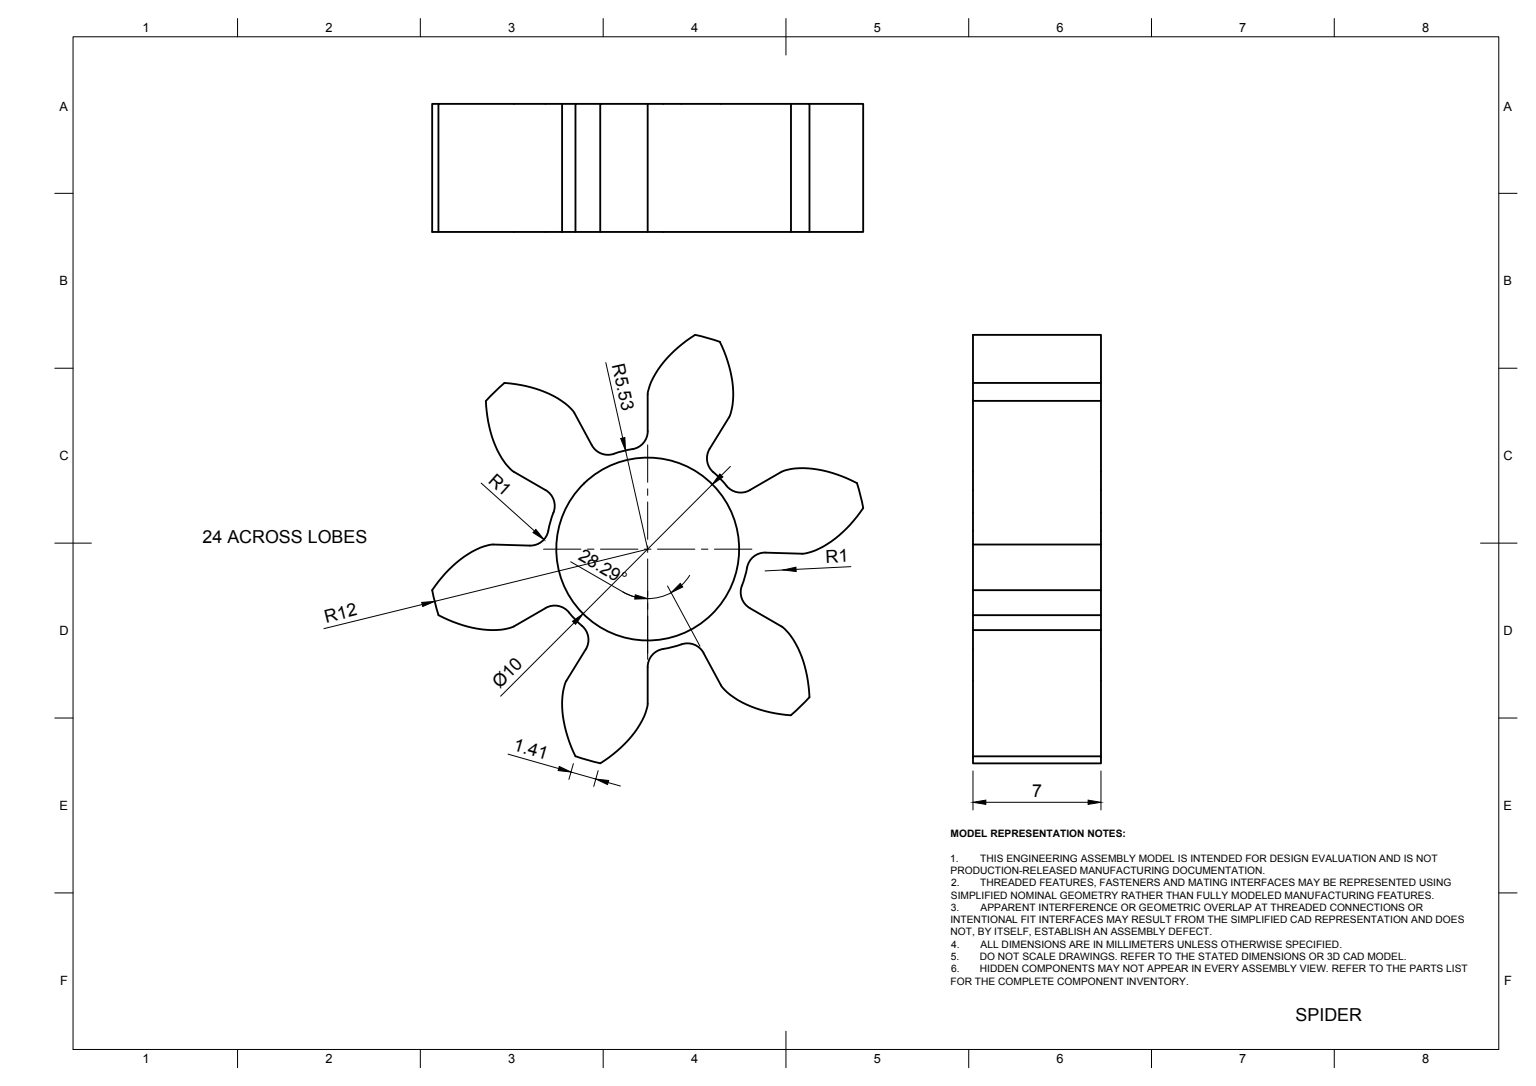
ISO-10303-21;
HEADER;
/* Generated by software containing ST-Developer
 * from STEP Tools, Inc. (www.steptools.com) 
 */

FILE_DESCRIPTION(
/* description */ (''),
/* implementation_level */ '2;1');

FILE_NAME(
/* name */ 'Spider.step',
/* time_stamp */ '2026-10-05T21:34:53-07:00',
/* author */ (''),
/* organization */ (''),
/* preprocessor_version */ 'ST-DEVELOPER v20.2',
/* originating_system */ 'Autodesk Translation Framework v15.15.0.0',
/* authorisation */ '');

FILE_SCHEMA (('AUTOMOTIVE_DESIGN { 1 0 10303 214 3 1 1 }'));
ENDSEC;

DATA;
#10=MECHANICAL_DESIGN_GEOMETRIC_PRESENTATION_REPRESENTATION('',(#65),#9822);
#47=SHAPE_REPRESENTATION_RELATIONSHIP('SRR','None',#9857,#56);
#56=ADVANCED_BREP_SHAPE_REPRESENTATION('',(#74),#9813);
#65=STYLED_ITEM('',(#9911),#74);
#74=MANIFOLD_SOLID_BREP('Body1',#3288);
#83=FACE_BOUND('',#486,.T.);
#84=FACE_BOUND('',#500,.T.);
#99=B_SPLINE_CURVE_WITH_KNOTS('',5,(#4949,#4950,#4951,#4952,#4953,#4954,
#4955,#4956,#4957,#4958,#4959,#4960,#4961,#4962,#4963,#4964,#4965,#4966,
#4967,#4968,#4969,#4970,#4971,#4972,#4973,#4974,#4975,#4976,#4977,#4978,
#4979,#4980,#4981,#4982,#4983,#4984,#4985,#4986,#4987,#4988,#4989,#4990,
#4991,#4992,#4993,#4994,#4995,#4996,#4997,#4998,#4999,#5000,#5001,#5002,
#5003,#5004,#5005,#5006,#5007,#5008,#5009,#5010,#5011,#5012,#5013,#5014,
#5015,#5016,#5017,#5018,#5019,#5020,#5021,#5022,#5023),.UNSPECIFIED.,.F.,
 .F.,(6,1,1,1,1,1,1,1,1,1,1,1,1,1,1,1,1,1,1,1,1,1,1,1,1,1,1,1,1,1,1,1,1,
1,1,1,1,1,1,1,1,1,1,1,1,1,1,1,1,1,1,1,1,1,1,1,1,1,1,1,1,1,1,1,1,1,1,1,1,
1,6),(-1.,-0.985714285714284,-0.97142857142857,-0.957142857142856,-0.942857142857141,
-0.928571428571427,-0.914285714285713,-0.899999999999999,-0.885714285714284,
-0.87142857142857,-0.857142857142856,-0.842857142857142,-0.828571428571428,
-0.814285714285713,-0.799999999999999,-0.785714285714285,-0.771428571428571,
-0.757142857142856,-0.742857142857142,-0.728571428571428,-0.714285714285714,
-0.699999999999999,-0.685714285714285,-0.671428571428571,-0.657142857142857,
-0.642857142857142,-0.628571428571428,-0.614285714285714,-0.6,-0.585714285714286,
-0.571428571428571,-0.557142857142857,-0.542857142857143,-0.528571428571429,
-0.514285714285714,-0.5,-0.485714285714286,-0.471428571428572,-0.457142857142857,
-0.442857142857143,-0.428571428571429,-0.414285714285714,-0.4,-0.385714285714286,
-0.371428571428571,-0.357142857142857,-0.342857142857143,-0.328571428571429,
-0.314285714285714,-0.3,-0.285714285714286,-0.271428571428571,-0.257142857142857,
-0.242857142857143,-0.228571428571429,-0.214285714285714,-0.2,-0.185714285714286,
-0.171428571428571,-0.157142857142857,-0.142857142857143,-0.128571428571429,
-0.114285714285714,-0.1,-0.0857142857142857,-0.0714285714285714,-0.0571428571428571,
-0.0428571428571429,-0.0285714285714286,-0.0142857142857143,0.),
 .UNSPECIFIED.);
#100=B_SPLINE_CURVE_WITH_KNOTS('',5,(#5025,#5026,#5027,#5028,#5029,#5030,
#5031,#5032,#5033,#5034,#5035,#5036,#5037,#5038,#5039,#5040,#5041,#5042,
#5043,#5044,#5045,#5046,#5047,#5048,#5049,#5050,#5051,#5052,#5053,#5054,
#5055,#5056,#5057,#5058,#5059,#5060,#5061,#5062,#5063,#5064,#5065,#5066,
#5067,#5068,#5069,#5070,#5071,#5072,#5073,#5074,#5075,#5076,#5077,#5078,
#5079,#5080,#5081,#5082,#5083,#5084,#5085,#5086,#5087,#5088,#5089,#5090,
#5091,#5092,#5093,#5094,#5095,#5096,#5097,#5098,#5099),.UNSPECIFIED.,.F.,
 .F.,(6,1,1,1,1,1,1,1,1,1,1,1,1,1,1,1,1,1,1,1,1,1,1,1,1,1,1,1,1,1,1,1,1,
1,1,1,1,1,1,1,1,1,1,1,1,1,1,1,1,1,1,1,1,1,1,1,1,1,1,1,1,1,1,1,1,1,1,1,1,
1,6),(-1.,-0.985714285714284,-0.97142857142857,-0.957142857142856,-0.942857142857141,
-0.928571428571427,-0.914285714285713,-0.899999999999999,-0.885714285714284,
-0.87142857142857,-0.857142857142856,-0.842857142857142,-0.828571428571428,
-0.814285714285713,-0.799999999999999,-0.785714285714285,-0.771428571428571,
-0.757142857142856,-0.742857142857142,-0.728571428571428,-0.714285714285714,
-0.699999999999999,-0.685714285714285,-0.671428571428571,-0.657142857142857,
-0.642857142857142,-0.628571428571428,-0.614285714285714,-0.6,-0.585714285714286,
-0.571428571428571,-0.557142857142857,-0.542857142857143,-0.528571428571429,
-0.514285714285714,-0.5,-0.485714285714286,-0.471428571428572,-0.457142857142857,
-0.442857142857143,-0.428571428571429,-0.414285714285714,-0.4,-0.385714285714286,
-0.371428571428571,-0.357142857142857,-0.342857142857143,-0.328571428571429,
-0.314285714285714,-0.3,-0.285714285714286,-0.271428571428571,-0.257142857142857,
-0.242857142857143,-0.228571428571429,-0.214285714285714,-0.2,-0.185714285714286,
-0.171428571428571,-0.157142857142857,-0.142857142857143,-0.128571428571429,
-0.114285714285714,-0.1,-0.0857142857142857,-0.0714285714285714,-0.0571428571428571,
-0.0428571428571429,-0.0285714285714286,-0.0142857142857143,0.),
 .UNSPECIFIED.);
#101=B_SPLINE_CURVE_WITH_KNOTS('',5,(#5257,#5258,#5259,#5260,#5261,#5262,
#5263,#5264,#5265,#5266,#5267,#5268,#5269,#5270,#5271,#5272,#5273,#5274,
#5275,#5276,#5277,#5278,#5279,#5280,#5281,#5282,#5283,#5284,#5285,#5286,
#5287,#5288,#5289,#5290,#5291,#5292,#5293,#5294,#5295,#5296,#5297,#5298,
#5299,#5300,#5301,#5302,#5303,#5304,#5305,#5306,#5307,#5308,#5309,#5310,
#5311,#5312,#5313,#5314,#5315,#5316,#5317,#5318,#5319,#5320,#5321,#5322,
#5323,#5324,#5325,#5326,#5327,#5328,#5329,#5330,#5331),.UNSPECIFIED.,.F.,
 .F.,(6,1,1,1,1,1,1,1,1,1,1,1,1,1,1,1,1,1,1,1,1,1,1,1,1,1,1,1,1,1,1,1,1,
1,1,1,1,1,1,1,1,1,1,1,1,1,1,1,1,1,1,1,1,1,1,1,1,1,1,1,1,1,1,1,1,1,1,1,1,
1,6),(0.,0.0142857142857143,0.0285714285714286,0.0428571428571429,0.0571428571428571,
0.0714285714285714,0.0857142857142857,0.1,0.114285714285714,0.128571428571429,
0.142857142857143,0.157142857142857,0.171428571428571,0.185714285714286,
0.2,0.214285714285714,0.228571428571429,0.242857142857143,0.257142857142857,
0.271428571428571,0.285714285714286,0.3,0.314285714285714,0.328571428571429,
0.342857142857143,0.357142857142857,0.371428571428571,0.385714285714286,
0.4,0.414285714285714,0.428571428571429,0.442857142857143,0.457142857142857,
0.471428571428572,0.485714285714286,0.5,0.514285714285714,0.528571428571429,
0.542857142857143,0.557142857142857,0.571428571428571,0.585714285714286,
0.6,0.614285714285714,0.628571428571428,0.642857142857142,0.657142857142857,
0.671428571428571,0.685714285714285,0.699999999999999,0.714285714285714,
0.728571428571428,0.742857142857142,0.757142857142856,0.771428571428571,
0.785714285714285,0.799999999999999,0.814285714285713,0.828571428571428,
0.842857142857142,0.857142857142856,0.87142857142857,0.885714285714284,
0.899999999999999,0.914285714285713,0.928571428571427,0.942857142857141,
0.957142857142856,0.97142857142857,0.985714285714284,1.),.UNSPECIFIED.);
#102=B_SPLINE_CURVE_WITH_KNOTS('',5,(#5332,#5333,#5334,#5335,#5336,#5337,
#5338,#5339,#5340,#5341,#5342,#5343,#5344,#5345,#5346,#5347,#5348,#5349,
#5350,#5351,#5352,#5353,#5354,#5355,#5356,#5357,#5358,#5359,#5360,#5361,
#5362,#5363,#5364,#5365,#5366,#5367,#5368,#5369,#5370,#5371,#5372,#5373,
#5374,#5375,#5376,#5377,#5378,#5379,#5380,#5381,#5382,#5383,#5384,#5385,
#5386,#5387,#5388,#5389,#5390,#5391,#5392,#5393,#5394,#5395,#5396,#5397,
#5398,#5399,#5400,#5401,#5402,#5403,#5404,#5405,#5406),.UNSPECIFIED.,.F.,
 .F.,(6,1,1,1,1,1,1,1,1,1,1,1,1,1,1,1,1,1,1,1,1,1,1,1,1,1,1,1,1,1,1,1,1,
1,1,1,1,1,1,1,1,1,1,1,1,1,1,1,1,1,1,1,1,1,1,1,1,1,1,1,1,1,1,1,1,1,1,1,1,
1,6),(0.,0.0142857142857143,0.0285714285714286,0.0428571428571429,0.0571428571428571,
0.0714285714285714,0.0857142857142857,0.1,0.114285714285714,0.128571428571429,
0.142857142857143,0.157142857142857,0.171428571428571,0.185714285714286,
0.2,0.214285714285714,0.228571428571429,0.242857142857143,0.257142857142857,
0.271428571428571,0.285714285714286,0.3,0.314285714285714,0.328571428571429,
0.342857142857143,0.357142857142857,0.371428571428571,0.385714285714286,
0.4,0.414285714285714,0.428571428571429,0.442857142857143,0.457142857142857,
0.471428571428572,0.485714285714286,0.5,0.514285714285714,0.528571428571429,
0.542857142857143,0.557142857142857,0.571428571428571,0.585714285714286,
0.6,0.614285714285714,0.628571428571428,0.642857142857142,0.657142857142857,
0.671428571428571,0.685714285714285,0.699999999999999,0.714285714285714,
0.728571428571428,0.742857142857142,0.757142857142856,0.771428571428571,
0.785714285714285,0.799999999999999,0.814285714285713,0.828571428571428,
0.842857142857142,0.857142857142856,0.87142857142857,0.885714285714284,
0.899999999999999,0.914285714285713,0.928571428571427,0.942857142857141,
0.957142857142856,0.97142857142857,0.985714285714284,1.),.UNSPECIFIED.);
#103=B_SPLINE_CURVE_WITH_KNOTS('',5,(#5558,#5559,#5560,#5561,#5562,#5563,
#5564,#5565,#5566,#5567,#5568,#5569,#5570,#5571,#5572,#5573,#5574,#5575,
#5576,#5577,#5578,#5579,#5580,#5581,#5582,#5583,#5584,#5585,#5586,#5587,
#5588,#5589,#5590,#5591,#5592,#5593,#5594,#5595,#5596,#5597,#5598,#5599,
#5600,#5601,#5602,#5603,#5604,#5605,#5606,#5607,#5608,#5609,#5610,#5611,
#5612,#5613,#5614,#5615,#5616,#5617,#5618,#5619,#5620,#5621,#5622,#5623,
#5624,#5625,#5626,#5627,#5628,#5629,#5630,#5631,#5632),.UNSPECIFIED.,.F.,
 .F.,(6,1,1,1,1,1,1,1,1,1,1,1,1,1,1,1,1,1,1,1,1,1,1,1,1,1,1,1,1,1,1,1,1,
1,1,1,1,1,1,1,1,1,1,1,1,1,1,1,1,1,1,1,1,1,1,1,1,1,1,1,1,1,1,1,1,1,1,1,1,
1,6),(-1.,-0.985714285714284,-0.97142857142857,-0.957142857142856,-0.942857142857141,
-0.928571428571427,-0.914285714285713,-0.899999999999999,-0.885714285714284,
-0.87142857142857,-0.857142857142856,-0.842857142857142,-0.828571428571428,
-0.814285714285713,-0.799999999999999,-0.785714285714285,-0.771428571428571,
-0.757142857142856,-0.742857142857142,-0.728571428571428,-0.714285714285714,
-0.699999999999999,-0.685714285714285,-0.671428571428571,-0.657142857142857,
-0.642857142857142,-0.628571428571428,-0.614285714285714,-0.6,-0.585714285714286,
-0.571428571428571,-0.557142857142857,-0.542857142857143,-0.528571428571429,
-0.514285714285714,-0.5,-0.485714285714286,-0.471428571428572,-0.457142857142857,
-0.442857142857143,-0.428571428571429,-0.414285714285714,-0.4,-0.385714285714286,
-0.371428571428571,-0.357142857142857,-0.342857142857143,-0.328571428571429,
-0.314285714285714,-0.3,-0.285714285714286,-0.271428571428571,-0.257142857142857,
-0.242857142857143,-0.228571428571429,-0.214285714285714,-0.2,-0.185714285714286,
-0.171428571428571,-0.157142857142857,-0.142857142857143,-0.128571428571429,
-0.114285714285714,-0.1,-0.0857142857142857,-0.0714285714285714,-0.0571428571428571,
-0.0428571428571429,-0.0285714285714286,-0.0142857142857143,0.),
 .UNSPECIFIED.);
#104=B_SPLINE_CURVE_WITH_KNOTS('',5,(#5634,#5635,#5636,#5637,#5638,#5639,
#5640,#5641,#5642,#5643,#5644,#5645,#5646,#5647,#5648,#5649,#5650,#5651,
#5652,#5653,#5654,#5655,#5656,#5657,#5658,#5659,#5660,#5661,#5662,#5663,
#5664,#5665,#5666,#5667,#5668,#5669,#5670,#5671,#5672,#5673,#5674,#5675,
#5676,#5677,#5678,#5679,#5680,#5681,#5682,#5683,#5684,#5685,#5686,#5687,
#5688,#5689,#5690,#5691,#5692,#5693,#5694,#5695,#5696,#5697,#5698,#5699,
#5700,#5701,#5702,#5703,#5704,#5705,#5706,#5707,#5708),.UNSPECIFIED.,.F.,
 .F.,(6,1,1,1,1,1,1,1,1,1,1,1,1,1,1,1,1,1,1,1,1,1,1,1,1,1,1,1,1,1,1,1,1,
1,1,1,1,1,1,1,1,1,1,1,1,1,1,1,1,1,1,1,1,1,1,1,1,1,1,1,1,1,1,1,1,1,1,1,1,
1,6),(-1.,-0.985714285714284,-0.97142857142857,-0.957142857142856,-0.942857142857141,
-0.928571428571427,-0.914285714285713,-0.899999999999999,-0.885714285714284,
-0.87142857142857,-0.857142857142856,-0.842857142857142,-0.828571428571428,
-0.814285714285713,-0.799999999999999,-0.785714285714285,-0.771428571428571,
-0.757142857142856,-0.742857142857142,-0.728571428571428,-0.714285714285714,
-0.699999999999999,-0.685714285714285,-0.671428571428571,-0.657142857142857,
-0.642857142857142,-0.628571428571428,-0.614285714285714,-0.6,-0.585714285714286,
-0.571428571428571,-0.557142857142857,-0.542857142857143,-0.528571428571429,
-0.514285714285714,-0.5,-0.485714285714286,-0.471428571428572,-0.457142857142857,
-0.442857142857143,-0.428571428571429,-0.414285714285714,-0.4,-0.385714285714286,
-0.371428571428571,-0.357142857142857,-0.342857142857143,-0.328571428571429,
-0.314285714285714,-0.3,-0.285714285714286,-0.271428571428571,-0.257142857142857,
-0.242857142857143,-0.228571428571429,-0.214285714285714,-0.2,-0.185714285714286,
-0.171428571428571,-0.157142857142857,-0.142857142857143,-0.128571428571429,
-0.114285714285714,-0.1,-0.0857142857142857,-0.0714285714285714,-0.0571428571428571,
-0.0428571428571429,-0.0285714285714286,-0.0142857142857143,0.),
 .UNSPECIFIED.);
#105=B_SPLINE_CURVE_WITH_KNOTS('',5,(#5866,#5867,#5868,#5869,#5870,#5871,
#5872,#5873,#5874,#5875,#5876,#5877,#5878,#5879,#5880,#5881,#5882,#5883,
#5884,#5885,#5886,#5887,#5888,#5889,#5890,#5891,#5892,#5893,#5894,#5895,
#5896,#5897,#5898,#5899,#5900,#5901,#5902,#5903,#5904,#5905,#5906,#5907,
#5908,#5909,#5910,#5911,#5912,#5913,#5914,#5915,#5916,#5917,#5918,#5919,
#5920,#5921,#5922,#5923,#5924,#5925,#5926,#5927,#5928,#5929,#5930,#5931,
#5932,#5933,#5934,#5935,#5936,#5937,#5938,#5939,#5940),.UNSPECIFIED.,.F.,
 .F.,(6,1,1,1,1,1,1,1,1,1,1,1,1,1,1,1,1,1,1,1,1,1,1,1,1,1,1,1,1,1,1,1,1,
1,1,1,1,1,1,1,1,1,1,1,1,1,1,1,1,1,1,1,1,1,1,1,1,1,1,1,1,1,1,1,1,1,1,1,1,
1,6),(0.,0.0142857142857143,0.0285714285714286,0.0428571428571429,0.0571428571428571,
0.0714285714285714,0.0857142857142857,0.1,0.114285714285714,0.128571428571429,
0.142857142857143,0.157142857142857,0.171428571428571,0.185714285714286,
0.2,0.214285714285714,0.228571428571429,0.242857142857143,0.257142857142857,
0.271428571428571,0.285714285714286,0.3,0.314285714285714,0.328571428571429,
0.342857142857143,0.357142857142857,0.371428571428571,0.385714285714286,
0.4,0.414285714285714,0.428571428571429,0.442857142857143,0.457142857142857,
0.471428571428572,0.485714285714286,0.5,0.514285714285714,0.528571428571429,
0.542857142857143,0.557142857142857,0.571428571428571,0.585714285714286,
0.6,0.614285714285714,0.628571428571428,0.642857142857142,0.657142857142857,
0.671428571428571,0.685714285714285,0.699999999999999,0.714285714285714,
0.728571428571428,0.742857142857142,0.757142857142856,0.771428571428571,
0.785714285714285,0.799999999999999,0.814285714285713,0.828571428571428,
0.842857142857142,0.857142857142856,0.87142857142857,0.885714285714284,
0.899999999999999,0.914285714285713,0.928571428571427,0.942857142857141,
0.957142857142856,0.97142857142857,0.985714285714284,1.),.UNSPECIFIED.);
#106=B_SPLINE_CURVE_WITH_KNOTS('',5,(#5941,#5942,#5943,#5944,#5945,#5946,
#5947,#5948,#5949,#5950,#5951,#5952,#5953,#5954,#5955,#5956,#5957,#5958,
#5959,#5960,#5961,#5962,#5963,#5964,#5965,#5966,#5967,#5968,#5969,#5970,
#5971,#5972,#5973,#5974,#5975,#5976,#5977,#5978,#5979,#5980,#5981,#5982,
#5983,#5984,#5985,#5986,#5987,#5988,#5989,#5990,#5991,#5992,#5993,#5994,
#5995,#5996,#5997,#5998,#5999,#6000,#6001,#6002,#6003,#6004,#6005,#6006,
#6007,#6008,#6009,#6010,#6011,#6012,#6013,#6014,#6015),.UNSPECIFIED.,.F.,
 .F.,(6,1,1,1,1,1,1,1,1,1,1,1,1,1,1,1,1,1,1,1,1,1,1,1,1,1,1,1,1,1,1,1,1,
1,1,1,1,1,1,1,1,1,1,1,1,1,1,1,1,1,1,1,1,1,1,1,1,1,1,1,1,1,1,1,1,1,1,1,1,
1,6),(0.,0.0142857142857143,0.0285714285714286,0.0428571428571429,0.0571428571428571,
0.0714285714285714,0.0857142857142857,0.1,0.114285714285714,0.128571428571429,
0.142857142857143,0.157142857142857,0.171428571428571,0.185714285714286,
0.2,0.214285714285714,0.228571428571429,0.242857142857143,0.257142857142857,
0.271428571428571,0.285714285714286,0.3,0.314285714285714,0.328571428571429,
0.342857142857143,0.357142857142857,0.371428571428571,0.385714285714286,
0.4,0.414285714285714,0.428571428571429,0.442857142857143,0.457142857142857,
0.471428571428572,0.485714285714286,0.5,0.514285714285714,0.528571428571429,
0.542857142857143,0.557142857142857,0.571428571428571,0.585714285714286,
0.6,0.614285714285714,0.628571428571428,0.642857142857142,0.657142857142857,
0.671428571428571,0.685714285714285,0.699999999999999,0.714285714285714,
0.728571428571428,0.742857142857142,0.757142857142856,0.771428571428571,
0.785714285714285,0.799999999999999,0.814285714285713,0.828571428571428,
0.842857142857142,0.857142857142856,0.87142857142857,0.885714285714284,
0.899999999999999,0.914285714285713,0.928571428571427,0.942857142857141,
0.957142857142856,0.97142857142857,0.985714285714284,1.),.UNSPECIFIED.);
#107=B_SPLINE_CURVE_WITH_KNOTS('',5,(#6167,#6168,#6169,#6170,#6171,#6172,
#6173,#6174,#6175,#6176,#6177,#6178,#6179,#6180,#6181,#6182,#6183,#6184,
#6185,#6186,#6187,#6188,#6189,#6190,#6191,#6192,#6193,#6194,#6195,#6196,
#6197,#6198,#6199,#6200,#6201,#6202,#6203,#6204,#6205,#6206,#6207,#6208,
#6209,#6210,#6211,#6212,#6213,#6214,#6215,#6216,#6217,#6218,#6219,#6220,
#6221,#6222,#6223,#6224,#6225,#6226,#6227,#6228,#6229,#6230,#6231,#6232,
#6233,#6234,#6235,#6236,#6237,#6238,#6239,#6240,#6241),.UNSPECIFIED.,.F.,
 .F.,(6,1,1,1,1,1,1,1,1,1,1,1,1,1,1,1,1,1,1,1,1,1,1,1,1,1,1,1,1,1,1,1,1,
1,1,1,1,1,1,1,1,1,1,1,1,1,1,1,1,1,1,1,1,1,1,1,1,1,1,1,1,1,1,1,1,1,1,1,1,
1,6),(-1.,-0.985714285714284,-0.97142857142857,-0.957142857142856,-0.942857142857141,
-0.928571428571427,-0.914285714285713,-0.899999999999999,-0.885714285714284,
-0.87142857142857,-0.857142857142856,-0.842857142857142,-0.828571428571428,
-0.814285714285713,-0.799999999999999,-0.785714285714285,-0.771428571428571,
-0.757142857142856,-0.742857142857142,-0.728571428571428,-0.714285714285714,
-0.699999999999999,-0.685714285714285,-0.671428571428571,-0.657142857142857,
-0.642857142857142,-0.628571428571428,-0.614285714285714,-0.6,-0.585714285714286,
-0.571428571428571,-0.557142857142857,-0.542857142857143,-0.528571428571429,
-0.514285714285714,-0.5,-0.485714285714286,-0.471428571428572,-0.457142857142857,
-0.442857142857143,-0.428571428571429,-0.414285714285714,-0.4,-0.385714285714286,
-0.371428571428571,-0.357142857142857,-0.342857142857143,-0.328571428571429,
-0.314285714285714,-0.3,-0.285714285714286,-0.271428571428571,-0.257142857142857,
-0.242857142857143,-0.228571428571429,-0.214285714285714,-0.2,-0.185714285714286,
-0.171428571428571,-0.157142857142857,-0.142857142857143,-0.128571428571429,
-0.114285714285714,-0.1,-0.0857142857142857,-0.0714285714285714,-0.0571428571428571,
-0.0428571428571429,-0.0285714285714286,-0.0142857142857143,0.),
 .UNSPECIFIED.);
#108=B_SPLINE_CURVE_WITH_KNOTS('',5,(#6243,#6244,#6245,#6246,#6247,#6248,
#6249,#6250,#6251,#6252,#6253,#6254,#6255,#6256,#6257,#6258,#6259,#6260,
#6261,#6262,#6263,#6264,#6265,#6266,#6267,#6268,#6269,#6270,#6271,#6272,
#6273,#6274,#6275,#6276,#6277,#6278,#6279,#6280,#6281,#6282,#6283,#6284,
#6285,#6286,#6287,#6288,#6289,#6290,#6291,#6292,#6293,#6294,#6295,#6296,
#6297,#6298,#6299,#6300,#6301,#6302,#6303,#6304,#6305,#6306,#6307,#6308,
#6309,#6310,#6311,#6312,#6313,#6314,#6315,#6316,#6317),.UNSPECIFIED.,.F.,
 .F.,(6,1,1,1,1,1,1,1,1,1,1,1,1,1,1,1,1,1,1,1,1,1,1,1,1,1,1,1,1,1,1,1,1,
1,1,1,1,1,1,1,1,1,1,1,1,1,1,1,1,1,1,1,1,1,1,1,1,1,1,1,1,1,1,1,1,1,1,1,1,
1,6),(-1.,-0.985714285714284,-0.97142857142857,-0.957142857142856,-0.942857142857141,
-0.928571428571427,-0.914285714285713,-0.899999999999999,-0.885714285714284,
-0.87142857142857,-0.857142857142856,-0.842857142857142,-0.828571428571428,
-0.814285714285713,-0.799999999999999,-0.785714285714285,-0.771428571428571,
-0.757142857142856,-0.742857142857142,-0.728571428571428,-0.714285714285714,
-0.699999999999999,-0.685714285714285,-0.671428571428571,-0.657142857142857,
-0.642857142857142,-0.628571428571428,-0.614285714285714,-0.6,-0.585714285714286,
-0.571428571428571,-0.557142857142857,-0.542857142857143,-0.528571428571429,
-0.514285714285714,-0.5,-0.485714285714286,-0.471428571428572,-0.457142857142857,
-0.442857142857143,-0.428571428571429,-0.414285714285714,-0.4,-0.385714285714286,
-0.371428571428571,-0.357142857142857,-0.342857142857143,-0.328571428571429,
-0.314285714285714,-0.3,-0.285714285714286,-0.271428571428571,-0.257142857142857,
-0.242857142857143,-0.228571428571429,-0.214285714285714,-0.2,-0.185714285714286,
-0.171428571428571,-0.157142857142857,-0.142857142857143,-0.128571428571429,
-0.114285714285714,-0.1,-0.0857142857142857,-0.0714285714285714,-0.0571428571428571,
-0.0428571428571429,-0.0285714285714286,-0.0142857142857143,0.),
 .UNSPECIFIED.);
#109=B_SPLINE_CURVE_WITH_KNOTS('',5,(#6475,#6476,#6477,#6478,#6479,#6480,
#6481,#6482,#6483,#6484,#6485,#6486,#6487,#6488,#6489,#6490,#6491,#6492,
#6493,#6494,#6495,#6496,#6497,#6498,#6499,#6500,#6501,#6502,#6503,#6504,
#6505,#6506,#6507,#6508,#6509,#6510,#6511,#6512,#6513,#6514,#6515,#6516,
#6517,#6518,#6519,#6520,#6521,#6522,#6523,#6524,#6525,#6526,#6527,#6528,
#6529,#6530,#6531,#6532,#6533,#6534,#6535,#6536,#6537,#6538,#6539,#6540,
#6541,#6542,#6543,#6544,#6545,#6546,#6547,#6548,#6549),.UNSPECIFIED.,.F.,
 .F.,(6,1,1,1,1,1,1,1,1,1,1,1,1,1,1,1,1,1,1,1,1,1,1,1,1,1,1,1,1,1,1,1,1,
1,1,1,1,1,1,1,1,1,1,1,1,1,1,1,1,1,1,1,1,1,1,1,1,1,1,1,1,1,1,1,1,1,1,1,1,
1,6),(0.,0.0142857142857143,0.0285714285714286,0.0428571428571429,0.0571428571428571,
0.0714285714285714,0.0857142857142857,0.1,0.114285714285714,0.128571428571429,
0.142857142857143,0.157142857142857,0.171428571428571,0.185714285714286,
0.2,0.214285714285714,0.228571428571429,0.242857142857143,0.257142857142857,
0.271428571428571,0.285714285714286,0.3,0.314285714285714,0.328571428571429,
0.342857142857143,0.357142857142857,0.371428571428571,0.385714285714286,
0.4,0.414285714285714,0.428571428571429,0.442857142857143,0.457142857142857,
0.471428571428572,0.485714285714286,0.5,0.514285714285714,0.528571428571429,
0.542857142857143,0.557142857142857,0.571428571428571,0.585714285714286,
0.6,0.614285714285714,0.628571428571428,0.642857142857142,0.657142857142857,
0.671428571428571,0.685714285714285,0.699999999999999,0.714285714285714,
0.728571428571428,0.742857142857142,0.757142857142856,0.771428571428571,
0.785714285714285,0.799999999999999,0.814285714285713,0.828571428571428,
0.842857142857142,0.857142857142856,0.87142857142857,0.885714285714284,
0.899999999999999,0.914285714285713,0.928571428571427,0.942857142857141,
0.957142857142856,0.97142857142857,0.985714285714284,1.),.UNSPECIFIED.);
#110=B_SPLINE_CURVE_WITH_KNOTS('',5,(#6550,#6551,#6552,#6553,#6554,#6555,
#6556,#6557,#6558,#6559,#6560,#6561,#6562,#6563,#6564,#6565,#6566,#6567,
#6568,#6569,#6570,#6571,#6572,#6573,#6574,#6575,#6576,#6577,#6578,#6579,
#6580,#6581,#6582,#6583,#6584,#6585,#6586,#6587,#6588,#6589,#6590,#6591,
#6592,#6593,#6594,#6595,#6596,#6597,#6598,#6599,#6600,#6601,#6602,#6603,
#6604,#6605,#6606,#6607,#6608,#6609,#6610,#6611,#6612,#6613,#6614,#6615,
#6616,#6617,#6618,#6619,#6620,#6621,#6622,#6623,#6624),.UNSPECIFIED.,.F.,
 .F.,(6,1,1,1,1,1,1,1,1,1,1,1,1,1,1,1,1,1,1,1,1,1,1,1,1,1,1,1,1,1,1,1,1,
1,1,1,1,1,1,1,1,1,1,1,1,1,1,1,1,1,1,1,1,1,1,1,1,1,1,1,1,1,1,1,1,1,1,1,1,
1,6),(0.,0.0142857142857143,0.0285714285714286,0.0428571428571429,0.0571428571428571,
0.0714285714285714,0.0857142857142857,0.1,0.114285714285714,0.128571428571429,
0.142857142857143,0.157142857142857,0.171428571428571,0.185714285714286,
0.2,0.214285714285714,0.228571428571429,0.242857142857143,0.257142857142857,
0.271428571428571,0.285714285714286,0.3,0.314285714285714,0.328571428571429,
0.342857142857143,0.357142857142857,0.371428571428571,0.385714285714286,
0.4,0.414285714285714,0.428571428571429,0.442857142857143,0.457142857142857,
0.471428571428572,0.485714285714286,0.5,0.514285714285714,0.528571428571429,
0.542857142857143,0.557142857142857,0.571428571428571,0.585714285714286,
0.6,0.614285714285714,0.628571428571428,0.642857142857142,0.657142857142857,
0.671428571428571,0.685714285714285,0.699999999999999,0.714285714285714,
0.728571428571428,0.742857142857142,0.757142857142856,0.771428571428571,
0.785714285714285,0.799999999999999,0.814285714285713,0.828571428571428,
0.842857142857142,0.857142857142856,0.87142857142857,0.885714285714284,
0.899999999999999,0.914285714285713,0.928571428571427,0.942857142857141,
0.957142857142856,0.97142857142857,0.985714285714284,1.),.UNSPECIFIED.);
#111=B_SPLINE_CURVE_WITH_KNOTS('',5,(#6776,#6777,#6778,#6779,#6780,#6781,
#6782,#6783,#6784,#6785,#6786,#6787,#6788,#6789,#6790,#6791,#6792,#6793,
#6794,#6795,#6796,#6797,#6798,#6799,#6800,#6801,#6802,#6803,#6804,#6805,
#6806,#6807,#6808,#6809,#6810,#6811,#6812,#6813,#6814,#6815,#6816,#6817,
#6818,#6819,#6820,#6821,#6822,#6823,#6824,#6825,#6826,#6827,#6828,#6829,
#6830,#6831,#6832,#6833,#6834,#6835,#6836,#6837,#6838,#6839,#6840,#6841,
#6842,#6843,#6844,#6845,#6846,#6847,#6848,#6849,#6850),.UNSPECIFIED.,.F.,
 .F.,(6,1,1,1,1,1,1,1,1,1,1,1,1,1,1,1,1,1,1,1,1,1,1,1,1,1,1,1,1,1,1,1,1,
1,1,1,1,1,1,1,1,1,1,1,1,1,1,1,1,1,1,1,1,1,1,1,1,1,1,1,1,1,1,1,1,1,1,1,1,
1,6),(-1.,-0.985714285714284,-0.97142857142857,-0.957142857142856,-0.942857142857141,
-0.928571428571427,-0.914285714285713,-0.899999999999999,-0.885714285714284,
-0.87142857142857,-0.857142857142856,-0.842857142857142,-0.828571428571428,
-0.814285714285713,-0.799999999999999,-0.785714285714285,-0.771428571428571,
-0.757142857142856,-0.742857142857142,-0.728571428571428,-0.714285714285714,
-0.699999999999999,-0.685714285714285,-0.671428571428571,-0.657142857142857,
-0.642857142857142,-0.628571428571428,-0.614285714285714,-0.6,-0.585714285714286,
-0.571428571428571,-0.557142857142857,-0.542857142857143,-0.528571428571429,
-0.514285714285714,-0.5,-0.485714285714286,-0.471428571428572,-0.457142857142857,
-0.442857142857143,-0.428571428571429,-0.414285714285714,-0.4,-0.385714285714286,
-0.371428571428571,-0.357142857142857,-0.342857142857143,-0.328571428571429,
-0.314285714285714,-0.3,-0.285714285714286,-0.271428571428571,-0.257142857142857,
-0.242857142857143,-0.228571428571429,-0.214285714285714,-0.2,-0.185714285714286,
-0.171428571428571,-0.157142857142857,-0.142857142857143,-0.128571428571429,
-0.114285714285714,-0.1,-0.0857142857142857,-0.0714285714285714,-0.0571428571428571,
-0.0428571428571429,-0.0285714285714286,-0.0142857142857143,0.),
 .UNSPECIFIED.);
#112=B_SPLINE_CURVE_WITH_KNOTS('',5,(#6852,#6853,#6854,#6855,#6856,#6857,
#6858,#6859,#6860,#6861,#6862,#6863,#6864,#6865,#6866,#6867,#6868,#6869,
#6870,#6871,#6872,#6873,#6874,#6875,#6876,#6877,#6878,#6879,#6880,#6881,
#6882,#6883,#6884,#6885,#6886,#6887,#6888,#6889,#6890,#6891,#6892,#6893,
#6894,#6895,#6896,#6897,#6898,#6899,#6900,#6901,#6902,#6903,#6904,#6905,
#6906,#6907,#6908,#6909,#6910,#6911,#6912,#6913,#6914,#6915,#6916,#6917,
#6918,#6919,#6920,#6921,#6922,#6923,#6924,#6925,#6926),.UNSPECIFIED.,.F.,
 .F.,(6,1,1,1,1,1,1,1,1,1,1,1,1,1,1,1,1,1,1,1,1,1,1,1,1,1,1,1,1,1,1,1,1,
1,1,1,1,1,1,1,1,1,1,1,1,1,1,1,1,1,1,1,1,1,1,1,1,1,1,1,1,1,1,1,1,1,1,1,1,
1,6),(-1.,-0.985714285714284,-0.97142857142857,-0.957142857142856,-0.942857142857141,
-0.928571428571427,-0.914285714285713,-0.899999999999999,-0.885714285714284,
-0.87142857142857,-0.857142857142856,-0.842857142857142,-0.828571428571428,
-0.814285714285713,-0.799999999999999,-0.785714285714285,-0.771428571428571,
-0.757142857142856,-0.742857142857142,-0.728571428571428,-0.714285714285714,
-0.699999999999999,-0.685714285714285,-0.671428571428571,-0.657142857142857,
-0.642857142857142,-0.628571428571428,-0.614285714285714,-0.6,-0.585714285714286,
-0.571428571428571,-0.557142857142857,-0.542857142857143,-0.528571428571429,
-0.514285714285714,-0.5,-0.485714285714286,-0.471428571428572,-0.457142857142857,
-0.442857142857143,-0.428571428571429,-0.414285714285714,-0.4,-0.385714285714286,
-0.371428571428571,-0.357142857142857,-0.342857142857143,-0.328571428571429,
-0.314285714285714,-0.3,-0.285714285714286,-0.271428571428571,-0.257142857142857,
-0.242857142857143,-0.228571428571429,-0.214285714285714,-0.2,-0.185714285714286,
-0.171428571428571,-0.157142857142857,-0.142857142857143,-0.128571428571429,
-0.114285714285714,-0.1,-0.0857142857142857,-0.0714285714285714,-0.0571428571428571,
-0.0428571428571429,-0.0285714285714286,-0.0142857142857143,0.),
 .UNSPECIFIED.);
#113=B_SPLINE_CURVE_WITH_KNOTS('',5,(#7084,#7085,#7086,#7087,#7088,#7089,
#7090,#7091,#7092,#7093,#7094,#7095,#7096,#7097,#7098,#7099,#7100,#7101,
#7102,#7103,#7104,#7105,#7106,#7107,#7108,#7109,#7110,#7111,#7112,#7113,
#7114,#7115,#7116,#7117,#7118,#7119,#7120,#7121,#7122,#7123,#7124,#7125,
#7126,#7127,#7128,#7129,#7130,#7131,#7132,#7133,#7134,#7135,#7136,#7137,
#7138,#7139,#7140,#7141,#7142,#7143,#7144,#7145,#7146,#7147,#7148,#7149,
#7150,#7151,#7152,#7153,#7154,#7155,#7156,#7157,#7158),.UNSPECIFIED.,.F.,
 .F.,(6,1,1,1,1,1,1,1,1,1,1,1,1,1,1,1,1,1,1,1,1,1,1,1,1,1,1,1,1,1,1,1,1,
1,1,1,1,1,1,1,1,1,1,1,1,1,1,1,1,1,1,1,1,1,1,1,1,1,1,1,1,1,1,1,1,1,1,1,1,
1,6),(0.,0.0142857142857143,0.0285714285714286,0.0428571428571429,0.0571428571428571,
0.0714285714285714,0.0857142857142857,0.1,0.114285714285714,0.128571428571429,
0.142857142857143,0.157142857142857,0.171428571428571,0.185714285714286,
0.2,0.214285714285714,0.228571428571429,0.242857142857143,0.257142857142857,
0.271428571428571,0.285714285714286,0.3,0.314285714285714,0.328571428571429,
0.342857142857143,0.357142857142857,0.371428571428571,0.385714285714286,
0.4,0.414285714285714,0.428571428571429,0.442857142857143,0.457142857142857,
0.471428571428572,0.485714285714286,0.5,0.514285714285714,0.528571428571429,
0.542857142857143,0.557142857142857,0.571428571428571,0.585714285714286,
0.6,0.614285714285714,0.628571428571428,0.642857142857142,0.657142857142857,
0.671428571428571,0.685714285714285,0.699999999999999,0.714285714285714,
0.728571428571428,0.742857142857142,0.757142857142856,0.771428571428571,
0.785714285714285,0.799999999999999,0.814285714285713,0.828571428571428,
0.842857142857142,0.857142857142856,0.87142857142857,0.885714285714284,
0.899999999999999,0.914285714285713,0.928571428571427,0.942857142857141,
0.957142857142856,0.97142857142857,0.985714285714284,1.),.UNSPECIFIED.);
#114=B_SPLINE_CURVE_WITH_KNOTS('',5,(#7159,#7160,#7161,#7162,#7163,#7164,
#7165,#7166,#7167,#7168,#7169,#7170,#7171,#7172,#7173,#7174,#7175,#7176,
#7177,#7178,#7179,#7180,#7181,#7182,#7183,#7184,#7185,#7186,#7187,#7188,
#7189,#7190,#7191,#7192,#7193,#7194,#7195,#7196,#7197,#7198,#7199,#7200,
#7201,#7202,#7203,#7204,#7205,#7206,#7207,#7208,#7209,#7210,#7211,#7212,
#7213,#7214,#7215,#7216,#7217,#7218,#7219,#7220,#7221,#7222,#7223,#7224,
#7225,#7226,#7227,#7228,#7229,#7230,#7231,#7232,#7233),.UNSPECIFIED.,.F.,
 .F.,(6,1,1,1,1,1,1,1,1,1,1,1,1,1,1,1,1,1,1,1,1,1,1,1,1,1,1,1,1,1,1,1,1,
1,1,1,1,1,1,1,1,1,1,1,1,1,1,1,1,1,1,1,1,1,1,1,1,1,1,1,1,1,1,1,1,1,1,1,1,
1,6),(0.,0.0142857142857143,0.0285714285714286,0.0428571428571429,0.0571428571428571,
0.0714285714285714,0.0857142857142857,0.1,0.114285714285714,0.128571428571429,
0.142857142857143,0.157142857142857,0.171428571428571,0.185714285714286,
0.2,0.214285714285714,0.228571428571429,0.242857142857143,0.257142857142857,
0.271428571428571,0.285714285714286,0.3,0.314285714285714,0.328571428571429,
0.342857142857143,0.357142857142857,0.371428571428571,0.385714285714286,
0.4,0.414285714285714,0.428571428571429,0.442857142857143,0.457142857142857,
0.471428571428572,0.485714285714286,0.5,0.514285714285714,0.528571428571429,
0.542857142857143,0.557142857142857,0.571428571428571,0.585714285714286,
0.6,0.614285714285714,0.628571428571428,0.642857142857142,0.657142857142857,
0.671428571428571,0.685714285714285,0.699999999999999,0.714285714285714,
0.728571428571428,0.742857142857142,0.757142857142856,0.771428571428571,
0.785714285714285,0.799999999999999,0.814285714285713,0.828571428571428,
0.842857142857142,0.857142857142856,0.87142857142857,0.885714285714284,
0.899999999999999,0.914285714285713,0.928571428571427,0.942857142857141,
0.957142857142856,0.97142857142857,0.985714285714284,1.),.UNSPECIFIED.);
#115=B_SPLINE_CURVE_WITH_KNOTS('',5,(#7385,#7386,#7387,#7388,#7389,#7390,
#7391,#7392,#7393,#7394,#7395,#7396,#7397,#7398,#7399,#7400,#7401,#7402,
#7403,#7404,#7405,#7406,#7407,#7408,#7409,#7410,#7411,#7412,#7413,#7414,
#7415,#7416,#7417,#7418,#7419,#7420,#7421,#7422,#7423,#7424,#7425,#7426,
#7427,#7428,#7429,#7430,#7431,#7432,#7433,#7434,#7435,#7436,#7437,#7438,
#7439,#7440,#7441,#7442,#7443,#7444,#7445,#7446,#7447,#7448,#7449,#7450,
#7451,#7452,#7453,#7454,#7455,#7456,#7457,#7458,#7459),.UNSPECIFIED.,.F.,
 .F.,(6,1,1,1,1,1,1,1,1,1,1,1,1,1,1,1,1,1,1,1,1,1,1,1,1,1,1,1,1,1,1,1,1,
1,1,1,1,1,1,1,1,1,1,1,1,1,1,1,1,1,1,1,1,1,1,1,1,1,1,1,1,1,1,1,1,1,1,1,1,
1,6),(-1.,-0.985714285714284,-0.97142857142857,-0.957142857142856,-0.942857142857141,
-0.928571428571427,-0.914285714285713,-0.899999999999999,-0.885714285714284,
-0.87142857142857,-0.857142857142856,-0.842857142857142,-0.828571428571428,
-0.814285714285713,-0.799999999999999,-0.785714285714285,-0.771428571428571,
-0.757142857142856,-0.742857142857142,-0.728571428571428,-0.714285714285714,
-0.699999999999999,-0.685714285714285,-0.671428571428571,-0.657142857142857,
-0.642857142857142,-0.628571428571428,-0.614285714285714,-0.6,-0.585714285714286,
-0.571428571428571,-0.557142857142857,-0.542857142857143,-0.528571428571429,
-0.514285714285714,-0.5,-0.485714285714286,-0.471428571428572,-0.457142857142857,
-0.442857142857143,-0.428571428571429,-0.414285714285714,-0.4,-0.385714285714286,
-0.371428571428571,-0.357142857142857,-0.342857142857143,-0.328571428571429,
-0.314285714285714,-0.3,-0.285714285714286,-0.271428571428571,-0.257142857142857,
-0.242857142857143,-0.228571428571429,-0.214285714285714,-0.2,-0.185714285714286,
-0.171428571428571,-0.157142857142857,-0.142857142857143,-0.128571428571429,
-0.114285714285714,-0.1,-0.0857142857142857,-0.0714285714285714,-0.0571428571428571,
-0.0428571428571429,-0.0285714285714286,-0.0142857142857143,0.),
 .UNSPECIFIED.);
#116=B_SPLINE_CURVE_WITH_KNOTS('',5,(#7461,#7462,#7463,#7464,#7465,#7466,
#7467,#7468,#7469,#7470,#7471,#7472,#7473,#7474,#7475,#7476,#7477,#7478,
#7479,#7480,#7481,#7482,#7483,#7484,#7485,#7486,#7487,#7488,#7489,#7490,
#7491,#7492,#7493,#7494,#7495,#7496,#7497,#7498,#7499,#7500,#7501,#7502,
#7503,#7504,#7505,#7506,#7507,#7508,#7509,#7510,#7511,#7512,#7513,#7514,
#7515,#7516,#7517,#7518,#7519,#7520,#7521,#7522,#7523,#7524,#7525,#7526,
#7527,#7528,#7529,#7530,#7531,#7532,#7533,#7534,#7535),.UNSPECIFIED.,.F.,
 .F.,(6,1,1,1,1,1,1,1,1,1,1,1,1,1,1,1,1,1,1,1,1,1,1,1,1,1,1,1,1,1,1,1,1,
1,1,1,1,1,1,1,1,1,1,1,1,1,1,1,1,1,1,1,1,1,1,1,1,1,1,1,1,1,1,1,1,1,1,1,1,
1,6),(-1.,-0.985714285714284,-0.97142857142857,-0.957142857142856,-0.942857142857141,
-0.928571428571427,-0.914285714285713,-0.899999999999999,-0.885714285714284,
-0.87142857142857,-0.857142857142856,-0.842857142857142,-0.828571428571428,
-0.814285714285713,-0.799999999999999,-0.785714285714285,-0.771428571428571,
-0.757142857142856,-0.742857142857142,-0.728571428571428,-0.714285714285714,
-0.699999999999999,-0.685714285714285,-0.671428571428571,-0.657142857142857,
-0.642857142857142,-0.628571428571428,-0.614285714285714,-0.6,-0.585714285714286,
-0.571428571428571,-0.557142857142857,-0.542857142857143,-0.528571428571429,
-0.514285714285714,-0.5,-0.485714285714286,-0.471428571428572,-0.457142857142857,
-0.442857142857143,-0.428571428571429,-0.414285714285714,-0.4,-0.385714285714286,
-0.371428571428571,-0.357142857142857,-0.342857142857143,-0.328571428571429,
-0.314285714285714,-0.3,-0.285714285714286,-0.271428571428571,-0.257142857142857,
-0.242857142857143,-0.228571428571429,-0.214285714285714,-0.2,-0.185714285714286,
-0.171428571428571,-0.157142857142857,-0.142857142857143,-0.128571428571429,
-0.114285714285714,-0.1,-0.0857142857142857,-0.0714285714285714,-0.0571428571428571,
-0.0428571428571429,-0.0285714285714286,-0.0142857142857143,0.),
 .UNSPECIFIED.);
#117=B_SPLINE_CURVE_WITH_KNOTS('',5,(#7693,#7694,#7695,#7696,#7697,#7698,
#7699,#7700,#7701,#7702,#7703,#7704,#7705,#7706,#7707,#7708,#7709,#7710,
#7711,#7712,#7713,#7714,#7715,#7716,#7717,#7718,#7719,#7720,#7721,#7722,
#7723,#7724,#7725,#7726,#7727,#7728,#7729,#7730,#7731,#7732,#7733,#7734,
#7735,#7736,#7737,#7738,#7739,#7740,#7741,#7742,#7743,#7744,#7745,#7746,
#7747,#7748,#7749,#7750,#7751,#7752,#7753,#7754,#7755,#7756,#7757,#7758,
#7759,#7760,#7761,#7762,#7763,#7764,#7765,#7766,#7767),.UNSPECIFIED.,.F.,
 .F.,(6,1,1,1,1,1,1,1,1,1,1,1,1,1,1,1,1,1,1,1,1,1,1,1,1,1,1,1,1,1,1,1,1,
1,1,1,1,1,1,1,1,1,1,1,1,1,1,1,1,1,1,1,1,1,1,1,1,1,1,1,1,1,1,1,1,1,1,1,1,
1,6),(0.,0.0142857142857143,0.0285714285714286,0.0428571428571429,0.0571428571428571,
0.0714285714285714,0.0857142857142857,0.1,0.114285714285714,0.128571428571429,
0.142857142857143,0.157142857142857,0.171428571428571,0.185714285714286,
0.2,0.214285714285714,0.228571428571429,0.242857142857143,0.257142857142857,
0.271428571428571,0.285714285714286,0.3,0.314285714285714,0.328571428571429,
0.342857142857143,0.357142857142857,0.371428571428571,0.385714285714286,
0.4,0.414285714285714,0.428571428571429,0.442857142857143,0.457142857142857,
0.471428571428572,0.485714285714286,0.5,0.514285714285714,0.528571428571429,
0.542857142857143,0.557142857142857,0.571428571428571,0.585714285714286,
0.6,0.614285714285714,0.628571428571428,0.642857142857142,0.657142857142857,
0.671428571428571,0.685714285714285,0.699999999999999,0.714285714285714,
0.728571428571428,0.742857142857142,0.757142857142856,0.771428571428571,
0.785714285714285,0.799999999999999,0.814285714285713,0.828571428571428,
0.842857142857142,0.857142857142856,0.87142857142857,0.885714285714284,
0.899999999999999,0.914285714285713,0.928571428571427,0.942857142857141,
0.957142857142856,0.97142857142857,0.985714285714284,1.),.UNSPECIFIED.);
#118=B_SPLINE_CURVE_WITH_KNOTS('',5,(#7768,#7769,#7770,#7771,#7772,#7773,
#7774,#7775,#7776,#7777,#7778,#7779,#7780,#7781,#7782,#7783,#7784,#7785,
#7786,#7787,#7788,#7789,#7790,#7791,#7792,#7793,#7794,#7795,#7796,#7797,
#7798,#7799,#7800,#7801,#7802,#7803,#7804,#7805,#7806,#7807,#7808,#7809,
#7810,#7811,#7812,#7813,#7814,#7815,#7816,#7817,#7818,#7819,#7820,#7821,
#7822,#7823,#7824,#7825,#7826,#7827,#7828,#7829,#7830,#7831,#7832,#7833,
#7834,#7835,#7836,#7837,#7838,#7839,#7840,#7841,#7842),.UNSPECIFIED.,.F.,
 .F.,(6,1,1,1,1,1,1,1,1,1,1,1,1,1,1,1,1,1,1,1,1,1,1,1,1,1,1,1,1,1,1,1,1,
1,1,1,1,1,1,1,1,1,1,1,1,1,1,1,1,1,1,1,1,1,1,1,1,1,1,1,1,1,1,1,1,1,1,1,1,
1,6),(0.,0.0142857142857143,0.0285714285714286,0.0428571428571429,0.0571428571428571,
0.0714285714285714,0.0857142857142857,0.1,0.114285714285714,0.128571428571429,
0.142857142857143,0.157142857142857,0.171428571428571,0.185714285714286,
0.2,0.214285714285714,0.228571428571429,0.242857142857143,0.257142857142857,
0.271428571428571,0.285714285714286,0.3,0.314285714285714,0.328571428571429,
0.342857142857143,0.357142857142857,0.371428571428571,0.385714285714286,
0.4,0.414285714285714,0.428571428571429,0.442857142857143,0.457142857142857,
0.471428571428572,0.485714285714286,0.5,0.514285714285714,0.528571428571429,
0.542857142857143,0.557142857142857,0.571428571428571,0.585714285714286,
0.6,0.614285714285714,0.628571428571428,0.642857142857142,0.657142857142857,
0.671428571428571,0.685714285714285,0.699999999999999,0.714285714285714,
0.728571428571428,0.742857142857142,0.757142857142856,0.771428571428571,
0.785714285714285,0.799999999999999,0.814285714285713,0.828571428571428,
0.842857142857142,0.857142857142856,0.87142857142857,0.885714285714284,
0.899999999999999,0.914285714285713,0.928571428571427,0.942857142857141,
0.957142857142856,0.97142857142857,0.985714285714284,1.),.UNSPECIFIED.);
#119=B_SPLINE_CURVE_WITH_KNOTS('',5,(#7854,#7855,#7856,#7857,#7858,#7859,
#7860,#7861,#7862,#7863,#7864,#7865,#7866,#7867,#7868,#7869,#7870,#7871,
#7872,#7873,#7874,#7875,#7876,#7877,#7878,#7879,#7880,#7881,#7882,#7883,
#7884,#7885,#7886,#7887,#7888,#7889,#7890,#7891,#7892,#7893,#7894,#7895,
#7896,#7897,#7898,#7899,#7900,#7901,#7902,#7903,#7904,#7905,#7906,#7907,
#7908,#7909,#7910,#7911,#7912,#7913,#7914,#7915,#7916,#7917,#7918,#7919,
#7920,#7921,#7922,#7923,#7924,#7925,#7926,#7927,#7928),.UNSPECIFIED.,.F.,
 .F.,(6,1,1,1,1,1,1,1,1,1,1,1,1,1,1,1,1,1,1,1,1,1,1,1,1,1,1,1,1,1,1,1,1,
1,1,1,1,1,1,1,1,1,1,1,1,1,1,1,1,1,1,1,1,1,1,1,1,1,1,1,1,1,1,1,1,1,1,1,1,
1,6),(-1.,-0.985714285714284,-0.97142857142857,-0.957142857142856,-0.942857142857141,
-0.928571428571427,-0.914285714285713,-0.899999999999999,-0.885714285714284,
-0.87142857142857,-0.857142857142856,-0.842857142857142,-0.828571428571428,
-0.814285714285713,-0.799999999999999,-0.785714285714285,-0.771428571428571,
-0.757142857142856,-0.742857142857142,-0.728571428571428,-0.714285714285714,
-0.699999999999999,-0.685714285714285,-0.671428571428571,-0.657142857142857,
-0.642857142857142,-0.628571428571428,-0.614285714285714,-0.6,-0.585714285714286,
-0.571428571428571,-0.557142857142857,-0.542857142857143,-0.528571428571429,
-0.514285714285714,-0.5,-0.485714285714286,-0.471428571428572,-0.457142857142857,
-0.442857142857143,-0.428571428571429,-0.414285714285714,-0.4,-0.385714285714286,
-0.371428571428571,-0.357142857142857,-0.342857142857143,-0.328571428571429,
-0.314285714285714,-0.3,-0.285714285714286,-0.271428571428571,-0.257142857142857,
-0.242857142857143,-0.228571428571429,-0.214285714285714,-0.2,-0.185714285714286,
-0.171428571428571,-0.157142857142857,-0.142857142857143,-0.128571428571429,
-0.114285714285714,-0.1,-0.0857142857142857,-0.0714285714285714,-0.0571428571428571,
-0.0428571428571429,-0.0285714285714286,-0.0142857142857143,0.),
 .UNSPECIFIED.);
#120=B_SPLINE_CURVE_WITH_KNOTS('',5,(#7932,#7933,#7934,#7935,#7936,#7937,
#7938,#7939,#7940,#7941,#7942,#7943,#7944,#7945,#7946,#7947,#7948,#7949,
#7950,#7951,#7952,#7953,#7954,#7955,#7956,#7957,#7958,#7959,#7960,#7961,
#7962,#7963,#7964,#7965,#7966,#7967,#7968,#7969,#7970,#7971,#7972,#7973,
#7974,#7975,#7976,#7977,#7978,#7979,#7980,#7981,#7982,#7983,#7984,#7985,
#7986,#7987,#7988,#7989,#7990,#7991,#7992,#7993,#7994,#7995,#7996,#7997,
#7998,#7999,#8000,#8001,#8002,#8003,#8004,#8005,#8006),.UNSPECIFIED.,.F.,
 .F.,(6,1,1,1,1,1,1,1,1,1,1,1,1,1,1,1,1,1,1,1,1,1,1,1,1,1,1,1,1,1,1,1,1,
1,1,1,1,1,1,1,1,1,1,1,1,1,1,1,1,1,1,1,1,1,1,1,1,1,1,1,1,1,1,1,1,1,1,1,1,
1,6),(0.,0.0142857142857143,0.0285714285714286,0.0428571428571429,0.0571428571428571,
0.0714285714285714,0.0857142857142857,0.1,0.114285714285714,0.128571428571429,
0.142857142857143,0.157142857142857,0.171428571428571,0.185714285714286,
0.2,0.214285714285714,0.228571428571429,0.242857142857143,0.257142857142857,
0.271428571428571,0.285714285714286,0.3,0.314285714285714,0.328571428571429,
0.342857142857143,0.357142857142857,0.371428571428571,0.385714285714286,
0.4,0.414285714285714,0.428571428571429,0.442857142857143,0.457142857142857,
0.471428571428572,0.485714285714286,0.5,0.514285714285714,0.528571428571429,
0.542857142857143,0.557142857142857,0.571428571428571,0.585714285714286,
0.6,0.614285714285714,0.628571428571428,0.642857142857142,0.657142857142857,
0.671428571428571,0.685714285714285,0.699999999999999,0.714285714285714,
0.728571428571428,0.742857142857142,0.757142857142856,0.771428571428571,
0.785714285714285,0.799999999999999,0.814285714285713,0.828571428571428,
0.842857142857142,0.857142857142856,0.87142857142857,0.885714285714284,
0.899999999999999,0.914285714285713,0.928571428571427,0.942857142857141,
0.957142857142856,0.97142857142857,0.985714285714284,1.),.UNSPECIFIED.);
#121=B_SPLINE_CURVE_WITH_KNOTS('',5,(#8196,#8197,#8198,#8199,#8200,#8201,
#8202,#8203,#8204,#8205,#8206,#8207,#8208,#8209,#8210,#8211,#8212,#8213,
#8214,#8215,#8216,#8217,#8218,#8219,#8220,#8221,#8222,#8223,#8224,#8225,
#8226,#8227,#8228,#8229,#8230,#8231,#8232,#8233,#8234,#8235,#8236,#8237,
#8238,#8239,#8240,#8241,#8242,#8243,#8244,#8245,#8246,#8247,#8248,#8249,
#8250,#8251,#8252,#8253,#8254,#8255,#8256,#8257,#8258,#8259,#8260,#8261,
#8262,#8263,#8264,#8265,#8266,#8267,#8268,#8269,#8270),.UNSPECIFIED.,.F.,
 .F.,(6,1,1,1,1,1,1,1,1,1,1,1,1,1,1,1,1,1,1,1,1,1,1,1,1,1,1,1,1,1,1,1,1,
1,1,1,1,1,1,1,1,1,1,1,1,1,1,1,1,1,1,1,1,1,1,1,1,1,1,1,1,1,1,1,1,1,1,1,1,
1,6),(-1.,-0.985714285714284,-0.97142857142857,-0.957142857142856,-0.942857142857141,
-0.928571428571427,-0.914285714285713,-0.899999999999999,-0.885714285714284,
-0.87142857142857,-0.857142857142856,-0.842857142857142,-0.828571428571428,
-0.814285714285713,-0.799999999999999,-0.785714285714285,-0.771428571428571,
-0.757142857142856,-0.742857142857142,-0.728571428571428,-0.714285714285714,
-0.699999999999999,-0.685714285714285,-0.671428571428571,-0.657142857142857,
-0.642857142857142,-0.628571428571428,-0.614285714285714,-0.6,-0.585714285714286,
-0.571428571428571,-0.557142857142857,-0.542857142857143,-0.528571428571429,
-0.514285714285714,-0.5,-0.485714285714286,-0.471428571428572,-0.457142857142857,
-0.442857142857143,-0.428571428571429,-0.414285714285714,-0.4,-0.385714285714286,
-0.371428571428571,-0.357142857142857,-0.342857142857143,-0.328571428571429,
-0.314285714285714,-0.3,-0.285714285714286,-0.271428571428571,-0.257142857142857,
-0.242857142857143,-0.228571428571429,-0.214285714285714,-0.2,-0.185714285714286,
-0.171428571428571,-0.157142857142857,-0.142857142857143,-0.128571428571429,
-0.114285714285714,-0.1,-0.0857142857142857,-0.0714285714285714,-0.0571428571428571,
-0.0428571428571429,-0.0285714285714286,-0.0142857142857143,0.),
 .UNSPECIFIED.);
#122=B_SPLINE_CURVE_WITH_KNOTS('',5,(#8426,#8427,#8428,#8429,#8430,#8431,
#8432,#8433,#8434,#8435,#8436,#8437,#8438,#8439,#8440,#8441,#8442,#8443,
#8444,#8445,#8446,#8447,#8448,#8449,#8450,#8451,#8452,#8453,#8454,#8455,
#8456,#8457,#8458,#8459,#8460,#8461,#8462,#8463,#8464,#8465,#8466,#8467,
#8468,#8469,#8470,#8471,#8472,#8473,#8474,#8475,#8476,#8477,#8478,#8479,
#8480,#8481,#8482,#8483,#8484,#8485,#8486,#8487,#8488,#8489,#8490,#8491,
#8492,#8493,#8494,#8495,#8496,#8497,#8498,#8499,#8500),.UNSPECIFIED.,.F.,
 .F.,(6,1,1,1,1,1,1,1,1,1,1,1,1,1,1,1,1,1,1,1,1,1,1,1,1,1,1,1,1,1,1,1,1,
1,1,1,1,1,1,1,1,1,1,1,1,1,1,1,1,1,1,1,1,1,1,1,1,1,1,1,1,1,1,1,1,1,1,1,1,
1,6),(0.,0.0142857142857143,0.0285714285714286,0.0428571428571429,0.0571428571428571,
0.0714285714285714,0.0857142857142857,0.1,0.114285714285714,0.128571428571429,
0.142857142857143,0.157142857142857,0.171428571428571,0.185714285714286,
0.2,0.214285714285714,0.228571428571429,0.242857142857143,0.257142857142857,
0.271428571428571,0.285714285714286,0.3,0.314285714285714,0.328571428571429,
0.342857142857143,0.357142857142857,0.371428571428571,0.385714285714286,
0.4,0.414285714285714,0.428571428571429,0.442857142857143,0.457142857142857,
0.471428571428572,0.485714285714286,0.5,0.514285714285714,0.528571428571429,
0.542857142857143,0.557142857142857,0.571428571428571,0.585714285714286,
0.6,0.614285714285714,0.628571428571428,0.642857142857142,0.657142857142857,
0.671428571428571,0.685714285714285,0.699999999999999,0.714285714285714,
0.728571428571428,0.742857142857142,0.757142857142856,0.771428571428571,
0.785714285714285,0.799999999999999,0.814285714285713,0.828571428571428,
0.842857142857142,0.857142857142856,0.87142857142857,0.885714285714284,
0.899999999999999,0.914285714285713,0.928571428571427,0.942857142857141,
0.957142857142856,0.97142857142857,0.985714285714284,1.),.UNSPECIFIED.);
#157=B_SPLINE_SURFACE_WITH_KNOTS('',5,1,((#4798,#4799),(#4800,#4801),(#4802,
#4803),(#4804,#4805),(#4806,#4807),(#4808,#4809),(#4810,#4811),(#4812,#4813),
(#4814,#4815),(#4816,#4817),(#4818,#4819),(#4820,#4821),(#4822,#4823),(#4824,
#4825),(#4826,#4827),(#4828,#4829),(#4830,#4831),(#4832,#4833),(#4834,#4835),
(#4836,#4837),(#4838,#4839),(#4840,#4841),(#4842,#4843),(#4844,#4845),(#4846,
#4847),(#4848,#4849),(#4850,#4851),(#4852,#4853),(#4854,#4855),(#4856,#4857),
(#4858,#4859),(#4860,#4861),(#4862,#4863),(#4864,#4865),(#4866,#4867),(#4868,
#4869),(#4870,#4871),(#4872,#4873),(#4874,#4875),(#4876,#4877),(#4878,#4879),
(#4880,#4881),(#4882,#4883),(#4884,#4885),(#4886,#4887),(#4888,#4889),(#4890,
#4891),(#4892,#4893),(#4894,#4895),(#4896,#4897),(#4898,#4899),(#4900,#4901),
(#4902,#4903),(#4904,#4905),(#4906,#4907),(#4908,#4909),(#4910,#4911),(#4912,
#4913),(#4914,#4915),(#4916,#4917),(#4918,#4919),(#4920,#4921),(#4922,#4923),
(#4924,#4925),(#4926,#4927),(#4928,#4929),(#4930,#4931),(#4932,#4933),(#4934,
#4935),(#4936,#4937),(#4938,#4939),(#4940,#4941),(#4942,#4943),(#4944,#4945),
(#4946,#4947)),.UNSPECIFIED.,.F.,.F.,.F.,(6,1,1,1,1,1,1,1,1,1,1,1,1,1,1,
1,1,1,1,1,1,1,1,1,1,1,1,1,1,1,1,1,1,1,1,1,1,1,1,1,1,1,1,1,1,1,1,1,1,1,1,
1,1,1,1,1,1,1,1,1,1,1,1,1,1,1,1,1,1,1,6),(2,2),(-1.,-0.985714285714284,
-0.97142857142857,-0.957142857142856,-0.942857142857141,-0.928571428571427,
-0.914285714285713,-0.899999999999999,-0.885714285714284,-0.87142857142857,
-0.857142857142856,-0.842857142857142,-0.828571428571428,-0.814285714285713,
-0.799999999999999,-0.785714285714285,-0.771428571428571,-0.757142857142856,
-0.742857142857142,-0.728571428571428,-0.714285714285714,-0.699999999999999,
-0.685714285714285,-0.671428571428571,-0.657142857142857,-0.642857142857142,
-0.628571428571428,-0.614285714285714,-0.6,-0.585714285714286,-0.571428571428571,
-0.557142857142857,-0.542857142857143,-0.528571428571429,-0.514285714285714,
-0.5,-0.485714285714286,-0.471428571428572,-0.457142857142857,-0.442857142857143,
-0.428571428571429,-0.414285714285714,-0.4,-0.385714285714286,-0.371428571428571,
-0.357142857142857,-0.342857142857143,-0.328571428571429,-0.314285714285714,
-0.3,-0.285714285714286,-0.271428571428571,-0.257142857142857,-0.242857142857143,
-0.228571428571429,-0.214285714285714,-0.2,-0.185714285714286,-0.171428571428571,
-0.157142857142857,-0.142857142857143,-0.128571428571429,-0.114285714285714,
-0.1,-0.0857142857142857,-0.0714285714285714,-0.0571428571428571,-0.0428571428571429,
-0.0285714285714286,-0.0142857142857143,0.),(0.,1.65),.UNSPECIFIED.);
#158=B_SPLINE_SURFACE_WITH_KNOTS('',5,1,((#5107,#5108),(#5109,#5110),(#5111,
#5112),(#5113,#5114),(#5115,#5116),(#5117,#5118),(#5119,#5120),(#5121,#5122),
(#5123,#5124),(#5125,#5126),(#5127,#5128),(#5129,#5130),(#5131,#5132),(#5133,
#5134),(#5135,#5136),(#5137,#5138),(#5139,#5140),(#5141,#5142),(#5143,#5144),
(#5145,#5146),(#5147,#5148),(#5149,#5150),(#5151,#5152),(#5153,#5154),(#5155,
#5156),(#5157,#5158),(#5159,#5160),(#5161,#5162),(#5163,#5164),(#5165,#5166),
(#5167,#5168),(#5169,#5170),(#5171,#5172),(#5173,#5174),(#5175,#5176),(#5177,
#5178),(#5179,#5180),(#5181,#5182),(#5183,#5184),(#5185,#5186),(#5187,#5188),
(#5189,#5190),(#5191,#5192),(#5193,#5194),(#5195,#5196),(#5197,#5198),(#5199,
#5200),(#5201,#5202),(#5203,#5204),(#5205,#5206),(#5207,#5208),(#5209,#5210),
(#5211,#5212),(#5213,#5214),(#5215,#5216),(#5217,#5218),(#5219,#5220),(#5221,
#5222),(#5223,#5224),(#5225,#5226),(#5227,#5228),(#5229,#5230),(#5231,#5232),
(#5233,#5234),(#5235,#5236),(#5237,#5238),(#5239,#5240),(#5241,#5242),(#5243,
#5244),(#5245,#5246),(#5247,#5248),(#5249,#5250),(#5251,#5252),(#5253,#5254),
(#5255,#5256)),.UNSPECIFIED.,.F.,.F.,.F.,(6,1,1,1,1,1,1,1,1,1,1,1,1,1,1,
1,1,1,1,1,1,1,1,1,1,1,1,1,1,1,1,1,1,1,1,1,1,1,1,1,1,1,1,1,1,1,1,1,1,1,1,
1,1,1,1,1,1,1,1,1,1,1,1,1,1,1,1,1,1,1,6),(2,2),(0.,0.0142857142857143,0.0285714285714286,
0.0428571428571429,0.0571428571428571,0.0714285714285714,0.0857142857142857,
0.1,0.114285714285714,0.128571428571429,0.142857142857143,0.157142857142857,
0.171428571428571,0.185714285714286,0.2,0.214285714285714,0.228571428571429,
0.242857142857143,0.257142857142857,0.271428571428571,0.285714285714286,
0.3,0.314285714285714,0.328571428571429,0.342857142857143,0.357142857142857,
0.371428571428571,0.385714285714286,0.4,0.414285714285714,0.428571428571429,
0.442857142857143,0.457142857142857,0.471428571428572,0.485714285714286,
0.5,0.514285714285714,0.528571428571429,0.542857142857143,0.557142857142857,
0.571428571428571,0.585714285714286,0.6,0.614285714285714,0.628571428571428,
0.642857142857142,0.657142857142857,0.671428571428571,0.685714285714285,
0.699999999999999,0.714285714285714,0.728571428571428,0.742857142857142,
0.757142857142856,0.771428571428571,0.785714285714285,0.799999999999999,
0.814285714285713,0.828571428571428,0.842857142857142,0.857142857142856,
0.87142857142857,0.885714285714284,0.899999999999999,0.914285714285713,
0.928571428571427,0.942857142857141,0.957142857142856,0.97142857142857,
0.985714285714284,1.),(0.,1.65),.UNSPECIFIED.);
#159=B_SPLINE_SURFACE_WITH_KNOTS('',5,1,((#5407,#5408),(#5409,#5410),(#5411,
#5412),(#5413,#5414),(#5415,#5416),(#5417,#5418),(#5419,#5420),(#5421,#5422),
(#5423,#5424),(#5425,#5426),(#5427,#5428),(#5429,#5430),(#5431,#5432),(#5433,
#5434),(#5435,#5436),(#5437,#5438),(#5439,#5440),(#5441,#5442),(#5443,#5444),
(#5445,#5446),(#5447,#5448),(#5449,#5450),(#5451,#5452),(#5453,#5454),(#5455,
#5456),(#5457,#5458),(#5459,#5460),(#5461,#5462),(#5463,#5464),(#5465,#5466),
(#5467,#5468),(#5469,#5470),(#5471,#5472),(#5473,#5474),(#5475,#5476),(#5477,
#5478),(#5479,#5480),(#5481,#5482),(#5483,#5484),(#5485,#5486),(#5487,#5488),
(#5489,#5490),(#5491,#5492),(#5493,#5494),(#5495,#5496),(#5497,#5498),(#5499,
#5500),(#5501,#5502),(#5503,#5504),(#5505,#5506),(#5507,#5508),(#5509,#5510),
(#5511,#5512),(#5513,#5514),(#5515,#5516),(#5517,#5518),(#5519,#5520),(#5521,
#5522),(#5523,#5524),(#5525,#5526),(#5527,#5528),(#5529,#5530),(#5531,#5532),
(#5533,#5534),(#5535,#5536),(#5537,#5538),(#5539,#5540),(#5541,#5542),(#5543,
#5544),(#5545,#5546),(#5547,#5548),(#5549,#5550),(#5551,#5552),(#5553,#5554),
(#5555,#5556)),.UNSPECIFIED.,.F.,.F.,.F.,(6,1,1,1,1,1,1,1,1,1,1,1,1,1,1,
1,1,1,1,1,1,1,1,1,1,1,1,1,1,1,1,1,1,1,1,1,1,1,1,1,1,1,1,1,1,1,1,1,1,1,1,
1,1,1,1,1,1,1,1,1,1,1,1,1,1,1,1,1,1,1,6),(2,2),(-1.,-0.985714285714284,
-0.97142857142857,-0.957142857142856,-0.942857142857141,-0.928571428571427,
-0.914285714285713,-0.899999999999999,-0.885714285714284,-0.87142857142857,
-0.857142857142856,-0.842857142857142,-0.828571428571428,-0.814285714285713,
-0.799999999999999,-0.785714285714285,-0.771428571428571,-0.757142857142856,
-0.742857142857142,-0.728571428571428,-0.714285714285714,-0.699999999999999,
-0.685714285714285,-0.671428571428571,-0.657142857142857,-0.642857142857142,
-0.628571428571428,-0.614285714285714,-0.6,-0.585714285714286,-0.571428571428571,
-0.557142857142857,-0.542857142857143,-0.528571428571429,-0.514285714285714,
-0.5,-0.485714285714286,-0.471428571428572,-0.457142857142857,-0.442857142857143,
-0.428571428571429,-0.414285714285714,-0.4,-0.385714285714286,-0.371428571428571,
-0.357142857142857,-0.342857142857143,-0.328571428571429,-0.314285714285714,
-0.3,-0.285714285714286,-0.271428571428571,-0.257142857142857,-0.242857142857143,
-0.228571428571429,-0.214285714285714,-0.2,-0.185714285714286,-0.171428571428571,
-0.157142857142857,-0.142857142857143,-0.128571428571429,-0.114285714285714,
-0.1,-0.0857142857142857,-0.0714285714285714,-0.0571428571428571,-0.0428571428571429,
-0.0285714285714286,-0.0142857142857143,0.),(0.,1.65),.UNSPECIFIED.);
#160=B_SPLINE_SURFACE_WITH_KNOTS('',5,1,((#5716,#5717),(#5718,#5719),(#5720,
#5721),(#5722,#5723),(#5724,#5725),(#5726,#5727),(#5728,#5729),(#5730,#5731),
(#5732,#5733),(#5734,#5735),(#5736,#5737),(#5738,#5739),(#5740,#5741),(#5742,
#5743),(#5744,#5745),(#5746,#5747),(#5748,#5749),(#5750,#5751),(#5752,#5753),
(#5754,#5755),(#5756,#5757),(#5758,#5759),(#5760,#5761),(#5762,#5763),(#5764,
#5765),(#5766,#5767),(#5768,#5769),(#5770,#5771),(#5772,#5773),(#5774,#5775),
(#5776,#5777),(#5778,#5779),(#5780,#5781),(#5782,#5783),(#5784,#5785),(#5786,
#5787),(#5788,#5789),(#5790,#5791),(#5792,#5793),(#5794,#5795),(#5796,#5797),
(#5798,#5799),(#5800,#5801),(#5802,#5803),(#5804,#5805),(#5806,#5807),(#5808,
#5809),(#5810,#5811),(#5812,#5813),(#5814,#5815),(#5816,#5817),(#5818,#5819),
(#5820,#5821),(#5822,#5823),(#5824,#5825),(#5826,#5827),(#5828,#5829),(#5830,
#5831),(#5832,#5833),(#5834,#5835),(#5836,#5837),(#5838,#5839),(#5840,#5841),
(#5842,#5843),(#5844,#5845),(#5846,#5847),(#5848,#5849),(#5850,#5851),(#5852,
#5853),(#5854,#5855),(#5856,#5857),(#5858,#5859),(#5860,#5861),(#5862,#5863),
(#5864,#5865)),.UNSPECIFIED.,.F.,.F.,.F.,(6,1,1,1,1,1,1,1,1,1,1,1,1,1,1,
1,1,1,1,1,1,1,1,1,1,1,1,1,1,1,1,1,1,1,1,1,1,1,1,1,1,1,1,1,1,1,1,1,1,1,1,
1,1,1,1,1,1,1,1,1,1,1,1,1,1,1,1,1,1,1,6),(2,2),(0.,0.0142857142857143,0.0285714285714286,
0.0428571428571429,0.0571428571428571,0.0714285714285714,0.0857142857142857,
0.1,0.114285714285714,0.128571428571429,0.142857142857143,0.157142857142857,
0.171428571428571,0.185714285714286,0.2,0.214285714285714,0.228571428571429,
0.242857142857143,0.257142857142857,0.271428571428571,0.285714285714286,
0.3,0.314285714285714,0.328571428571429,0.342857142857143,0.357142857142857,
0.371428571428571,0.385714285714286,0.4,0.414285714285714,0.428571428571429,
0.442857142857143,0.457142857142857,0.471428571428572,0.485714285714286,
0.5,0.514285714285714,0.528571428571429,0.542857142857143,0.557142857142857,
0.571428571428571,0.585714285714286,0.6,0.614285714285714,0.628571428571428,
0.642857142857142,0.657142857142857,0.671428571428571,0.685714285714285,
0.699999999999999,0.714285714285714,0.728571428571428,0.742857142857142,
0.757142857142856,0.771428571428571,0.785714285714285,0.799999999999999,
0.814285714285713,0.828571428571428,0.842857142857142,0.857142857142856,
0.87142857142857,0.885714285714284,0.899999999999999,0.914285714285713,
0.928571428571427,0.942857142857141,0.957142857142856,0.97142857142857,
0.985714285714284,1.),(0.,1.65),.UNSPECIFIED.);
#161=B_SPLINE_SURFACE_WITH_KNOTS('',5,1,((#6016,#6017),(#6018,#6019),(#6020,
#6021),(#6022,#6023),(#6024,#6025),(#6026,#6027),(#6028,#6029),(#6030,#6031),
(#6032,#6033),(#6034,#6035),(#6036,#6037),(#6038,#6039),(#6040,#6041),(#6042,
#6043),(#6044,#6045),(#6046,#6047),(#6048,#6049),(#6050,#6051),(#6052,#6053),
(#6054,#6055),(#6056,#6057),(#6058,#6059),(#6060,#6061),(#6062,#6063),(#6064,
#6065),(#6066,#6067),(#6068,#6069),(#6070,#6071),(#6072,#6073),(#6074,#6075),
(#6076,#6077),(#6078,#6079),(#6080,#6081),(#6082,#6083),(#6084,#6085),(#6086,
#6087),(#6088,#6089),(#6090,#6091),(#6092,#6093),(#6094,#6095),(#6096,#6097),
(#6098,#6099),(#6100,#6101),(#6102,#6103),(#6104,#6105),(#6106,#6107),(#6108,
#6109),(#6110,#6111),(#6112,#6113),(#6114,#6115),(#6116,#6117),(#6118,#6119),
(#6120,#6121),(#6122,#6123),(#6124,#6125),(#6126,#6127),(#6128,#6129),(#6130,
#6131),(#6132,#6133),(#6134,#6135),(#6136,#6137),(#6138,#6139),(#6140,#6141),
(#6142,#6143),(#6144,#6145),(#6146,#6147),(#6148,#6149),(#6150,#6151),(#6152,
#6153),(#6154,#6155),(#6156,#6157),(#6158,#6159),(#6160,#6161),(#6162,#6163),
(#6164,#6165)),.UNSPECIFIED.,.F.,.F.,.F.,(6,1,1,1,1,1,1,1,1,1,1,1,1,1,1,
1,1,1,1,1,1,1,1,1,1,1,1,1,1,1,1,1,1,1,1,1,1,1,1,1,1,1,1,1,1,1,1,1,1,1,1,
1,1,1,1,1,1,1,1,1,1,1,1,1,1,1,1,1,1,1,6),(2,2),(-1.,-0.985714285714284,
-0.97142857142857,-0.957142857142856,-0.942857142857141,-0.928571428571427,
-0.914285714285713,-0.899999999999999,-0.885714285714284,-0.87142857142857,
-0.857142857142856,-0.842857142857142,-0.828571428571428,-0.814285714285713,
-0.799999999999999,-0.785714285714285,-0.771428571428571,-0.757142857142856,
-0.742857142857142,-0.728571428571428,-0.714285714285714,-0.699999999999999,
-0.685714285714285,-0.671428571428571,-0.657142857142857,-0.642857142857142,
-0.628571428571428,-0.614285714285714,-0.6,-0.585714285714286,-0.571428571428571,
-0.557142857142857,-0.542857142857143,-0.528571428571429,-0.514285714285714,
-0.5,-0.485714285714286,-0.471428571428572,-0.457142857142857,-0.442857142857143,
-0.428571428571429,-0.414285714285714,-0.4,-0.385714285714286,-0.371428571428571,
-0.357142857142857,-0.342857142857143,-0.328571428571429,-0.314285714285714,
-0.3,-0.285714285714286,-0.271428571428571,-0.257142857142857,-0.242857142857143,
-0.228571428571429,-0.214285714285714,-0.2,-0.185714285714286,-0.171428571428571,
-0.157142857142857,-0.142857142857143,-0.128571428571429,-0.114285714285714,
-0.1,-0.0857142857142857,-0.0714285714285714,-0.0571428571428571,-0.0428571428571429,
-0.0285714285714286,-0.0142857142857143,0.),(0.,1.65),.UNSPECIFIED.);
#162=B_SPLINE_SURFACE_WITH_KNOTS('',5,1,((#6325,#6326),(#6327,#6328),(#6329,
#6330),(#6331,#6332),(#6333,#6334),(#6335,#6336),(#6337,#6338),(#6339,#6340),
(#6341,#6342),(#6343,#6344),(#6345,#6346),(#6347,#6348),(#6349,#6350),(#6351,
#6352),(#6353,#6354),(#6355,#6356),(#6357,#6358),(#6359,#6360),(#6361,#6362),
(#6363,#6364),(#6365,#6366),(#6367,#6368),(#6369,#6370),(#6371,#6372),(#6373,
#6374),(#6375,#6376),(#6377,#6378),(#6379,#6380),(#6381,#6382),(#6383,#6384),
(#6385,#6386),(#6387,#6388),(#6389,#6390),(#6391,#6392),(#6393,#6394),(#6395,
#6396),(#6397,#6398),(#6399,#6400),(#6401,#6402),(#6403,#6404),(#6405,#6406),
(#6407,#6408),(#6409,#6410),(#6411,#6412),(#6413,#6414),(#6415,#6416),(#6417,
#6418),(#6419,#6420),(#6421,#6422),(#6423,#6424),(#6425,#6426),(#6427,#6428),
(#6429,#6430),(#6431,#6432),(#6433,#6434),(#6435,#6436),(#6437,#6438),(#6439,
#6440),(#6441,#6442),(#6443,#6444),(#6445,#6446),(#6447,#6448),(#6449,#6450),
(#6451,#6452),(#6453,#6454),(#6455,#6456),(#6457,#6458),(#6459,#6460),(#6461,
#6462),(#6463,#6464),(#6465,#6466),(#6467,#6468),(#6469,#6470),(#6471,#6472),
(#6473,#6474)),.UNSPECIFIED.,.F.,.F.,.F.,(6,1,1,1,1,1,1,1,1,1,1,1,1,1,1,
1,1,1,1,1,1,1,1,1,1,1,1,1,1,1,1,1,1,1,1,1,1,1,1,1,1,1,1,1,1,1,1,1,1,1,1,
1,1,1,1,1,1,1,1,1,1,1,1,1,1,1,1,1,1,1,6),(2,2),(0.,0.0142857142857143,0.0285714285714286,
0.0428571428571429,0.0571428571428571,0.0714285714285714,0.0857142857142857,
0.1,0.114285714285714,0.128571428571429,0.142857142857143,0.157142857142857,
0.171428571428571,0.185714285714286,0.2,0.214285714285714,0.228571428571429,
0.242857142857143,0.257142857142857,0.271428571428571,0.285714285714286,
0.3,0.314285714285714,0.328571428571429,0.342857142857143,0.357142857142857,
0.371428571428571,0.385714285714286,0.4,0.414285714285714,0.428571428571429,
0.442857142857143,0.457142857142857,0.471428571428572,0.485714285714286,
0.5,0.514285714285714,0.528571428571429,0.542857142857143,0.557142857142857,
0.571428571428571,0.585714285714286,0.6,0.614285714285714,0.628571428571428,
0.642857142857142,0.657142857142857,0.671428571428571,0.685714285714285,
0.699999999999999,0.714285714285714,0.728571428571428,0.742857142857142,
0.757142857142856,0.771428571428571,0.785714285714285,0.799999999999999,
0.814285714285713,0.828571428571428,0.842857142857142,0.857142857142856,
0.87142857142857,0.885714285714284,0.899999999999999,0.914285714285713,
0.928571428571427,0.942857142857141,0.957142857142856,0.97142857142857,
0.985714285714284,1.),(0.,1.65),.UNSPECIFIED.);
#163=B_SPLINE_SURFACE_WITH_KNOTS('',5,1,((#6625,#6626),(#6627,#6628),(#6629,
#6630),(#6631,#6632),(#6633,#6634),(#6635,#6636),(#6637,#6638),(#6639,#6640),
(#6641,#6642),(#6643,#6644),(#6645,#6646),(#6647,#6648),(#6649,#6650),(#6651,
#6652),(#6653,#6654),(#6655,#6656),(#6657,#6658),(#6659,#6660),(#6661,#6662),
(#6663,#6664),(#6665,#6666),(#6667,#6668),(#6669,#6670),(#6671,#6672),(#6673,
#6674),(#6675,#6676),(#6677,#6678),(#6679,#6680),(#6681,#6682),(#6683,#6684),
(#6685,#6686),(#6687,#6688),(#6689,#6690),(#6691,#6692),(#6693,#6694),(#6695,
#6696),(#6697,#6698),(#6699,#6700),(#6701,#6702),(#6703,#6704),(#6705,#6706),
(#6707,#6708),(#6709,#6710),(#6711,#6712),(#6713,#6714),(#6715,#6716),(#6717,
#6718),(#6719,#6720),(#6721,#6722),(#6723,#6724),(#6725,#6726),(#6727,#6728),
(#6729,#6730),(#6731,#6732),(#6733,#6734),(#6735,#6736),(#6737,#6738),(#6739,
#6740),(#6741,#6742),(#6743,#6744),(#6745,#6746),(#6747,#6748),(#6749,#6750),
(#6751,#6752),(#6753,#6754),(#6755,#6756),(#6757,#6758),(#6759,#6760),(#6761,
#6762),(#6763,#6764),(#6765,#6766),(#6767,#6768),(#6769,#6770),(#6771,#6772),
(#6773,#6774)),.UNSPECIFIED.,.F.,.F.,.F.,(6,1,1,1,1,1,1,1,1,1,1,1,1,1,1,
1,1,1,1,1,1,1,1,1,1,1,1,1,1,1,1,1,1,1,1,1,1,1,1,1,1,1,1,1,1,1,1,1,1,1,1,
1,1,1,1,1,1,1,1,1,1,1,1,1,1,1,1,1,1,1,6),(2,2),(-1.,-0.985714285714284,
-0.97142857142857,-0.957142857142856,-0.942857142857141,-0.928571428571427,
-0.914285714285713,-0.899999999999999,-0.885714285714284,-0.87142857142857,
-0.857142857142856,-0.842857142857142,-0.828571428571428,-0.814285714285713,
-0.799999999999999,-0.785714285714285,-0.771428571428571,-0.757142857142856,
-0.742857142857142,-0.728571428571428,-0.714285714285714,-0.699999999999999,
-0.685714285714285,-0.671428571428571,-0.657142857142857,-0.642857142857142,
-0.628571428571428,-0.614285714285714,-0.6,-0.585714285714286,-0.571428571428571,
-0.557142857142857,-0.542857142857143,-0.528571428571429,-0.514285714285714,
-0.5,-0.485714285714286,-0.471428571428572,-0.457142857142857,-0.442857142857143,
-0.428571428571429,-0.414285714285714,-0.4,-0.385714285714286,-0.371428571428571,
-0.357142857142857,-0.342857142857143,-0.328571428571429,-0.314285714285714,
-0.3,-0.285714285714286,-0.271428571428571,-0.257142857142857,-0.242857142857143,
-0.228571428571429,-0.214285714285714,-0.2,-0.185714285714286,-0.171428571428571,
-0.157142857142857,-0.142857142857143,-0.128571428571429,-0.114285714285714,
-0.1,-0.0857142857142857,-0.0714285714285714,-0.0571428571428571,-0.0428571428571429,
-0.0285714285714286,-0.0142857142857143,0.),(0.,1.65),.UNSPECIFIED.);
#164=B_SPLINE_SURFACE_WITH_KNOTS('',5,1,((#6934,#6935),(#6936,#6937),(#6938,
#6939),(#6940,#6941),(#6942,#6943),(#6944,#6945),(#6946,#6947),(#6948,#6949),
(#6950,#6951),(#6952,#6953),(#6954,#6955),(#6956,#6957),(#6958,#6959),(#6960,
#6961),(#6962,#6963),(#6964,#6965),(#6966,#6967),(#6968,#6969),(#6970,#6971),
(#6972,#6973),(#6974,#6975),(#6976,#6977),(#6978,#6979),(#6980,#6981),(#6982,
#6983),(#6984,#6985),(#6986,#6987),(#6988,#6989),(#6990,#6991),(#6992,#6993),
(#6994,#6995),(#6996,#6997),(#6998,#6999),(#7000,#7001),(#7002,#7003),(#7004,
#7005),(#7006,#7007),(#7008,#7009),(#7010,#7011),(#7012,#7013),(#7014,#7015),
(#7016,#7017),(#7018,#7019),(#7020,#7021),(#7022,#7023),(#7024,#7025),(#7026,
#7027),(#7028,#7029),(#7030,#7031),(#7032,#7033),(#7034,#7035),(#7036,#7037),
(#7038,#7039),(#7040,#7041),(#7042,#7043),(#7044,#7045),(#7046,#7047),(#7048,
#7049),(#7050,#7051),(#7052,#7053),(#7054,#7055),(#7056,#7057),(#7058,#7059),
(#7060,#7061),(#7062,#7063),(#7064,#7065),(#7066,#7067),(#7068,#7069),(#7070,
#7071),(#7072,#7073),(#7074,#7075),(#7076,#7077),(#7078,#7079),(#7080,#7081),
(#7082,#7083)),.UNSPECIFIED.,.F.,.F.,.F.,(6,1,1,1,1,1,1,1,1,1,1,1,1,1,1,
1,1,1,1,1,1,1,1,1,1,1,1,1,1,1,1,1,1,1,1,1,1,1,1,1,1,1,1,1,1,1,1,1,1,1,1,
1,1,1,1,1,1,1,1,1,1,1,1,1,1,1,1,1,1,1,6),(2,2),(0.,0.0142857142857143,0.0285714285714286,
0.0428571428571429,0.0571428571428571,0.0714285714285714,0.0857142857142857,
0.1,0.114285714285714,0.128571428571429,0.142857142857143,0.157142857142857,
0.171428571428571,0.185714285714286,0.2,0.214285714285714,0.228571428571429,
0.242857142857143,0.257142857142857,0.271428571428571,0.285714285714286,
0.3,0.314285714285714,0.328571428571429,0.342857142857143,0.357142857142857,
0.371428571428571,0.385714285714286,0.4,0.414285714285714,0.428571428571429,
0.442857142857143,0.457142857142857,0.471428571428572,0.485714285714286,
0.5,0.514285714285714,0.528571428571429,0.542857142857143,0.557142857142857,
0.571428571428571,0.585714285714286,0.6,0.614285714285714,0.628571428571428,
0.642857142857142,0.657142857142857,0.671428571428571,0.685714285714285,
0.699999999999999,0.714285714285714,0.728571428571428,0.742857142857142,
0.757142857142856,0.771428571428571,0.785714285714285,0.799999999999999,
0.814285714285713,0.828571428571428,0.842857142857142,0.857142857142856,
0.87142857142857,0.885714285714284,0.899999999999999,0.914285714285713,
0.928571428571427,0.942857142857141,0.957142857142856,0.97142857142857,
0.985714285714284,1.),(0.,1.65),.UNSPECIFIED.);
#165=B_SPLINE_SURFACE_WITH_KNOTS('',5,1,((#7234,#7235),(#7236,#7237),(#7238,
#7239),(#7240,#7241),(#7242,#7243),(#7244,#7245),(#7246,#7247),(#7248,#7249),
(#7250,#7251),(#7252,#7253),(#7254,#7255),(#7256,#7257),(#7258,#7259),(#7260,
#7261),(#7262,#7263),(#7264,#7265),(#7266,#7267),(#7268,#7269),(#7270,#7271),
(#7272,#7273),(#7274,#7275),(#7276,#7277),(#7278,#7279),(#7280,#7281),(#7282,
#7283),(#7284,#7285),(#7286,#7287),(#7288,#7289),(#7290,#7291),(#7292,#7293),
(#7294,#7295),(#7296,#7297),(#7298,#7299),(#7300,#7301),(#7302,#7303),(#7304,
#7305),(#7306,#7307),(#7308,#7309),(#7310,#7311),(#7312,#7313),(#7314,#7315),
(#7316,#7317),(#7318,#7319),(#7320,#7321),(#7322,#7323),(#7324,#7325),(#7326,
#7327),(#7328,#7329),(#7330,#7331),(#7332,#7333),(#7334,#7335),(#7336,#7337),
(#7338,#7339),(#7340,#7341),(#7342,#7343),(#7344,#7345),(#7346,#7347),(#7348,
#7349),(#7350,#7351),(#7352,#7353),(#7354,#7355),(#7356,#7357),(#7358,#7359),
(#7360,#7361),(#7362,#7363),(#7364,#7365),(#7366,#7367),(#7368,#7369),(#7370,
#7371),(#7372,#7373),(#7374,#7375),(#7376,#7377),(#7378,#7379),(#7380,#7381),
(#7382,#7383)),.UNSPECIFIED.,.F.,.F.,.F.,(6,1,1,1,1,1,1,1,1,1,1,1,1,1,1,
1,1,1,1,1,1,1,1,1,1,1,1,1,1,1,1,1,1,1,1,1,1,1,1,1,1,1,1,1,1,1,1,1,1,1,1,
1,1,1,1,1,1,1,1,1,1,1,1,1,1,1,1,1,1,1,6),(2,2),(-1.,-0.985714285714284,
-0.97142857142857,-0.957142857142856,-0.942857142857141,-0.928571428571427,
-0.914285714285713,-0.899999999999999,-0.885714285714284,-0.87142857142857,
-0.857142857142856,-0.842857142857142,-0.828571428571428,-0.814285714285713,
-0.799999999999999,-0.785714285714285,-0.771428571428571,-0.757142857142856,
-0.742857142857142,-0.728571428571428,-0.714285714285714,-0.699999999999999,
-0.685714285714285,-0.671428571428571,-0.657142857142857,-0.642857142857142,
-0.628571428571428,-0.614285714285714,-0.6,-0.585714285714286,-0.571428571428571,
-0.557142857142857,-0.542857142857143,-0.528571428571429,-0.514285714285714,
-0.5,-0.485714285714286,-0.471428571428572,-0.457142857142857,-0.442857142857143,
-0.428571428571429,-0.414285714285714,-0.4,-0.385714285714286,-0.371428571428571,
-0.357142857142857,-0.342857142857143,-0.328571428571429,-0.314285714285714,
-0.3,-0.285714285714286,-0.271428571428571,-0.257142857142857,-0.242857142857143,
-0.228571428571429,-0.214285714285714,-0.2,-0.185714285714286,-0.171428571428571,
-0.157142857142857,-0.142857142857143,-0.128571428571429,-0.114285714285714,
-0.1,-0.0857142857142857,-0.0714285714285714,-0.0571428571428571,-0.0428571428571429,
-0.0285714285714286,-0.0142857142857143,0.),(0.,1.65),.UNSPECIFIED.);
#166=B_SPLINE_SURFACE_WITH_KNOTS('',5,1,((#7543,#7544),(#7545,#7546),(#7547,
#7548),(#7549,#7550),(#7551,#7552),(#7553,#7554),(#7555,#7556),(#7557,#7558),
(#7559,#7560),(#7561,#7562),(#7563,#7564),(#7565,#7566),(#7567,#7568),(#7569,
#7570),(#7571,#7572),(#7573,#7574),(#7575,#7576),(#7577,#7578),(#7579,#7580),
(#7581,#7582),(#7583,#7584),(#7585,#7586),(#7587,#7588),(#7589,#7590),(#7591,
#7592),(#7593,#7594),(#7595,#7596),(#7597,#7598),(#7599,#7600),(#7601,#7602),
(#7603,#7604),(#7605,#7606),(#7607,#7608),(#7609,#7610),(#7611,#7612),(#7613,
#7614),(#7615,#7616),(#7617,#7618),(#7619,#7620),(#7621,#7622),(#7623,#7624),
(#7625,#7626),(#7627,#7628),(#7629,#7630),(#7631,#7632),(#7633,#7634),(#7635,
#7636),(#7637,#7638),(#7639,#7640),(#7641,#7642),(#7643,#7644),(#7645,#7646),
(#7647,#7648),(#7649,#7650),(#7651,#7652),(#7653,#7654),(#7655,#7656),(#7657,
#7658),(#7659,#7660),(#7661,#7662),(#7663,#7664),(#7665,#7666),(#7667,#7668),
(#7669,#7670),(#7671,#7672),(#7673,#7674),(#7675,#7676),(#7677,#7678),(#7679,
#7680),(#7681,#7682),(#7683,#7684),(#7685,#7686),(#7687,#7688),(#7689,#7690),
(#7691,#7692)),.UNSPECIFIED.,.F.,.F.,.F.,(6,1,1,1,1,1,1,1,1,1,1,1,1,1,1,
1,1,1,1,1,1,1,1,1,1,1,1,1,1,1,1,1,1,1,1,1,1,1,1,1,1,1,1,1,1,1,1,1,1,1,1,
1,1,1,1,1,1,1,1,1,1,1,1,1,1,1,1,1,1,1,6),(2,2),(0.,0.0142857142857143,0.0285714285714286,
0.0428571428571429,0.0571428571428571,0.0714285714285714,0.0857142857142857,
0.1,0.114285714285714,0.128571428571429,0.142857142857143,0.157142857142857,
0.171428571428571,0.185714285714286,0.2,0.214285714285714,0.228571428571429,
0.242857142857143,0.257142857142857,0.271428571428571,0.285714285714286,
0.3,0.314285714285714,0.328571428571429,0.342857142857143,0.357142857142857,
0.371428571428571,0.385714285714286,0.4,0.414285714285714,0.428571428571429,
0.442857142857143,0.457142857142857,0.471428571428572,0.485714285714286,
0.5,0.514285714285714,0.528571428571429,0.542857142857143,0.557142857142857,
0.571428571428571,0.585714285714286,0.6,0.614285714285714,0.628571428571428,
0.642857142857142,0.657142857142857,0.671428571428571,0.685714285714285,
0.699999999999999,0.714285714285714,0.728571428571428,0.742857142857142,
0.757142857142856,0.771428571428571,0.785714285714285,0.799999999999999,
0.814285714285713,0.828571428571428,0.842857142857142,0.857142857142856,
0.87142857142857,0.885714285714284,0.899999999999999,0.914285714285713,
0.928571428571427,0.942857142857141,0.957142857142856,0.97142857142857,
0.985714285714284,1.),(0.,1.65),.UNSPECIFIED.);
#167=B_SPLINE_SURFACE_WITH_KNOTS('',5,1,((#8045,#8046),(#8047,#8048),(#8049,
#8050),(#8051,#8052),(#8053,#8054),(#8055,#8056),(#8057,#8058),(#8059,#8060),
(#8061,#8062),(#8063,#8064),(#8065,#8066),(#8067,#8068),(#8069,#8070),(#8071,
#8072),(#8073,#8074),(#8075,#8076),(#8077,#8078),(#8079,#8080),(#8081,#8082),
(#8083,#8084),(#8085,#8086),(#8087,#8088),(#8089,#8090),(#8091,#8092),(#8093,
#8094),(#8095,#8096),(#8097,#8098),(#8099,#8100),(#8101,#8102),(#8103,#8104),
(#8105,#8106),(#8107,#8108),(#8109,#8110),(#8111,#8112),(#8113,#8114),(#8115,
#8116),(#8117,#8118),(#8119,#8120),(#8121,#8122),(#8123,#8124),(#8125,#8126),
(#8127,#8128),(#8129,#8130),(#8131,#8132),(#8133,#8134),(#8135,#8136),(#8137,
#8138),(#8139,#8140),(#8141,#8142),(#8143,#8144),(#8145,#8146),(#8147,#8148),
(#8149,#8150),(#8151,#8152),(#8153,#8154),(#8155,#8156),(#8157,#8158),(#8159,
#8160),(#8161,#8162),(#8163,#8164),(#8165,#8166),(#8167,#8168),(#8169,#8170),
(#8171,#8172),(#8173,#8174),(#8175,#8176),(#8177,#8178),(#8179,#8180),(#8181,
#8182),(#8183,#8184),(#8185,#8186),(#8187,#8188),(#8189,#8190),(#8191,#8192),
(#8193,#8194)),.UNSPECIFIED.,.F.,.F.,.F.,(6,1,1,1,1,1,1,1,1,1,1,1,1,1,1,
1,1,1,1,1,1,1,1,1,1,1,1,1,1,1,1,1,1,1,1,1,1,1,1,1,1,1,1,1,1,1,1,1,1,1,1,
1,1,1,1,1,1,1,1,1,1,1,1,1,1,1,1,1,1,1,6),(2,2),(-1.,-0.985714285714284,
-0.97142857142857,-0.957142857142856,-0.942857142857141,-0.928571428571427,
-0.914285714285713,-0.899999999999999,-0.885714285714284,-0.87142857142857,
-0.857142857142856,-0.842857142857142,-0.828571428571428,-0.814285714285713,
-0.799999999999999,-0.785714285714285,-0.771428571428571,-0.757142857142856,
-0.742857142857142,-0.728571428571428,-0.714285714285714,-0.699999999999999,
-0.685714285714285,-0.671428571428571,-0.657142857142857,-0.642857142857142,
-0.628571428571428,-0.614285714285714,-0.6,-0.585714285714286,-0.571428571428571,
-0.557142857142857,-0.542857142857143,-0.528571428571429,-0.514285714285714,
-0.5,-0.485714285714286,-0.471428571428572,-0.457142857142857,-0.442857142857143,
-0.428571428571429,-0.414285714285714,-0.4,-0.385714285714286,-0.371428571428571,
-0.357142857142857,-0.342857142857143,-0.328571428571429,-0.314285714285714,
-0.3,-0.285714285714286,-0.271428571428571,-0.257142857142857,-0.242857142857143,
-0.228571428571429,-0.214285714285714,-0.2,-0.185714285714286,-0.171428571428571,
-0.157142857142857,-0.142857142857143,-0.128571428571429,-0.114285714285714,
-0.1,-0.0857142857142857,-0.0714285714285714,-0.0571428571428571,-0.0428571428571429,
-0.0285714285714286,-0.0142857142857143,0.),(0.,1.65),.UNSPECIFIED.);
#168=B_SPLINE_SURFACE_WITH_KNOTS('',5,1,((#8276,#8277),(#8278,#8279),(#8280,
#8281),(#8282,#8283),(#8284,#8285),(#8286,#8287),(#8288,#8289),(#8290,#8291),
(#8292,#8293),(#8294,#8295),(#8296,#8297),(#8298,#8299),(#8300,#8301),(#8302,
#8303),(#8304,#8305),(#8306,#8307),(#8308,#8309),(#8310,#8311),(#8312,#8313),
(#8314,#8315),(#8316,#8317),(#8318,#8319),(#8320,#8321),(#8322,#8323),(#8324,
#8325),(#8326,#8327),(#8328,#8329),(#8330,#8331),(#8332,#8333),(#8334,#8335),
(#8336,#8337),(#8338,#8339),(#8340,#8341),(#8342,#8343),(#8344,#8345),(#8346,
#8347),(#8348,#8349),(#8350,#8351),(#8352,#8353),(#8354,#8355),(#8356,#8357),
(#8358,#8359),(#8360,#8361),(#8362,#8363),(#8364,#8365),(#8366,#8367),(#8368,
#8369),(#8370,#8371),(#8372,#8373),(#8374,#8375),(#8376,#8377),(#8378,#8379),
(#8380,#8381),(#8382,#8383),(#8384,#8385),(#8386,#8387),(#8388,#8389),(#8390,
#8391),(#8392,#8393),(#8394,#8395),(#8396,#8397),(#8398,#8399),(#8400,#8401),
(#8402,#8403),(#8404,#8405),(#8406,#8407),(#8408,#8409),(#8410,#8411),(#8412,
#8413),(#8414,#8415),(#8416,#8417),(#8418,#8419),(#8420,#8421),(#8422,#8423),
(#8424,#8425)),.UNSPECIFIED.,.F.,.F.,.F.,(6,1,1,1,1,1,1,1,1,1,1,1,1,1,1,
1,1,1,1,1,1,1,1,1,1,1,1,1,1,1,1,1,1,1,1,1,1,1,1,1,1,1,1,1,1,1,1,1,1,1,1,
1,1,1,1,1,1,1,1,1,1,1,1,1,1,1,1,1,1,1,6),(2,2),(0.,0.0142857142857143,0.0285714285714286,
0.0428571428571429,0.0571428571428571,0.0714285714285714,0.0857142857142857,
0.1,0.114285714285714,0.128571428571429,0.142857142857143,0.157142857142857,
0.171428571428571,0.185714285714286,0.2,0.214285714285714,0.228571428571429,
0.242857142857143,0.257142857142857,0.271428571428571,0.285714285714286,
0.3,0.314285714285714,0.328571428571429,0.342857142857143,0.357142857142857,
0.371428571428571,0.385714285714286,0.4,0.414285714285714,0.428571428571429,
0.442857142857143,0.457142857142857,0.471428571428572,0.485714285714286,
0.5,0.514285714285714,0.528571428571429,0.542857142857143,0.557142857142857,
0.571428571428571,0.585714285714286,0.6,0.614285714285714,0.628571428571428,
0.642857142857142,0.657142857142857,0.671428571428571,0.685714285714285,
0.699999999999999,0.714285714285714,0.728571428571428,0.742857142857142,
0.757142857142856,0.771428571428571,0.785714285714285,0.799999999999999,
0.814285714285713,0.828571428571428,0.842857142857142,0.857142857142856,
0.87142857142857,0.885714285714284,0.899999999999999,0.914285714285713,
0.928571428571427,0.942857142857141,0.957142857142856,0.97142857142857,
0.985714285714284,1.),(0.,1.65),.UNSPECIFIED.);
#181=PLANE('',#3402);
#182=PLANE('',#3406);
#183=PLANE('',#3410);
#184=PLANE('',#3414);
#185=PLANE('',#3418);
#186=PLANE('',#3422);
#187=PLANE('',#3426);
#188=PLANE('',#3430);
#189=PLANE('',#3434);
#190=PLANE('',#3438);
#191=PLANE('',#3454);
#192=PLANE('',#3477);
#193=PLANE('',#3480);
#194=PLANE('',#3483);
#265=FACE_OUTER_BOUND('',#450,.T.);
#266=FACE_OUTER_BOUND('',#451,.T.);
#267=FACE_OUTER_BOUND('',#452,.T.);
#268=FACE_OUTER_BOUND('',#453,.T.);
#269=FACE_OUTER_BOUND('',#454,.T.);
#270=FACE_OUTER_BOUND('',#455,.T.);
#271=FACE_OUTER_BOUND('',#456,.T.);
#272=FACE_OUTER_BOUND('',#457,.T.);
#273=FACE_OUTER_BOUND('',#458,.T.);
#274=FACE_OUTER_BOUND('',#459,.T.);
#275=FACE_OUTER_BOUND('',#460,.T.);
#276=FACE_OUTER_BOUND('',#461,.T.);
#277=FACE_OUTER_BOUND('',#462,.T.);
#278=FACE_OUTER_BOUND('',#463,.T.);
#279=FACE_OUTER_BOUND('',#464,.T.);
#280=FACE_OUTER_BOUND('',#465,.T.);
#281=FACE_OUTER_BOUND('',#466,.T.);
#282=FACE_OUTER_BOUND('',#467,.T.);
#283=FACE_OUTER_BOUND('',#468,.T.);
#284=FACE_OUTER_BOUND('',#469,.T.);
#285=FACE_OUTER_BOUND('',#470,.T.);
#286=FACE_OUTER_BOUND('',#471,.T.);
#287=FACE_OUTER_BOUND('',#472,.T.);
#288=FACE_OUTER_BOUND('',#473,.T.);
#289=FACE_OUTER_BOUND('',#474,.T.);
#290=FACE_OUTER_BOUND('',#475,.T.);
#291=FACE_OUTER_BOUND('',#476,.T.);
#292=FACE_OUTER_BOUND('',#477,.T.);
#293=FACE_OUTER_BOUND('',#478,.T.);
#294=FACE_OUTER_BOUND('',#479,.T.);
#295=FACE_OUTER_BOUND('',#480,.T.);
#296=FACE_OUTER_BOUND('',#481,.T.);
#297=FACE_OUTER_BOUND('',#482,.T.);
#298=FACE_OUTER_BOUND('',#483,.T.);
#299=FACE_OUTER_BOUND('',#484,.T.);
#300=FACE_OUTER_BOUND('',#485,.T.);
#301=FACE_OUTER_BOUND('',#487,.T.);
#302=FACE_OUTER_BOUND('',#488,.T.);
#303=FACE_OUTER_BOUND('',#489,.T.);
#304=FACE_OUTER_BOUND('',#490,.T.);
#305=FACE_OUTER_BOUND('',#491,.T.);
#306=FACE_OUTER_BOUND('',#492,.T.);
#307=FACE_OUTER_BOUND('',#493,.T.);
#308=FACE_OUTER_BOUND('',#494,.T.);
#309=FACE_OUTER_BOUND('',#495,.T.);
#310=FACE_OUTER_BOUND('',#496,.T.);
#311=FACE_OUTER_BOUND('',#497,.T.);
#312=FACE_OUTER_BOUND('',#498,.T.);
#313=FACE_OUTER_BOUND('',#499,.T.);
#314=FACE_OUTER_BOUND('',#501,.T.);
#315=FACE_OUTER_BOUND('',#502,.T.);
#450=EDGE_LOOP('',(#2092,#2093,#2094,#2095));
#451=EDGE_LOOP('',(#2096,#2097,#2098,#2099));
#452=EDGE_LOOP('',(#2100,#2101,#2102,#2103));
#453=EDGE_LOOP('',(#2104,#2105,#2106,#2107));
#454=EDGE_LOOP('',(#2108,#2109,#2110,#2111));
#455=EDGE_LOOP('',(#2112,#2113,#2114,#2115));
#456=EDGE_LOOP('',(#2116,#2117,#2118,#2119));
#457=EDGE_LOOP('',(#2120,#2121,#2122,#2123));
#458=EDGE_LOOP('',(#2124,#2125,#2126,#2127));
#459=EDGE_LOOP('',(#2128,#2129,#2130,#2131));
#460=EDGE_LOOP('',(#2132,#2133,#2134,#2135));
#461=EDGE_LOOP('',(#2136,#2137,#2138,#2139));
#462=EDGE_LOOP('',(#2140,#2141,#2142,#2143));
#463=EDGE_LOOP('',(#2144,#2145,#2146,#2147));
#464=EDGE_LOOP('',(#2148,#2149,#2150,#2151));
#465=EDGE_LOOP('',(#2152,#2153,#2154,#2155));
#466=EDGE_LOOP('',(#2156,#2157,#2158,#2159));
#467=EDGE_LOOP('',(#2160,#2161,#2162,#2163));
#468=EDGE_LOOP('',(#2164,#2165,#2166,#2167));
#469=EDGE_LOOP('',(#2168,#2169,#2170,#2171));
#470=EDGE_LOOP('',(#2172,#2173,#2174,#2175));
#471=EDGE_LOOP('',(#2176,#2177,#2178,#2179));
#472=EDGE_LOOP('',(#2180,#2181,#2182,#2183));
#473=EDGE_LOOP('',(#2184,#2185,#2186,#2187));
#474=EDGE_LOOP('',(#2188,#2189,#2190,#2191));
#475=EDGE_LOOP('',(#2192,#2193,#2194,#2195));
#476=EDGE_LOOP('',(#2196,#2197,#2198,#2199));
#477=EDGE_LOOP('',(#2200,#2201,#2202,#2203));
#478=EDGE_LOOP('',(#2204,#2205,#2206,#2207));
#479=EDGE_LOOP('',(#2208,#2209,#2210,#2211));
#480=EDGE_LOOP('',(#2212,#2213,#2214,#2215));
#481=EDGE_LOOP('',(#2216,#2217,#2218,#2219));
#482=EDGE_LOOP('',(#2220,#2221,#2222,#2223));
#483=EDGE_LOOP('',(#2224,#2225,#2226,#2227));
#484=EDGE_LOOP('',(#2228,#2229,#2230,#2231));
#485=EDGE_LOOP('',(#2232,#2233,#2234,#2235,#2236,#2237,#2238,#2239,#2240,
#2241,#2242,#2243,#2244,#2245,#2246,#2247,#2248,#2249,#2250,#2251,#2252,
#2253,#2254,#2255,#2256,#2257,#2258,#2259,#2260,#2261,#2262,#2263,#2264,
#2265,#2266,#2267,#2268,#2269,#2270,#2271,#2272,#2273,#2274,#2275,#2276,
#2277,#2278,#2279));
#486=EDGE_LOOP('',(#2280));
#487=EDGE_LOOP('',(#2281,#2282,#2283,#2284));
#488=EDGE_LOOP('',(#2285,#2286,#2287,#2288));
#489=EDGE_LOOP('',(#2289,#2290,#2291,#2292));
#490=EDGE_LOOP('',(#2293,#2294,#2295,#2296));
#491=EDGE_LOOP('',(#2297,#2298,#2299,#2300));
#492=EDGE_LOOP('',(#2301,#2302,#2303,#2304));
#493=EDGE_LOOP('',(#2305,#2306,#2307,#2308));
#494=EDGE_LOOP('',(#2309,#2310,#2311,#2312));
#495=EDGE_LOOP('',(#2313,#2314,#2315,#2316));
#496=EDGE_LOOP('',(#2317,#2318,#2319,#2320));
#497=EDGE_LOOP('',(#2321,#2322,#2323,#2324));
#498=EDGE_LOOP('',(#2325,#2326,#2327,#2328));
#499=EDGE_LOOP('',(#2329,#2330,#2331,#2332,#2333,#2334,#2335,#2336,#2337,
#2338,#2339,#2340,#2341,#2342,#2343,#2344,#2345,#2346,#2347,#2348,#2349,
#2350,#2351,#2352,#2353,#2354,#2355,#2356,#2357,#2358,#2359,#2360,#2361,
#2362,#2363,#2364,#2365,#2366,#2367,#2368,#2369,#2370,#2371,#2372,#2373,
#2374,#2375,#2376));
#500=EDGE_LOOP('',(#2377));
#501=EDGE_LOOP('',(#2378,#2379,#2380,#2381));
#502=EDGE_LOOP('',(#2382,#2383,#2384,#2385));
#651=LINE('',#4653,#910);
#652=LINE('',#4656,#911);
#653=LINE('',#4659,#912);
#654=LINE('',#4661,#913);
#655=LINE('',#4662,#914);
#656=LINE('',#4668,#915);
#657=LINE('',#4671,#916);
#658=LINE('',#4674,#917);
#659=LINE('',#4676,#918);
#660=LINE('',#4677,#919);
#661=LINE('',#4683,#920);
#662=LINE('',#4686,#921);
#663=LINE('',#4689,#922);
#664=LINE('',#4691,#923);
#665=LINE('',#4692,#924);
#666=LINE('',#4698,#925);
#667=LINE('',#4701,#926);
#668=LINE('',#4704,#927);
#669=LINE('',#4706,#928);
#670=LINE('',#4707,#929);
#671=LINE('',#4713,#930);
#672=LINE('',#4716,#931);
#673=LINE('',#4719,#932);
#674=LINE('',#4721,#933);
#675=LINE('',#4722,#934);
#676=LINE('',#4728,#935);
#677=LINE('',#4731,#936);
#678=LINE('',#4734,#937);
#679=LINE('',#4736,#938);
#680=LINE('',#4737,#939);
#681=LINE('',#4743,#940);
#682=LINE('',#4746,#941);
#683=LINE('',#4749,#942);
#684=LINE('',#4751,#943);
#685=LINE('',#4752,#944);
#686=LINE('',#4758,#945);
#687=LINE('',#4761,#946);
#688=LINE('',#4764,#947);
#689=LINE('',#4766,#948);
#690=LINE('',#4767,#949);
#691=LINE('',#4773,#950);
#692=LINE('',#4776,#951);
#693=LINE('',#4779,#952);
#694=LINE('',#4781,#953);
#695=LINE('',#4782,#954);
#696=LINE('',#4788,#955);
#697=LINE('',#4791,#956);
#698=LINE('',#4794,#957);
#699=LINE('',#4796,#958);
#700=LINE('',#4797,#959);
#701=LINE('',#5100,#960);
#702=LINE('',#5106,#961);
#703=LINE('',#5709,#962);
#704=LINE('',#5715,#963);
#705=LINE('',#6318,#964);
#706=LINE('',#6324,#965);
#707=LINE('',#6927,#966);
#708=LINE('',#6933,#967);
#709=LINE('',#7536,#968);
#710=LINE('',#7542,#969);
#711=LINE('',#7852,#970);
#712=LINE('',#8008,#971);
#713=LINE('',#8018,#972);
#714=LINE('',#8030,#973);
#715=LINE('',#8033,#974);
#716=LINE('',#8034,#975);
#717=LINE('',#8037,#976);
#718=LINE('',#8040,#977);
#719=LINE('',#8043,#978);
#720=LINE('',#8044,#979);
#721=LINE('',#8271,#980);
#722=LINE('',#8275,#981);
#723=LINE('',#8506,#982);
#910=VECTOR('',#3735,10.);
#911=VECTOR('',#3738,10.);
#912=VECTOR('',#3741,10.);
#913=VECTOR('',#3742,10.);
#914=VECTOR('',#3743,10.);
#915=VECTOR('',#3748,10.);
#916=VECTOR('',#3751,10.);
#917=VECTOR('',#3754,10.);
#918=VECTOR('',#3755,10.);
#919=VECTOR('',#3756,10.);
#920=VECTOR('',#3761,10.);
#921=VECTOR('',#3764,10.);
#922=VECTOR('',#3767,10.);
#923=VECTOR('',#3768,10.);
#924=VECTOR('',#3769,10.);
#925=VECTOR('',#3774,10.);
#926=VECTOR('',#3777,10.);
#927=VECTOR('',#3780,10.);
#928=VECTOR('',#3781,10.);
#929=VECTOR('',#3782,10.);
#930=VECTOR('',#3787,10.);
#931=VECTOR('',#3790,10.);
#932=VECTOR('',#3793,10.);
#933=VECTOR('',#3794,10.);
#934=VECTOR('',#3795,10.);
#935=VECTOR('',#3800,10.);
#936=VECTOR('',#3803,10.);
#937=VECTOR('',#3806,10.);
#938=VECTOR('',#3807,10.);
#939=VECTOR('',#3808,10.);
#940=VECTOR('',#3813,10.);
#941=VECTOR('',#3816,10.);
#942=VECTOR('',#3819,10.);
#943=VECTOR('',#3820,10.);
#944=VECTOR('',#3821,10.);
#945=VECTOR('',#3826,10.);
#946=VECTOR('',#3829,10.);
#947=VECTOR('',#3832,10.);
#948=VECTOR('',#3833,10.);
#949=VECTOR('',#3834,10.);
#950=VECTOR('',#3839,10.);
#951=VECTOR('',#3842,10.);
#952=VECTOR('',#3845,10.);
#953=VECTOR('',#3846,10.);
#954=VECTOR('',#3847,10.);
#955=VECTOR('',#3852,10.);
#956=VECTOR('',#3855,10.);
#957=VECTOR('',#3858,10.);
#958=VECTOR('',#3859,10.);
#959=VECTOR('',#3860,10.);
#960=VECTOR('',#3861,10.);
#961=VECTOR('',#3868,10.);
#962=VECTOR('',#3869,10.);
#963=VECTOR('',#3876,10.);
#964=VECTOR('',#3877,10.);
#965=VECTOR('',#3884,10.);
#966=VECTOR('',#3885,10.);
#967=VECTOR('',#3892,10.);
#968=VECTOR('',#3893,10.);
#969=VECTOR('',#3900,10.);
#970=VECTOR('',#3913,10.);
#971=VECTOR('',#3916,10.);
#972=VECTOR('',#3929,10.);
#973=VECTOR('',#3950,10.);
#974=VECTOR('',#3953,10.);
#975=VECTOR('',#3954,10.);
#976=VECTOR('',#3957,10.);
#977=VECTOR('',#3960,10.);
#978=VECTOR('',#3963,10.);
#979=VECTOR('',#3964,10.);
#980=VECTOR('',#3965,10.);
#981=VECTOR('',#3970,10.);
#982=VECTOR('',#3979,5.);
#1169=CIRCLE('',#3400,1.);
#1170=CIRCLE('',#3401,1.);
#1171=CIRCLE('',#3404,1.);
#1172=CIRCLE('',#3405,1.);
#1173=CIRCLE('',#3408,1.);
#1174=CIRCLE('',#3409,1.);
#1175=CIRCLE('',#3412,1.);
#1176=CIRCLE('',#3413,1.);
#1177=CIRCLE('',#3416,1.);
#1178=CIRCLE('',#3417,1.);
#1179=CIRCLE('',#3420,1.);
#1180=CIRCLE('',#3421,1.);
#1181=CIRCLE('',#3424,1.);
#1182=CIRCLE('',#3425,1.);
#1183=CIRCLE('',#3428,1.);
#1184=CIRCLE('',#3429,1.);
#1185=CIRCLE('',#3432,1.);
#1186=CIRCLE('',#3433,1.);
#1187=CIRCLE('',#3436,1.);
#1188=CIRCLE('',#3437,1.);
#1189=CIRCLE('',#3440,11.9999999999996);
#1190=CIRCLE('',#3441,11.9999999999996);
#1191=CIRCLE('',#3443,11.9999999999996);
#1192=CIRCLE('',#3444,11.9999999999996);
#1193=CIRCLE('',#3446,11.9999999999996);
#1194=CIRCLE('',#3447,11.9999999999996);
#1195=CIRCLE('',#3449,11.9999999999996);
#1196=CIRCLE('',#3450,11.9999999999996);
#1197=CIRCLE('',#3452,11.9999999999996);
#1198=CIRCLE('',#3453,11.9999999999996);
#1199=CIRCLE('',#3455,5.529);
#1200=CIRCLE('',#3456,5.529);
#1201=CIRCLE('',#3457,5.529);
#1202=CIRCLE('',#3458,5.529);
#1203=CIRCLE('',#3459,1.);
#1204=CIRCLE('',#3460,11.9999999999996);
#1205=CIRCLE('',#3461,1.);
#1206=CIRCLE('',#3462,5.529);
#1207=CIRCLE('',#3463,5.529);
#1208=CIRCLE('',#3464,5.);
#1209=CIRCLE('',#3466,5.529);
#1210=CIRCLE('',#3468,5.529);
#1211=CIRCLE('',#3470,5.529);
#1212=CIRCLE('',#3472,5.529);
#1213=CIRCLE('',#3474,5.529);
#1214=CIRCLE('',#3476,1.);
#1215=CIRCLE('',#3479,1.);
#1216=CIRCLE('',#3482,11.9999999999996);
#1217=CIRCLE('',#3484,5.529);
#1218=CIRCLE('',#3485,5.);
#1319=VERTEX_POINT('',#4649);
#1320=VERTEX_POINT('',#4650);
#1321=VERTEX_POINT('',#4652);
#1322=VERTEX_POINT('',#4654);
#1323=VERTEX_POINT('',#4658);
#1324=VERTEX_POINT('',#4660);
#1325=VERTEX_POINT('',#4664);
#1326=VERTEX_POINT('',#4665);
#1327=VERTEX_POINT('',#4667);
#1328=VERTEX_POINT('',#4669);
#1329=VERTEX_POINT('',#4673);
#1330=VERTEX_POINT('',#4675);
#1331=VERTEX_POINT('',#4679);
#1332=VERTEX_POINT('',#4680);
#1333=VERTEX_POINT('',#4682);
#1334=VERTEX_POINT('',#4684);
#1335=VERTEX_POINT('',#4688);
#1336=VERTEX_POINT('',#4690);
#1337=VERTEX_POINT('',#4694);
#1338=VERTEX_POINT('',#4695);
#1339=VERTEX_POINT('',#4697);
#1340=VERTEX_POINT('',#4699);
#1341=VERTEX_POINT('',#4703);
#1342=VERTEX_POINT('',#4705);
#1343=VERTEX_POINT('',#4709);
#1344=VERTEX_POINT('',#4710);
#1345=VERTEX_POINT('',#4712);
#1346=VERTEX_POINT('',#4714);
#1347=VERTEX_POINT('',#4718);
#1348=VERTEX_POINT('',#4720);
#1349=VERTEX_POINT('',#4724);
#1350=VERTEX_POINT('',#4725);
#1351=VERTEX_POINT('',#4727);
#1352=VERTEX_POINT('',#4729);
#1353=VERTEX_POINT('',#4733);
#1354=VERTEX_POINT('',#4735);
#1355=VERTEX_POINT('',#4739);
#1356=VERTEX_POINT('',#4740);
#1357=VERTEX_POINT('',#4742);
#1358=VERTEX_POINT('',#4744);
#1359=VERTEX_POINT('',#4748);
#1360=VERTEX_POINT('',#4750);
#1361=VERTEX_POINT('',#4754);
#1362=VERTEX_POINT('',#4755);
#1363=VERTEX_POINT('',#4757);
#1364=VERTEX_POINT('',#4759);
#1365=VERTEX_POINT('',#4763);
#1366=VERTEX_POINT('',#4765);
#1367=VERTEX_POINT('',#4769);
#1368=VERTEX_POINT('',#4770);
#1369=VERTEX_POINT('',#4772);
#1370=VERTEX_POINT('',#4774);
#1371=VERTEX_POINT('',#4778);
#1372=VERTEX_POINT('',#4780);
#1373=VERTEX_POINT('',#4784);
#1374=VERTEX_POINT('',#4785);
#1375=VERTEX_POINT('',#4787);
#1376=VERTEX_POINT('',#4789);
#1377=VERTEX_POINT('',#4793);
#1378=VERTEX_POINT('',#4795);
#1379=VERTEX_POINT('',#4948);
#1380=VERTEX_POINT('',#5024);
#1381=VERTEX_POINT('',#5102);
#1382=VERTEX_POINT('',#5104);
#1383=VERTEX_POINT('',#5557);
#1384=VERTEX_POINT('',#5633);
#1385=VERTEX_POINT('',#5711);
#1386=VERTEX_POINT('',#5713);
#1387=VERTEX_POINT('',#6166);
#1388=VERTEX_POINT('',#6242);
#1389=VERTEX_POINT('',#6320);
#1390=VERTEX_POINT('',#6322);
#1391=VERTEX_POINT('',#6775);
#1392=VERTEX_POINT('',#6851);
#1393=VERTEX_POINT('',#6929);
#1394=VERTEX_POINT('',#6931);
#1395=VERTEX_POINT('',#7384);
#1396=VERTEX_POINT('',#7460);
#1397=VERTEX_POINT('',#7538);
#1398=VERTEX_POINT('',#7540);
#1399=VERTEX_POINT('',#7847);
#1400=VERTEX_POINT('',#7849);
#1401=VERTEX_POINT('',#7851);
#1402=VERTEX_POINT('',#7853);
#1403=VERTEX_POINT('',#7929);
#1404=VERTEX_POINT('',#7931);
#1405=VERTEX_POINT('',#8007);
#1406=VERTEX_POINT('',#8009);
#1407=VERTEX_POINT('',#8013);
#1408=VERTEX_POINT('',#8016);
#1409=VERTEX_POINT('',#8028);
#1410=VERTEX_POINT('',#8032);
#1411=VERTEX_POINT('',#8036);
#1412=VERTEX_POINT('',#8038);
#1413=VERTEX_POINT('',#8042);
#1414=VERTEX_POINT('',#8195);
#1415=VERTEX_POINT('',#8273);
#1416=VERTEX_POINT('',#8503);
#1625=EDGE_CURVE('',#1319,#1320,#1169,.F.);
#1626=EDGE_CURVE('',#1320,#1321,#651,.T.);
#1627=EDGE_CURVE('',#1321,#1322,#1170,.T.);
#1628=EDGE_CURVE('',#1322,#1319,#652,.T.);
#1629=EDGE_CURVE('',#1323,#1320,#653,.T.);
#1630=EDGE_CURVE('',#1324,#1323,#654,.T.);
#1631=EDGE_CURVE('',#1321,#1324,#655,.F.);
#1632=EDGE_CURVE('',#1325,#1326,#1171,.T.);
#1633=EDGE_CURVE('',#1326,#1327,#656,.T.);
#1634=EDGE_CURVE('',#1327,#1328,#1172,.F.);
#1635=EDGE_CURVE('',#1328,#1325,#657,.T.);
#1636=EDGE_CURVE('',#1326,#1329,#658,.T.);
#1637=EDGE_CURVE('',#1329,#1330,#659,.T.);
#1638=EDGE_CURVE('',#1327,#1330,#660,.T.);
#1639=EDGE_CURVE('',#1331,#1332,#1173,.F.);
#1640=EDGE_CURVE('',#1332,#1333,#661,.T.);
#1641=EDGE_CURVE('',#1333,#1334,#1174,.T.);
#1642=EDGE_CURVE('',#1334,#1331,#662,.T.);
#1643=EDGE_CURVE('',#1335,#1332,#663,.T.);
#1644=EDGE_CURVE('',#1336,#1335,#664,.T.);
#1645=EDGE_CURVE('',#1333,#1336,#665,.F.);
#1646=EDGE_CURVE('',#1337,#1338,#1175,.T.);
#1647=EDGE_CURVE('',#1338,#1339,#666,.T.);
#1648=EDGE_CURVE('',#1339,#1340,#1176,.F.);
#1649=EDGE_CURVE('',#1340,#1337,#667,.T.);
#1650=EDGE_CURVE('',#1338,#1341,#668,.T.);
#1651=EDGE_CURVE('',#1341,#1342,#669,.T.);
#1652=EDGE_CURVE('',#1339,#1342,#670,.T.);
#1653=EDGE_CURVE('',#1343,#1344,#1177,.F.);
#1654=EDGE_CURVE('',#1344,#1345,#671,.T.);
#1655=EDGE_CURVE('',#1345,#1346,#1178,.T.);
#1656=EDGE_CURVE('',#1346,#1343,#672,.T.);
#1657=EDGE_CURVE('',#1347,#1344,#673,.T.);
#1658=EDGE_CURVE('',#1348,#1347,#674,.T.);
#1659=EDGE_CURVE('',#1345,#1348,#675,.F.);
#1660=EDGE_CURVE('',#1349,#1350,#1179,.T.);
#1661=EDGE_CURVE('',#1350,#1351,#676,.T.);
#1662=EDGE_CURVE('',#1351,#1352,#1180,.F.);
#1663=EDGE_CURVE('',#1352,#1349,#677,.T.);
#1664=EDGE_CURVE('',#1350,#1353,#678,.T.);
#1665=EDGE_CURVE('',#1353,#1354,#679,.T.);
#1666=EDGE_CURVE('',#1351,#1354,#680,.T.);
#1667=EDGE_CURVE('',#1355,#1356,#1181,.F.);
#1668=EDGE_CURVE('',#1356,#1357,#681,.T.);
#1669=EDGE_CURVE('',#1357,#1358,#1182,.T.);
#1670=EDGE_CURVE('',#1358,#1355,#682,.T.);
#1671=EDGE_CURVE('',#1359,#1356,#683,.T.);
#1672=EDGE_CURVE('',#1360,#1359,#684,.T.);
#1673=EDGE_CURVE('',#1357,#1360,#685,.F.);
#1674=EDGE_CURVE('',#1361,#1362,#1183,.T.);
#1675=EDGE_CURVE('',#1362,#1363,#686,.T.);
#1676=EDGE_CURVE('',#1363,#1364,#1184,.F.);
#1677=EDGE_CURVE('',#1364,#1361,#687,.T.);
#1678=EDGE_CURVE('',#1362,#1365,#688,.T.);
#1679=EDGE_CURVE('',#1365,#1366,#689,.T.);
#1680=EDGE_CURVE('',#1363,#1366,#690,.T.);
#1681=EDGE_CURVE('',#1367,#1368,#1185,.F.);
#1682=EDGE_CURVE('',#1368,#1369,#691,.T.);
#1683=EDGE_CURVE('',#1369,#1370,#1186,.T.);
#1684=EDGE_CURVE('',#1370,#1367,#692,.T.);
#1685=EDGE_CURVE('',#1371,#1368,#693,.T.);
#1686=EDGE_CURVE('',#1372,#1371,#694,.T.);
#1687=EDGE_CURVE('',#1369,#1372,#695,.F.);
#1688=EDGE_CURVE('',#1373,#1374,#1187,.T.);
#1689=EDGE_CURVE('',#1374,#1375,#696,.T.);
#1690=EDGE_CURVE('',#1375,#1376,#1188,.F.);
#1691=EDGE_CURVE('',#1376,#1373,#697,.T.);
#1692=EDGE_CURVE('',#1374,#1377,#698,.T.);
#1693=EDGE_CURVE('',#1377,#1378,#699,.T.);
#1694=EDGE_CURVE('',#1375,#1378,#700,.T.);
#1695=EDGE_CURVE('',#1324,#1379,#99,.F.);
#1696=EDGE_CURVE('',#1380,#1323,#100,.T.);
#1697=EDGE_CURVE('',#1379,#1380,#701,.T.);
#1698=EDGE_CURVE('',#1381,#1379,#1189,.T.);
#1699=EDGE_CURVE('',#1382,#1380,#1190,.T.);
#1700=EDGE_CURVE('',#1381,#1382,#702,.T.);
#1701=EDGE_CURVE('',#1329,#1381,#101,.T.);
#1702=EDGE_CURVE('',#1330,#1382,#102,.T.);
#1703=EDGE_CURVE('',#1336,#1383,#103,.F.);
#1704=EDGE_CURVE('',#1384,#1335,#104,.T.);
#1705=EDGE_CURVE('',#1383,#1384,#703,.T.);
#1706=EDGE_CURVE('',#1385,#1383,#1191,.T.);
#1707=EDGE_CURVE('',#1386,#1384,#1192,.T.);
#1708=EDGE_CURVE('',#1385,#1386,#704,.T.);
#1709=EDGE_CURVE('',#1341,#1385,#105,.T.);
#1710=EDGE_CURVE('',#1342,#1386,#106,.T.);
#1711=EDGE_CURVE('',#1348,#1387,#107,.F.);
#1712=EDGE_CURVE('',#1388,#1347,#108,.T.);
#1713=EDGE_CURVE('',#1387,#1388,#705,.T.);
#1714=EDGE_CURVE('',#1389,#1387,#1193,.T.);
#1715=EDGE_CURVE('',#1390,#1388,#1194,.T.);
#1716=EDGE_CURVE('',#1389,#1390,#706,.T.);
#1717=EDGE_CURVE('',#1353,#1389,#109,.T.);
#1718=EDGE_CURVE('',#1354,#1390,#110,.T.);
#1719=EDGE_CURVE('',#1360,#1391,#111,.F.);
#1720=EDGE_CURVE('',#1392,#1359,#112,.T.);
#1721=EDGE_CURVE('',#1391,#1392,#707,.T.);
#1722=EDGE_CURVE('',#1393,#1391,#1195,.T.);
#1723=EDGE_CURVE('',#1394,#1392,#1196,.T.);
#1724=EDGE_CURVE('',#1393,#1394,#708,.T.);
#1725=EDGE_CURVE('',#1365,#1393,#113,.T.);
#1726=EDGE_CURVE('',#1366,#1394,#114,.T.);
#1727=EDGE_CURVE('',#1372,#1395,#115,.F.);
#1728=EDGE_CURVE('',#1396,#1371,#116,.T.);
#1729=EDGE_CURVE('',#1395,#1396,#709,.T.);
#1730=EDGE_CURVE('',#1397,#1395,#1197,.T.);
#1731=EDGE_CURVE('',#1398,#1396,#1198,.T.);
#1732=EDGE_CURVE('',#1397,#1398,#710,.T.);
#1733=EDGE_CURVE('',#1377,#1397,#117,.T.);
#1734=EDGE_CURVE('',#1378,#1398,#118,.T.);
#1735=EDGE_CURVE('',#1346,#1337,#1199,.T.);
#1736=EDGE_CURVE('',#1358,#1349,#1200,.T.);
#1737=EDGE_CURVE('',#1370,#1361,#1201,.T.);
#1738=EDGE_CURVE('',#1399,#1373,#1202,.T.);
#1739=EDGE_CURVE('',#1400,#1399,#1203,.T.);
#1740=EDGE_CURVE('',#1400,#1401,#711,.F.);
#1741=EDGE_CURVE('',#1401,#1402,#119,.F.);
#1742=EDGE_CURVE('',#1403,#1402,#1204,.T.);
#1743=EDGE_CURVE('',#1404,#1403,#120,.T.);
#1744=EDGE_CURVE('',#1405,#1404,#712,.T.);
#1745=EDGE_CURVE('',#1406,#1405,#1205,.T.);
#1746=EDGE_CURVE('',#1322,#1406,#1206,.T.);
#1747=EDGE_CURVE('',#1334,#1325,#1207,.T.);
#1748=EDGE_CURVE('',#1407,#1407,#1208,.T.);
#1749=EDGE_CURVE('',#1408,#1376,#1209,.T.);
#1750=EDGE_CURVE('',#1399,#1408,#713,.T.);
#1751=EDGE_CURVE('',#1367,#1364,#1210,.T.);
#1752=EDGE_CURVE('',#1355,#1352,#1211,.T.);
#1753=EDGE_CURVE('',#1343,#1340,#1212,.T.);
#1754=EDGE_CURVE('',#1331,#1328,#1213,.T.);
#1755=EDGE_CURVE('',#1408,#1409,#1214,.F.);
#1756=EDGE_CURVE('',#1409,#1400,#714,.T.);
#1757=EDGE_CURVE('',#1410,#1409,#715,.T.);
#1758=EDGE_CURVE('',#1401,#1410,#716,.T.);
#1759=EDGE_CURVE('',#1405,#1411,#717,.T.);
#1760=EDGE_CURVE('',#1411,#1412,#1215,.F.);
#1761=EDGE_CURVE('',#1412,#1406,#718,.T.);
#1762=EDGE_CURVE('',#1404,#1413,#719,.T.);
#1763=EDGE_CURVE('',#1411,#1413,#720,.T.);
#1764=EDGE_CURVE('',#1414,#1410,#121,.T.);
#1765=EDGE_CURVE('',#1402,#1414,#721,.T.);
#1766=EDGE_CURVE('',#1415,#1414,#1216,.T.);
#1767=EDGE_CURVE('',#1403,#1415,#722,.T.);
#1768=EDGE_CURVE('',#1413,#1415,#122,.T.);
#1769=EDGE_CURVE('',#1319,#1412,#1217,.T.);
#1770=EDGE_CURVE('',#1416,#1416,#1218,.T.);
#1771=EDGE_CURVE('',#1407,#1416,#723,.T.);
#2092=ORIENTED_EDGE('',*,*,#1625,.T.);
#2093=ORIENTED_EDGE('',*,*,#1626,.T.);
#2094=ORIENTED_EDGE('',*,*,#1627,.T.);
#2095=ORIENTED_EDGE('',*,*,#1628,.T.);
#2096=ORIENTED_EDGE('',*,*,#1626,.F.);
#2097=ORIENTED_EDGE('',*,*,#1629,.F.);
#2098=ORIENTED_EDGE('',*,*,#1630,.F.);
#2099=ORIENTED_EDGE('',*,*,#1631,.F.);
#2100=ORIENTED_EDGE('',*,*,#1632,.T.);
#2101=ORIENTED_EDGE('',*,*,#1633,.T.);
#2102=ORIENTED_EDGE('',*,*,#1634,.T.);
#2103=ORIENTED_EDGE('',*,*,#1635,.T.);
#2104=ORIENTED_EDGE('',*,*,#1633,.F.);
#2105=ORIENTED_EDGE('',*,*,#1636,.T.);
#2106=ORIENTED_EDGE('',*,*,#1637,.T.);
#2107=ORIENTED_EDGE('',*,*,#1638,.F.);
#2108=ORIENTED_EDGE('',*,*,#1639,.T.);
#2109=ORIENTED_EDGE('',*,*,#1640,.T.);
#2110=ORIENTED_EDGE('',*,*,#1641,.T.);
#2111=ORIENTED_EDGE('',*,*,#1642,.T.);
#2112=ORIENTED_EDGE('',*,*,#1640,.F.);
#2113=ORIENTED_EDGE('',*,*,#1643,.F.);
#2114=ORIENTED_EDGE('',*,*,#1644,.F.);
#2115=ORIENTED_EDGE('',*,*,#1645,.F.);
#2116=ORIENTED_EDGE('',*,*,#1646,.T.);
#2117=ORIENTED_EDGE('',*,*,#1647,.T.);
#2118=ORIENTED_EDGE('',*,*,#1648,.T.);
#2119=ORIENTED_EDGE('',*,*,#1649,.T.);
#2120=ORIENTED_EDGE('',*,*,#1647,.F.);
#2121=ORIENTED_EDGE('',*,*,#1650,.T.);
#2122=ORIENTED_EDGE('',*,*,#1651,.T.);
#2123=ORIENTED_EDGE('',*,*,#1652,.F.);
#2124=ORIENTED_EDGE('',*,*,#1653,.T.);
#2125=ORIENTED_EDGE('',*,*,#1654,.T.);
#2126=ORIENTED_EDGE('',*,*,#1655,.T.);
#2127=ORIENTED_EDGE('',*,*,#1656,.T.);
#2128=ORIENTED_EDGE('',*,*,#1654,.F.);
#2129=ORIENTED_EDGE('',*,*,#1657,.F.);
#2130=ORIENTED_EDGE('',*,*,#1658,.F.);
#2131=ORIENTED_EDGE('',*,*,#1659,.F.);
#2132=ORIENTED_EDGE('',*,*,#1660,.T.);
#2133=ORIENTED_EDGE('',*,*,#1661,.T.);
#2134=ORIENTED_EDGE('',*,*,#1662,.T.);
#2135=ORIENTED_EDGE('',*,*,#1663,.T.);
#2136=ORIENTED_EDGE('',*,*,#1661,.F.);
#2137=ORIENTED_EDGE('',*,*,#1664,.T.);
#2138=ORIENTED_EDGE('',*,*,#1665,.T.);
#2139=ORIENTED_EDGE('',*,*,#1666,.F.);
#2140=ORIENTED_EDGE('',*,*,#1667,.T.);
#2141=ORIENTED_EDGE('',*,*,#1668,.T.);
#2142=ORIENTED_EDGE('',*,*,#1669,.T.);
#2143=ORIENTED_EDGE('',*,*,#1670,.T.);
#2144=ORIENTED_EDGE('',*,*,#1668,.F.);
#2145=ORIENTED_EDGE('',*,*,#1671,.F.);
#2146=ORIENTED_EDGE('',*,*,#1672,.F.);
#2147=ORIENTED_EDGE('',*,*,#1673,.F.);
#2148=ORIENTED_EDGE('',*,*,#1674,.T.);
#2149=ORIENTED_EDGE('',*,*,#1675,.T.);
#2150=ORIENTED_EDGE('',*,*,#1676,.T.);
#2151=ORIENTED_EDGE('',*,*,#1677,.T.);
#2152=ORIENTED_EDGE('',*,*,#1675,.F.);
#2153=ORIENTED_EDGE('',*,*,#1678,.T.);
#2154=ORIENTED_EDGE('',*,*,#1679,.T.);
#2155=ORIENTED_EDGE('',*,*,#1680,.F.);
#2156=ORIENTED_EDGE('',*,*,#1681,.T.);
#2157=ORIENTED_EDGE('',*,*,#1682,.T.);
#2158=ORIENTED_EDGE('',*,*,#1683,.T.);
#2159=ORIENTED_EDGE('',*,*,#1684,.T.);
#2160=ORIENTED_EDGE('',*,*,#1682,.F.);
#2161=ORIENTED_EDGE('',*,*,#1685,.F.);
#2162=ORIENTED_EDGE('',*,*,#1686,.F.);
#2163=ORIENTED_EDGE('',*,*,#1687,.F.);
#2164=ORIENTED_EDGE('',*,*,#1688,.T.);
#2165=ORIENTED_EDGE('',*,*,#1689,.T.);
#2166=ORIENTED_EDGE('',*,*,#1690,.T.);
#2167=ORIENTED_EDGE('',*,*,#1691,.T.);
#2168=ORIENTED_EDGE('',*,*,#1689,.F.);
#2169=ORIENTED_EDGE('',*,*,#1692,.T.);
#2170=ORIENTED_EDGE('',*,*,#1693,.T.);
#2171=ORIENTED_EDGE('',*,*,#1694,.F.);
#2172=ORIENTED_EDGE('',*,*,#1695,.F.);
#2173=ORIENTED_EDGE('',*,*,#1630,.T.);
#2174=ORIENTED_EDGE('',*,*,#1696,.F.);
#2175=ORIENTED_EDGE('',*,*,#1697,.F.);
#2176=ORIENTED_EDGE('',*,*,#1698,.T.);
#2177=ORIENTED_EDGE('',*,*,#1697,.T.);
#2178=ORIENTED_EDGE('',*,*,#1699,.F.);
#2179=ORIENTED_EDGE('',*,*,#1700,.F.);
#2180=ORIENTED_EDGE('',*,*,#1701,.T.);
#2181=ORIENTED_EDGE('',*,*,#1700,.T.);
#2182=ORIENTED_EDGE('',*,*,#1702,.F.);
#2183=ORIENTED_EDGE('',*,*,#1637,.F.);
#2184=ORIENTED_EDGE('',*,*,#1703,.F.);
#2185=ORIENTED_EDGE('',*,*,#1644,.T.);
#2186=ORIENTED_EDGE('',*,*,#1704,.F.);
#2187=ORIENTED_EDGE('',*,*,#1705,.F.);
#2188=ORIENTED_EDGE('',*,*,#1706,.T.);
#2189=ORIENTED_EDGE('',*,*,#1705,.T.);
#2190=ORIENTED_EDGE('',*,*,#1707,.F.);
#2191=ORIENTED_EDGE('',*,*,#1708,.F.);
#2192=ORIENTED_EDGE('',*,*,#1709,.T.);
#2193=ORIENTED_EDGE('',*,*,#1708,.T.);
#2194=ORIENTED_EDGE('',*,*,#1710,.F.);
#2195=ORIENTED_EDGE('',*,*,#1651,.F.);
#2196=ORIENTED_EDGE('',*,*,#1711,.F.);
#2197=ORIENTED_EDGE('',*,*,#1658,.T.);
#2198=ORIENTED_EDGE('',*,*,#1712,.F.);
#2199=ORIENTED_EDGE('',*,*,#1713,.F.);
#2200=ORIENTED_EDGE('',*,*,#1714,.T.);
#2201=ORIENTED_EDGE('',*,*,#1713,.T.);
#2202=ORIENTED_EDGE('',*,*,#1715,.F.);
#2203=ORIENTED_EDGE('',*,*,#1716,.F.);
#2204=ORIENTED_EDGE('',*,*,#1717,.T.);
#2205=ORIENTED_EDGE('',*,*,#1716,.T.);
#2206=ORIENTED_EDGE('',*,*,#1718,.F.);
#2207=ORIENTED_EDGE('',*,*,#1665,.F.);
#2208=ORIENTED_EDGE('',*,*,#1719,.F.);
#2209=ORIENTED_EDGE('',*,*,#1672,.T.);
#2210=ORIENTED_EDGE('',*,*,#1720,.F.);
#2211=ORIENTED_EDGE('',*,*,#1721,.F.);
#2212=ORIENTED_EDGE('',*,*,#1722,.T.);
#2213=ORIENTED_EDGE('',*,*,#1721,.T.);
#2214=ORIENTED_EDGE('',*,*,#1723,.F.);
#2215=ORIENTED_EDGE('',*,*,#1724,.F.);
#2216=ORIENTED_EDGE('',*,*,#1725,.T.);
#2217=ORIENTED_EDGE('',*,*,#1724,.T.);
#2218=ORIENTED_EDGE('',*,*,#1726,.F.);
#2219=ORIENTED_EDGE('',*,*,#1679,.F.);
#2220=ORIENTED_EDGE('',*,*,#1727,.F.);
#2221=ORIENTED_EDGE('',*,*,#1686,.T.);
#2222=ORIENTED_EDGE('',*,*,#1728,.F.);
#2223=ORIENTED_EDGE('',*,*,#1729,.F.);
#2224=ORIENTED_EDGE('',*,*,#1730,.T.);
#2225=ORIENTED_EDGE('',*,*,#1729,.T.);
#2226=ORIENTED_EDGE('',*,*,#1731,.F.);
#2227=ORIENTED_EDGE('',*,*,#1732,.F.);
#2228=ORIENTED_EDGE('',*,*,#1733,.T.);
#2229=ORIENTED_EDGE('',*,*,#1732,.T.);
#2230=ORIENTED_EDGE('',*,*,#1734,.F.);
#2231=ORIENTED_EDGE('',*,*,#1693,.F.);
#2232=ORIENTED_EDGE('',*,*,#1641,.F.);
#2233=ORIENTED_EDGE('',*,*,#1645,.T.);
#2234=ORIENTED_EDGE('',*,*,#1703,.T.);
#2235=ORIENTED_EDGE('',*,*,#1706,.F.);
#2236=ORIENTED_EDGE('',*,*,#1709,.F.);
#2237=ORIENTED_EDGE('',*,*,#1650,.F.);
#2238=ORIENTED_EDGE('',*,*,#1646,.F.);
#2239=ORIENTED_EDGE('',*,*,#1735,.F.);
#2240=ORIENTED_EDGE('',*,*,#1655,.F.);
#2241=ORIENTED_EDGE('',*,*,#1659,.T.);
#2242=ORIENTED_EDGE('',*,*,#1711,.T.);
#2243=ORIENTED_EDGE('',*,*,#1714,.F.);
#2244=ORIENTED_EDGE('',*,*,#1717,.F.);
#2245=ORIENTED_EDGE('',*,*,#1664,.F.);
#2246=ORIENTED_EDGE('',*,*,#1660,.F.);
#2247=ORIENTED_EDGE('',*,*,#1736,.F.);
#2248=ORIENTED_EDGE('',*,*,#1669,.F.);
#2249=ORIENTED_EDGE('',*,*,#1673,.T.);
#2250=ORIENTED_EDGE('',*,*,#1719,.T.);
#2251=ORIENTED_EDGE('',*,*,#1722,.F.);
#2252=ORIENTED_EDGE('',*,*,#1725,.F.);
#2253=ORIENTED_EDGE('',*,*,#1678,.F.);
#2254=ORIENTED_EDGE('',*,*,#1674,.F.);
#2255=ORIENTED_EDGE('',*,*,#1737,.F.);
#2256=ORIENTED_EDGE('',*,*,#1683,.F.);
#2257=ORIENTED_EDGE('',*,*,#1687,.T.);
#2258=ORIENTED_EDGE('',*,*,#1727,.T.);
#2259=ORIENTED_EDGE('',*,*,#1730,.F.);
#2260=ORIENTED_EDGE('',*,*,#1733,.F.);
#2261=ORIENTED_EDGE('',*,*,#1692,.F.);
#2262=ORIENTED_EDGE('',*,*,#1688,.F.);
#2263=ORIENTED_EDGE('',*,*,#1738,.F.);
#2264=ORIENTED_EDGE('',*,*,#1739,.F.);
#2265=ORIENTED_EDGE('',*,*,#1740,.T.);
#2266=ORIENTED_EDGE('',*,*,#1741,.T.);
#2267=ORIENTED_EDGE('',*,*,#1742,.F.);
#2268=ORIENTED_EDGE('',*,*,#1743,.F.);
#2269=ORIENTED_EDGE('',*,*,#1744,.F.);
#2270=ORIENTED_EDGE('',*,*,#1745,.F.);
#2271=ORIENTED_EDGE('',*,*,#1746,.F.);
#2272=ORIENTED_EDGE('',*,*,#1627,.F.);
#2273=ORIENTED_EDGE('',*,*,#1631,.T.);
#2274=ORIENTED_EDGE('',*,*,#1695,.T.);
#2275=ORIENTED_EDGE('',*,*,#1698,.F.);
#2276=ORIENTED_EDGE('',*,*,#1701,.F.);
#2277=ORIENTED_EDGE('',*,*,#1636,.F.);
#2278=ORIENTED_EDGE('',*,*,#1632,.F.);
#2279=ORIENTED_EDGE('',*,*,#1747,.F.);
#2280=ORIENTED_EDGE('',*,*,#1748,.F.);
#2281=ORIENTED_EDGE('',*,*,#1691,.F.);
#2282=ORIENTED_EDGE('',*,*,#1749,.F.);
#2283=ORIENTED_EDGE('',*,*,#1750,.F.);
#2284=ORIENTED_EDGE('',*,*,#1738,.T.);
#2285=ORIENTED_EDGE('',*,*,#1677,.F.);
#2286=ORIENTED_EDGE('',*,*,#1751,.F.);
#2287=ORIENTED_EDGE('',*,*,#1684,.F.);
#2288=ORIENTED_EDGE('',*,*,#1737,.T.);
#2289=ORIENTED_EDGE('',*,*,#1663,.F.);
#2290=ORIENTED_EDGE('',*,*,#1752,.F.);
#2291=ORIENTED_EDGE('',*,*,#1670,.F.);
#2292=ORIENTED_EDGE('',*,*,#1736,.T.);
#2293=ORIENTED_EDGE('',*,*,#1649,.F.);
#2294=ORIENTED_EDGE('',*,*,#1753,.F.);
#2295=ORIENTED_EDGE('',*,*,#1656,.F.);
#2296=ORIENTED_EDGE('',*,*,#1735,.T.);
#2297=ORIENTED_EDGE('',*,*,#1635,.F.);
#2298=ORIENTED_EDGE('',*,*,#1754,.F.);
#2299=ORIENTED_EDGE('',*,*,#1642,.F.);
#2300=ORIENTED_EDGE('',*,*,#1747,.T.);
#2301=ORIENTED_EDGE('',*,*,#1755,.T.);
#2302=ORIENTED_EDGE('',*,*,#1756,.T.);
#2303=ORIENTED_EDGE('',*,*,#1739,.T.);
#2304=ORIENTED_EDGE('',*,*,#1750,.T.);
#2305=ORIENTED_EDGE('',*,*,#1756,.F.);
#2306=ORIENTED_EDGE('',*,*,#1757,.F.);
#2307=ORIENTED_EDGE('',*,*,#1758,.F.);
#2308=ORIENTED_EDGE('',*,*,#1740,.F.);
#2309=ORIENTED_EDGE('',*,*,#1745,.T.);
#2310=ORIENTED_EDGE('',*,*,#1759,.T.);
#2311=ORIENTED_EDGE('',*,*,#1760,.T.);
#2312=ORIENTED_EDGE('',*,*,#1761,.T.);
#2313=ORIENTED_EDGE('',*,*,#1759,.F.);
#2314=ORIENTED_EDGE('',*,*,#1744,.T.);
#2315=ORIENTED_EDGE('',*,*,#1762,.T.);
#2316=ORIENTED_EDGE('',*,*,#1763,.F.);
#2317=ORIENTED_EDGE('',*,*,#1741,.F.);
#2318=ORIENTED_EDGE('',*,*,#1758,.T.);
#2319=ORIENTED_EDGE('',*,*,#1764,.F.);
#2320=ORIENTED_EDGE('',*,*,#1765,.F.);
#2321=ORIENTED_EDGE('',*,*,#1742,.T.);
#2322=ORIENTED_EDGE('',*,*,#1765,.T.);
#2323=ORIENTED_EDGE('',*,*,#1766,.F.);
#2324=ORIENTED_EDGE('',*,*,#1767,.F.);
#2325=ORIENTED_EDGE('',*,*,#1743,.T.);
#2326=ORIENTED_EDGE('',*,*,#1767,.T.);
#2327=ORIENTED_EDGE('',*,*,#1768,.F.);
#2328=ORIENTED_EDGE('',*,*,#1762,.F.);
#2329=ORIENTED_EDGE('',*,*,#1769,.T.);
#2330=ORIENTED_EDGE('',*,*,#1760,.F.);
#2331=ORIENTED_EDGE('',*,*,#1763,.T.);
#2332=ORIENTED_EDGE('',*,*,#1768,.T.);
#2333=ORIENTED_EDGE('',*,*,#1766,.T.);
#2334=ORIENTED_EDGE('',*,*,#1764,.T.);
#2335=ORIENTED_EDGE('',*,*,#1757,.T.);
#2336=ORIENTED_EDGE('',*,*,#1755,.F.);
#2337=ORIENTED_EDGE('',*,*,#1749,.T.);
#2338=ORIENTED_EDGE('',*,*,#1690,.F.);
#2339=ORIENTED_EDGE('',*,*,#1694,.T.);
#2340=ORIENTED_EDGE('',*,*,#1734,.T.);
#2341=ORIENTED_EDGE('',*,*,#1731,.T.);
#2342=ORIENTED_EDGE('',*,*,#1728,.T.);
#2343=ORIENTED_EDGE('',*,*,#1685,.T.);
#2344=ORIENTED_EDGE('',*,*,#1681,.F.);
#2345=ORIENTED_EDGE('',*,*,#1751,.T.);
#2346=ORIENTED_EDGE('',*,*,#1676,.F.);
#2347=ORIENTED_EDGE('',*,*,#1680,.T.);
#2348=ORIENTED_EDGE('',*,*,#1726,.T.);
#2349=ORIENTED_EDGE('',*,*,#1723,.T.);
#2350=ORIENTED_EDGE('',*,*,#1720,.T.);
#2351=ORIENTED_EDGE('',*,*,#1671,.T.);
#2352=ORIENTED_EDGE('',*,*,#1667,.F.);
#2353=ORIENTED_EDGE('',*,*,#1752,.T.);
#2354=ORIENTED_EDGE('',*,*,#1662,.F.);
#2355=ORIENTED_EDGE('',*,*,#1666,.T.);
#2356=ORIENTED_EDGE('',*,*,#1718,.T.);
#2357=ORIENTED_EDGE('',*,*,#1715,.T.);
#2358=ORIENTED_EDGE('',*,*,#1712,.T.);
#2359=ORIENTED_EDGE('',*,*,#1657,.T.);
#2360=ORIENTED_EDGE('',*,*,#1653,.F.);
#2361=ORIENTED_EDGE('',*,*,#1753,.T.);
#2362=ORIENTED_EDGE('',*,*,#1648,.F.);
#2363=ORIENTED_EDGE('',*,*,#1652,.T.);
#2364=ORIENTED_EDGE('',*,*,#1710,.T.);
#2365=ORIENTED_EDGE('',*,*,#1707,.T.);
#2366=ORIENTED_EDGE('',*,*,#1704,.T.);
#2367=ORIENTED_EDGE('',*,*,#1643,.T.);
#2368=ORIENTED_EDGE('',*,*,#1639,.F.);
#2369=ORIENTED_EDGE('',*,*,#1754,.T.);
#2370=ORIENTED_EDGE('',*,*,#1634,.F.);
#2371=ORIENTED_EDGE('',*,*,#1638,.T.);
#2372=ORIENTED_EDGE('',*,*,#1702,.T.);
#2373=ORIENTED_EDGE('',*,*,#1699,.T.);
#2374=ORIENTED_EDGE('',*,*,#1696,.T.);
#2375=ORIENTED_EDGE('',*,*,#1629,.T.);
#2376=ORIENTED_EDGE('',*,*,#1625,.F.);
#2377=ORIENTED_EDGE('',*,*,#1770,.T.);
#2378=ORIENTED_EDGE('',*,*,#1748,.T.);
#2379=ORIENTED_EDGE('',*,*,#1771,.T.);
#2380=ORIENTED_EDGE('',*,*,#1770,.F.);
#2381=ORIENTED_EDGE('',*,*,#1771,.F.);
#2382=ORIENTED_EDGE('',*,*,#1628,.F.);
#2383=ORIENTED_EDGE('',*,*,#1746,.T.);
#2384=ORIENTED_EDGE('',*,*,#1761,.F.);
#2385=ORIENTED_EDGE('',*,*,#1769,.F.);
#3026=CYLINDRICAL_SURFACE('',#3399,1.);
#3027=CYLINDRICAL_SURFACE('',#3403,1.);
#3028=CYLINDRICAL_SURFACE('',#3407,1.);
#3029=CYLINDRICAL_SURFACE('',#3411,1.);
#3030=CYLINDRICAL_SURFACE('',#3415,1.);
#3031=CYLINDRICAL_SURFACE('',#3419,1.);
#3032=CYLINDRICAL_SURFACE('',#3423,1.);
#3033=CYLINDRICAL_SURFACE('',#3427,1.);
#3034=CYLINDRICAL_SURFACE('',#3431,1.);
#3035=CYLINDRICAL_SURFACE('',#3435,1.);
#3036=CYLINDRICAL_SURFACE('',#3439,11.9999999999996);
#3037=CYLINDRICAL_SURFACE('',#3442,11.9999999999996);
#3038=CYLINDRICAL_SURFACE('',#3445,11.9999999999996);
#3039=CYLINDRICAL_SURFACE('',#3448,11.9999999999996);
#3040=CYLINDRICAL_SURFACE('',#3451,11.9999999999996);
#3041=CYLINDRICAL_SURFACE('',#3465,5.529);
#3042=CYLINDRICAL_SURFACE('',#3467,5.529);
#3043=CYLINDRICAL_SURFACE('',#3469,5.529);
#3044=CYLINDRICAL_SURFACE('',#3471,5.529);
#3045=CYLINDRICAL_SURFACE('',#3473,5.529);
#3046=CYLINDRICAL_SURFACE('',#3475,1.);
#3047=CYLINDRICAL_SURFACE('',#3478,1.);
#3048=CYLINDRICAL_SURFACE('',#3481,11.9999999999996);
#3049=CYLINDRICAL_SURFACE('',#3486,5.);
#3050=CYLINDRICAL_SURFACE('',#3487,5.529);
#3103=ADVANCED_FACE('',(#265),#3026,.F.);
#3104=ADVANCED_FACE('',(#266),#181,.T.);
#3105=ADVANCED_FACE('',(#267),#3027,.F.);
#3106=ADVANCED_FACE('',(#268),#182,.T.);
#3107=ADVANCED_FACE('',(#269),#3028,.F.);
#3108=ADVANCED_FACE('',(#270),#183,.T.);
#3109=ADVANCED_FACE('',(#271),#3029,.F.);
#3110=ADVANCED_FACE('',(#272),#184,.T.);
#3111=ADVANCED_FACE('',(#273),#3030,.F.);
#3112=ADVANCED_FACE('',(#274),#185,.T.);
#3113=ADVANCED_FACE('',(#275),#3031,.F.);
#3114=ADVANCED_FACE('',(#276),#186,.T.);
#3115=ADVANCED_FACE('',(#277),#3032,.F.);
#3116=ADVANCED_FACE('',(#278),#187,.T.);
#3117=ADVANCED_FACE('',(#279),#3033,.F.);
#3118=ADVANCED_FACE('',(#280),#188,.T.);
#3119=ADVANCED_FACE('',(#281),#3034,.F.);
#3120=ADVANCED_FACE('',(#282),#189,.T.);
#3121=ADVANCED_FACE('',(#283),#3035,.F.);
#3122=ADVANCED_FACE('',(#284),#190,.T.);
#3123=ADVANCED_FACE('',(#285),#157,.T.);
#3124=ADVANCED_FACE('',(#286),#3036,.T.);
#3125=ADVANCED_FACE('',(#287),#158,.T.);
#3126=ADVANCED_FACE('',(#288),#159,.T.);
#3127=ADVANCED_FACE('',(#289),#3037,.T.);
#3128=ADVANCED_FACE('',(#290),#160,.T.);
#3129=ADVANCED_FACE('',(#291),#161,.T.);
#3130=ADVANCED_FACE('',(#292),#3038,.T.);
#3131=ADVANCED_FACE('',(#293),#162,.T.);
#3132=ADVANCED_FACE('',(#294),#163,.T.);
#3133=ADVANCED_FACE('',(#295),#3039,.T.);
#3134=ADVANCED_FACE('',(#296),#164,.T.);
#3135=ADVANCED_FACE('',(#297),#165,.T.);
#3136=ADVANCED_FACE('',(#298),#3040,.T.);
#3137=ADVANCED_FACE('',(#299),#166,.T.);
#3138=ADVANCED_FACE('',(#300,#83),#191,.F.);
#3139=ADVANCED_FACE('',(#301),#3041,.T.);
#3140=ADVANCED_FACE('',(#302),#3042,.T.);
#3141=ADVANCED_FACE('',(#303),#3043,.T.);
#3142=ADVANCED_FACE('',(#304),#3044,.T.);
#3143=ADVANCED_FACE('',(#305),#3045,.T.);
#3144=ADVANCED_FACE('',(#306),#3046,.F.);
#3145=ADVANCED_FACE('',(#307),#192,.T.);
#3146=ADVANCED_FACE('',(#308),#3047,.F.);
#3147=ADVANCED_FACE('',(#309),#193,.T.);
#3148=ADVANCED_FACE('',(#310),#167,.T.);
#3149=ADVANCED_FACE('',(#311),#3048,.T.);
#3150=ADVANCED_FACE('',(#312),#168,.T.);
#3151=ADVANCED_FACE('',(#313,#84),#194,.T.);
#3152=ADVANCED_FACE('',(#314),#3049,.F.);
#3153=ADVANCED_FACE('',(#315),#3050,.T.);
#3288=CLOSED_SHELL('',(#3103,#3104,#3105,#3106,#3107,#3108,#3109,#3110,
#3111,#3112,#3113,#3114,#3115,#3116,#3117,#3118,#3119,#3120,#3121,#3122,
#3123,#3124,#3125,#3126,#3127,#3128,#3129,#3130,#3131,#3132,#3133,#3134,
#3135,#3136,#3137,#3138,#3139,#3140,#3141,#3142,#3143,#3144,#3145,#3146,
#3147,#3148,#3149,#3150,#3151,#3152,#3153));
#3398=AXIS2_PLACEMENT_3D('',#4647,#3729,#3730);
#3399=AXIS2_PLACEMENT_3D('',#4648,#3731,#3732);
#3400=AXIS2_PLACEMENT_3D('',#4651,#3733,#3734);
#3401=AXIS2_PLACEMENT_3D('',#4655,#3736,#3737);
#3402=AXIS2_PLACEMENT_3D('',#4657,#3739,#3740);
#3403=AXIS2_PLACEMENT_3D('',#4663,#3744,#3745);
#3404=AXIS2_PLACEMENT_3D('',#4666,#3746,#3747);
#3405=AXIS2_PLACEMENT_3D('',#4670,#3749,#3750);
#3406=AXIS2_PLACEMENT_3D('',#4672,#3752,#3753);
#3407=AXIS2_PLACEMENT_3D('',#4678,#3757,#3758);
#3408=AXIS2_PLACEMENT_3D('',#4681,#3759,#3760);
#3409=AXIS2_PLACEMENT_3D('',#4685,#3762,#3763);
#3410=AXIS2_PLACEMENT_3D('',#4687,#3765,#3766);
#3411=AXIS2_PLACEMENT_3D('',#4693,#3770,#3771);
#3412=AXIS2_PLACEMENT_3D('',#4696,#3772,#3773);
#3413=AXIS2_PLACEMENT_3D('',#4700,#3775,#3776);
#3414=AXIS2_PLACEMENT_3D('',#4702,#3778,#3779);
#3415=AXIS2_PLACEMENT_3D('',#4708,#3783,#3784);
#3416=AXIS2_PLACEMENT_3D('',#4711,#3785,#3786);
#3417=AXIS2_PLACEMENT_3D('',#4715,#3788,#3789);
#3418=AXIS2_PLACEMENT_3D('',#4717,#3791,#3792);
#3419=AXIS2_PLACEMENT_3D('',#4723,#3796,#3797);
#3420=AXIS2_PLACEMENT_3D('',#4726,#3798,#3799);
#3421=AXIS2_PLACEMENT_3D('',#4730,#3801,#3802);
#3422=AXIS2_PLACEMENT_3D('',#4732,#3804,#3805);
#3423=AXIS2_PLACEMENT_3D('',#4738,#3809,#3810);
#3424=AXIS2_PLACEMENT_3D('',#4741,#3811,#3812);
#3425=AXIS2_PLACEMENT_3D('',#4745,#3814,#3815);
#3426=AXIS2_PLACEMENT_3D('',#4747,#3817,#3818);
#3427=AXIS2_PLACEMENT_3D('',#4753,#3822,#3823);
#3428=AXIS2_PLACEMENT_3D('',#4756,#3824,#3825);
#3429=AXIS2_PLACEMENT_3D('',#4760,#3827,#3828);
#3430=AXIS2_PLACEMENT_3D('',#4762,#3830,#3831);
#3431=AXIS2_PLACEMENT_3D('',#4768,#3835,#3836);
#3432=AXIS2_PLACEMENT_3D('',#4771,#3837,#3838);
#3433=AXIS2_PLACEMENT_3D('',#4775,#3840,#3841);
#3434=AXIS2_PLACEMENT_3D('',#4777,#3843,#3844);
#3435=AXIS2_PLACEMENT_3D('',#4783,#3848,#3849);
#3436=AXIS2_PLACEMENT_3D('',#4786,#3850,#3851);
#3437=AXIS2_PLACEMENT_3D('',#4790,#3853,#3854);
#3438=AXIS2_PLACEMENT_3D('',#4792,#3856,#3857);
#3439=AXIS2_PLACEMENT_3D('',#5101,#3862,#3863);
#3440=AXIS2_PLACEMENT_3D('',#5103,#3864,#3865);
#3441=AXIS2_PLACEMENT_3D('',#5105,#3866,#3867);
#3442=AXIS2_PLACEMENT_3D('',#5710,#3870,#3871);
#3443=AXIS2_PLACEMENT_3D('',#5712,#3872,#3873);
#3444=AXIS2_PLACEMENT_3D('',#5714,#3874,#3875);
#3445=AXIS2_PLACEMENT_3D('',#6319,#3878,#3879);
#3446=AXIS2_PLACEMENT_3D('',#6321,#3880,#3881);
#3447=AXIS2_PLACEMENT_3D('',#6323,#3882,#3883);
#3448=AXIS2_PLACEMENT_3D('',#6928,#3886,#3887);
#3449=AXIS2_PLACEMENT_3D('',#6930,#3888,#3889);
#3450=AXIS2_PLACEMENT_3D('',#6932,#3890,#3891);
#3451=AXIS2_PLACEMENT_3D('',#7537,#3894,#3895);
#3452=AXIS2_PLACEMENT_3D('',#7539,#3896,#3897);
#3453=AXIS2_PLACEMENT_3D('',#7541,#3898,#3899);
#3454=AXIS2_PLACEMENT_3D('',#7843,#3901,#3902);
#3455=AXIS2_PLACEMENT_3D('',#7844,#3903,#3904);
#3456=AXIS2_PLACEMENT_3D('',#7845,#3905,#3906);
#3457=AXIS2_PLACEMENT_3D('',#7846,#3907,#3908);
#3458=AXIS2_PLACEMENT_3D('',#7848,#3909,#3910);
#3459=AXIS2_PLACEMENT_3D('',#7850,#3911,#3912);
#3460=AXIS2_PLACEMENT_3D('',#7930,#3914,#3915);
#3461=AXIS2_PLACEMENT_3D('',#8010,#3917,#3918);
#3462=AXIS2_PLACEMENT_3D('',#8011,#3919,#3920);
#3463=AXIS2_PLACEMENT_3D('',#8012,#3921,#3922);
#3464=AXIS2_PLACEMENT_3D('',#8014,#3923,#3924);
#3465=AXIS2_PLACEMENT_3D('',#8015,#3925,#3926);
#3466=AXIS2_PLACEMENT_3D('',#8017,#3927,#3928);
#3467=AXIS2_PLACEMENT_3D('',#8019,#3930,#3931);
#3468=AXIS2_PLACEMENT_3D('',#8020,#3932,#3933);
#3469=AXIS2_PLACEMENT_3D('',#8021,#3934,#3935);
#3470=AXIS2_PLACEMENT_3D('',#8022,#3936,#3937);
#3471=AXIS2_PLACEMENT_3D('',#8023,#3938,#3939);
#3472=AXIS2_PLACEMENT_3D('',#8024,#3940,#3941);
#3473=AXIS2_PLACEMENT_3D('',#8025,#3942,#3943);
#3474=AXIS2_PLACEMENT_3D('',#8026,#3944,#3945);
#3475=AXIS2_PLACEMENT_3D('',#8027,#3946,#3947);
#3476=AXIS2_PLACEMENT_3D('',#8029,#3948,#3949);
#3477=AXIS2_PLACEMENT_3D('',#8031,#3951,#3952);
#3478=AXIS2_PLACEMENT_3D('',#8035,#3955,#3956);
#3479=AXIS2_PLACEMENT_3D('',#8039,#3958,#3959);
#3480=AXIS2_PLACEMENT_3D('',#8041,#3961,#3962);
#3481=AXIS2_PLACEMENT_3D('',#8272,#3966,#3967);
#3482=AXIS2_PLACEMENT_3D('',#8274,#3968,#3969);
#3483=AXIS2_PLACEMENT_3D('',#8501,#3971,#3972);
#3484=AXIS2_PLACEMENT_3D('',#8502,#3973,#3974);
#3485=AXIS2_PLACEMENT_3D('',#8504,#3975,#3976);
#3486=AXIS2_PLACEMENT_3D('',#8505,#3977,#3978);
#3487=AXIS2_PLACEMENT_3D('',#8507,#3980,#3981);
#3729=DIRECTION('axis',(0.,0.,1.));
#3730=DIRECTION('refdir',(1.,0.,0.));
#3731=DIRECTION('center_axis',(0.,0.,-1.));
#3732=DIRECTION('ref_axis',(-0.995790400289429,-0.091659580467175,0.));
#3733=DIRECTION('center_axis',(0.,0.,-1.));
#3734=DIRECTION('ref_axis',(-0.995790400289429,-0.091659580467175,0.));
#3735=DIRECTION('',(0.,0.,-1.));
#3736=DIRECTION('center_axis',(0.,0.,-1.));
#3737=DIRECTION('ref_axis',(-0.995790400289429,-0.091659580467175,0.));
#3738=DIRECTION('',(0.,0.,1.));
#3739=DIRECTION('center_axis',(0.696489643340828,0.717566844774037,0.));
#3740=DIRECTION('ref_axis',(-0.717566844774037,0.696489643340828,0.));
#3741=DIRECTION('',(-0.717566844774037,0.696489643340828,0.));
#3742=DIRECTION('',(0.,0.,1.));
#3743=DIRECTION('',(-0.717566844774037,0.696489643340828,0.));
#3744=DIRECTION('center_axis',(0.,0.,1.));
#3745=DIRECTION('ref_axis',(0.577274725329514,0.816549993261732,0.));
#3746=DIRECTION('center_axis',(0.,0.,-1.));
#3747=DIRECTION('ref_axis',(0.577274725329514,0.816549993261732,0.));
#3748=DIRECTION('',(0.,0.,1.));
#3749=DIRECTION('center_axis',(0.,0.,-1.));
#3750=DIRECTION('ref_axis',(0.577274725329514,0.816549993261732,0.));
#3751=DIRECTION('',(0.,0.,-1.));
#3752=DIRECTION('center_axis',(-0.969675938158175,-0.2443943022189,0.));
#3753=DIRECTION('ref_axis',(0.2443943022189,-0.969675938158175,0.));
#3754=DIRECTION('',(0.2443943022189,-0.969675938158175,0.));
#3755=DIRECTION('',(0.,0.,1.));
#3756=DIRECTION('',(0.2443943022189,-0.969675938158175,0.));
#3757=DIRECTION('center_axis',(0.,0.,-1.));
#3758=DIRECTION('ref_axis',(-0.577274725329512,0.816549993261733,0.));
#3759=DIRECTION('center_axis',(0.,0.,-1.));
#3760=DIRECTION('ref_axis',(-0.577274725329512,0.816549993261733,0.));
#3761=DIRECTION('',(0.,0.,-1.));
#3762=DIRECTION('center_axis',(0.,0.,-1.));
#3763=DIRECTION('ref_axis',(-0.577274725329512,0.816549993261733,0.));
#3764=DIRECTION('',(0.,0.,1.));
#3765=DIRECTION('center_axis',(0.969675938158175,-0.244394302218901,0.));
#3766=DIRECTION('ref_axis',(0.244394302218901,0.969675938158175,0.));
#3767=DIRECTION('',(0.244394302218901,0.969675938158175,0.));
#3768=DIRECTION('',(0.,0.,1.));
#3769=DIRECTION('',(0.244394302218901,0.969675938158175,0.));
#3770=DIRECTION('center_axis',(0.,0.,1.));
#3771=DIRECTION('ref_axis',(0.995790400289429,-0.0916595804671751,0.));
#3772=DIRECTION('center_axis',(0.,0.,-1.));
#3773=DIRECTION('ref_axis',(0.995790400289429,-0.0916595804671751,0.));
#3774=DIRECTION('',(0.,0.,1.));
#3775=DIRECTION('center_axis',(0.,0.,-1.));
#3776=DIRECTION('ref_axis',(0.995790400289429,-0.0916595804671751,0.));
#3777=DIRECTION('',(0.,0.,-1.));
#3778=DIRECTION('center_axis',(-0.696489643340827,0.717566844774038,0.));
#3779=DIRECTION('ref_axis',(-0.717566844774038,-0.696489643340827,0.));
#3780=DIRECTION('',(-0.717566844774038,-0.696489643340827,0.));
#3781=DIRECTION('',(0.,0.,1.));
#3782=DIRECTION('',(-0.717566844774038,-0.696489643340827,0.));
#3783=DIRECTION('center_axis',(0.,0.,-1.));
#3784=DIRECTION('ref_axis',(0.418515674959917,0.908209573728908,0.));
#3785=DIRECTION('center_axis',(0.,0.,-1.));
#3786=DIRECTION('ref_axis',(0.418515674959917,0.908209573728908,0.));
#3787=DIRECTION('',(0.,0.,-1.));
#3788=DIRECTION('center_axis',(0.,0.,-1.));
#3789=DIRECTION('ref_axis',(0.418515674959917,0.908209573728908,0.));
#3790=DIRECTION('',(0.,0.,1.));
#3791=DIRECTION('center_axis',(0.273186294817348,-0.961961146992938,0.));
#3792=DIRECTION('ref_axis',(0.961961146992938,0.273186294817348,0.));
#3793=DIRECTION('',(0.961961146992938,0.273186294817348,0.));
#3794=DIRECTION('',(0.,0.,1.));
#3795=DIRECTION('',(0.961961146992938,0.273186294817348,0.));
#3796=DIRECTION('center_axis',(0.,0.,1.));
#3797=DIRECTION('ref_axis',(0.418515674959918,-0.908209573728908,0.));
#3798=DIRECTION('center_axis',(0.,0.,-1.));
#3799=DIRECTION('ref_axis',(0.418515674959918,-0.908209573728908,0.));
#3800=DIRECTION('',(0.,0.,1.));
#3801=DIRECTION('center_axis',(0.,0.,-1.));
#3802=DIRECTION('ref_axis',(0.418515674959918,-0.908209573728908,0.));
#3803=DIRECTION('',(0.,0.,-1.));
#3804=DIRECTION('center_axis',(0.273186294817348,0.961961146992938,0.));
#3805=DIRECTION('ref_axis',(-0.961961146992938,0.273186294817348,0.));
#3806=DIRECTION('',(-0.961961146992938,0.273186294817348,0.));
#3807=DIRECTION('',(0.,0.,1.));
#3808=DIRECTION('',(-0.961961146992938,0.273186294817348,0.));
#3809=DIRECTION('center_axis',(0.,0.,-1.));
#3810=DIRECTION('ref_axis',(0.995790400289429,0.0916595804671737,0.));
#3811=DIRECTION('center_axis',(0.,0.,-1.));
#3812=DIRECTION('ref_axis',(0.995790400289429,0.0916595804671737,0.));
#3813=DIRECTION('',(0.,0.,-1.));
#3814=DIRECTION('center_axis',(0.,0.,-1.));
#3815=DIRECTION('ref_axis',(0.995790400289429,0.0916595804671737,0.));
#3816=DIRECTION('',(0.,0.,1.));
#3817=DIRECTION('center_axis',(-0.696489643340827,-0.717566844774037,0.));
#3818=DIRECTION('ref_axis',(0.717566844774037,-0.696489643340827,0.));
#3819=DIRECTION('',(0.717566844774037,-0.696489643340827,0.));
#3820=DIRECTION('',(0.,0.,1.));
#3821=DIRECTION('',(0.717566844774037,-0.696489643340827,0.));
#3822=DIRECTION('center_axis',(0.,0.,1.));
#3823=DIRECTION('ref_axis',(-0.577274725329511,-0.816549993261734,0.));
#3824=DIRECTION('center_axis',(0.,0.,-1.));
#3825=DIRECTION('ref_axis',(-0.577274725329511,-0.816549993261734,0.));
#3826=DIRECTION('',(0.,0.,1.));
#3827=DIRECTION('center_axis',(0.,0.,-1.));
#3828=DIRECTION('ref_axis',(-0.577274725329511,-0.816549993261734,0.));
#3829=DIRECTION('',(0.,0.,-1.));
#3830=DIRECTION('center_axis',(0.969675938158175,0.244394302218901,0.));
#3831=DIRECTION('ref_axis',(-0.244394302218901,0.969675938158175,0.));
#3832=DIRECTION('',(-0.244394302218901,0.969675938158175,0.));
#3833=DIRECTION('',(0.,0.,1.));
#3834=DIRECTION('',(-0.244394302218901,0.969675938158175,0.));
#3835=DIRECTION('center_axis',(0.,0.,-1.));
#3836=DIRECTION('ref_axis',(0.577274725329512,-0.816549993261733,0.));
#3837=DIRECTION('center_axis',(0.,0.,-1.));
#3838=DIRECTION('ref_axis',(0.577274725329512,-0.816549993261733,0.));
#3839=DIRECTION('',(0.,0.,-1.));
#3840=DIRECTION('center_axis',(0.,0.,-1.));
#3841=DIRECTION('ref_axis',(0.577274725329512,-0.816549993261733,0.));
#3842=DIRECTION('',(0.,0.,1.));
#3843=DIRECTION('center_axis',(-0.969675938158175,0.244394302218901,0.));
#3844=DIRECTION('ref_axis',(-0.244394302218901,-0.969675938158175,0.));
#3845=DIRECTION('',(-0.244394302218901,-0.969675938158175,0.));
#3846=DIRECTION('',(0.,0.,1.));
#3847=DIRECTION('',(-0.244394302218901,-0.969675938158175,0.));
#3848=DIRECTION('center_axis',(0.,0.,1.));
#3849=DIRECTION('ref_axis',(-0.995790400289429,0.0916595804671751,0.));
#3850=DIRECTION('center_axis',(0.,0.,-1.));
#3851=DIRECTION('ref_axis',(-0.995790400289429,0.0916595804671751,0.));
#3852=DIRECTION('',(0.,0.,1.));
#3853=DIRECTION('center_axis',(0.,0.,-1.));
#3854=DIRECTION('ref_axis',(-0.995790400289429,0.0916595804671751,0.));
#3855=DIRECTION('',(0.,0.,-1.));
#3856=DIRECTION('center_axis',(0.696489643340827,-0.717566844774037,0.));
#3857=DIRECTION('ref_axis',(0.717566844774037,0.696489643340827,0.));
#3858=DIRECTION('',(0.717566844774037,0.696489643340827,0.));
#3859=DIRECTION('',(0.,0.,1.));
#3860=DIRECTION('',(0.717566844774037,0.696489643340827,0.));
#3861=DIRECTION('',(0.,0.,1.));
#3862=DIRECTION('center_axis',(0.,0.,1.));
#3863=DIRECTION('ref_axis',(0.448260781250512,-0.893902831404332,0.));
#3864=DIRECTION('center_axis',(0.,0.,1.));
#3865=DIRECTION('ref_axis',(0.448260781250512,-0.893902831404332,0.));
#3866=DIRECTION('center_axis',(0.,0.,1.));
#3867=DIRECTION('ref_axis',(0.448260781250512,-0.893902831404332,0.));
#3868=DIRECTION('',(0.,0.,1.));
#3869=DIRECTION('',(0.,0.,1.));
#3870=DIRECTION('center_axis',(0.,0.,1.));
#3871=DIRECTION('ref_axis',(-0.550012169885733,-0.835156639785368,0.));
#3872=DIRECTION('center_axis',(0.,0.,1.));
#3873=DIRECTION('ref_axis',(-0.550012169885733,-0.835156639785368,0.));
#3874=DIRECTION('center_axis',(0.,0.,1.));
#3875=DIRECTION('ref_axis',(-0.550012169885733,-0.835156639785368,0.));
#3876=DIRECTION('',(0.,0.,1.));
#3877=DIRECTION('',(0.,0.,1.));
#3878=DIRECTION('center_axis',(0.,0.,1.));
#3879=DIRECTION('ref_axis',(-0.998272951136245,0.0587461916189628,0.));
#3880=DIRECTION('center_axis',(0.,0.,1.));
#3881=DIRECTION('ref_axis',(-0.998272951136245,0.0587461916189628,0.));
#3882=DIRECTION('center_axis',(0.,0.,1.));
#3883=DIRECTION('ref_axis',(-0.998272951136245,0.0587461916189628,0.));
#3884=DIRECTION('',(0.,0.,1.));
#3885=DIRECTION('',(0.,0.,1.));
#3886=DIRECTION('center_axis',(0.,0.,1.));
#3887=DIRECTION('ref_axis',(-0.448260781250512,0.893902831404331,0.));
#3888=DIRECTION('center_axis',(0.,0.,1.));
#3889=DIRECTION('ref_axis',(-0.448260781250512,0.893902831404331,0.));
#3890=DIRECTION('center_axis',(0.,0.,1.));
#3891=DIRECTION('ref_axis',(-0.448260781250512,0.893902831404331,0.));
#3892=DIRECTION('',(0.,0.,1.));
#3893=DIRECTION('',(0.,0.,1.));
#3894=DIRECTION('center_axis',(0.,0.,1.));
#3895=DIRECTION('ref_axis',(0.550012169885733,0.835156639785369,0.));
#3896=DIRECTION('center_axis',(0.,0.,1.));
#3897=DIRECTION('ref_axis',(0.550012169885733,0.835156639785369,0.));
#3898=DIRECTION('center_axis',(0.,0.,1.));
#3899=DIRECTION('ref_axis',(0.550012169885733,0.835156639785369,0.));
#3900=DIRECTION('',(0.,0.,1.));
#3901=DIRECTION('center_axis',(0.,0.,1.));
#3902=DIRECTION('ref_axis',(1.,0.,0.));
#3903=DIRECTION('center_axis',(0.,0.,1.));
#3904=DIRECTION('ref_axis',(1.,0.,0.));
#3905=DIRECTION('center_axis',(0.,0.,1.));
#3906=DIRECTION('ref_axis',(1.,0.,0.));
#3907=DIRECTION('center_axis',(0.,0.,1.));
#3908=DIRECTION('ref_axis',(1.,0.,0.));
#3909=DIRECTION('center_axis',(0.,0.,1.));
#3910=DIRECTION('ref_axis',(1.,0.,0.));
#3911=DIRECTION('center_axis',(0.,0.,-1.));
#3912=DIRECTION('ref_axis',(-0.418515674959917,-0.908209573728908,0.));
#3913=DIRECTION('',(-0.961961146992938,-0.273186294817348,0.));
#3914=DIRECTION('center_axis',(0.,0.,1.));
#3915=DIRECTION('ref_axis',(0.998272951136245,-0.0587461916189627,0.));
#3916=DIRECTION('',(0.961961146992938,-0.273186294817348,0.));
#3917=DIRECTION('center_axis',(0.,0.,-1.));
#3918=DIRECTION('ref_axis',(-0.418515674959917,0.908209573728908,0.));
#3919=DIRECTION('center_axis',(0.,0.,1.));
#3920=DIRECTION('ref_axis',(1.,0.,0.));
#3921=DIRECTION('center_axis',(0.,0.,1.));
#3922=DIRECTION('ref_axis',(1.,0.,0.));
#3923=DIRECTION('center_axis',(0.,0.,-1.));
#3924=DIRECTION('ref_axis',(1.,0.,0.));
#3925=DIRECTION('center_axis',(0.,0.,1.));
#3926=DIRECTION('ref_axis',(1.,0.,0.));
#3927=DIRECTION('center_axis',(0.,0.,1.));
#3928=DIRECTION('ref_axis',(1.,0.,0.));
#3929=DIRECTION('',(0.,0.,1.));
#3930=DIRECTION('center_axis',(0.,0.,1.));
#3931=DIRECTION('ref_axis',(1.,0.,0.));
#3932=DIRECTION('center_axis',(0.,0.,1.));
#3933=DIRECTION('ref_axis',(1.,0.,0.));
#3934=DIRECTION('center_axis',(0.,0.,1.));
#3935=DIRECTION('ref_axis',(1.,0.,0.));
#3936=DIRECTION('center_axis',(0.,0.,1.));
#3937=DIRECTION('ref_axis',(1.,0.,0.));
#3938=DIRECTION('center_axis',(0.,0.,1.));
#3939=DIRECTION('ref_axis',(1.,0.,0.));
#3940=DIRECTION('center_axis',(0.,0.,1.));
#3941=DIRECTION('ref_axis',(1.,0.,0.));
#3942=DIRECTION('center_axis',(0.,0.,1.));
#3943=DIRECTION('ref_axis',(1.,0.,0.));
#3944=DIRECTION('center_axis',(0.,0.,1.));
#3945=DIRECTION('ref_axis',(1.,0.,0.));
#3946=DIRECTION('center_axis',(0.,0.,-1.));
#3947=DIRECTION('ref_axis',(-0.418515674959917,-0.908209573728908,0.));
#3948=DIRECTION('center_axis',(0.,0.,-1.));
#3949=DIRECTION('ref_axis',(-0.418515674959917,-0.908209573728908,0.));
#3950=DIRECTION('',(0.,0.,-1.));
#3951=DIRECTION('center_axis',(-0.273186294817348,0.961961146992938,0.));
#3952=DIRECTION('ref_axis',(-0.961961146992938,-0.273186294817348,0.));
#3953=DIRECTION('',(-0.961961146992938,-0.273186294817348,0.));
#3954=DIRECTION('',(0.,0.,1.));
#3955=DIRECTION('center_axis',(0.,0.,1.));
#3956=DIRECTION('ref_axis',(-0.418515674959917,0.908209573728908,0.));
#3957=DIRECTION('',(0.,0.,1.));
#3958=DIRECTION('center_axis',(0.,0.,-1.));
#3959=DIRECTION('ref_axis',(-0.418515674959917,0.908209573728908,0.));
#3960=DIRECTION('',(0.,0.,-1.));
#3961=DIRECTION('center_axis',(-0.273186294817348,-0.961961146992938,0.));
#3962=DIRECTION('ref_axis',(0.961961146992938,-0.273186294817348,0.));
#3963=DIRECTION('',(0.,0.,1.));
#3964=DIRECTION('',(0.961961146992938,-0.273186294817348,0.));
#3965=DIRECTION('',(0.,0.,1.));
#3966=DIRECTION('center_axis',(0.,0.,1.));
#3967=DIRECTION('ref_axis',(0.998272951136245,-0.0587461916189627,0.));
#3968=DIRECTION('center_axis',(0.,0.,1.));
#3969=DIRECTION('ref_axis',(0.998272951136245,-0.0587461916189627,0.));
#3970=DIRECTION('',(0.,0.,1.));
#3971=DIRECTION('center_axis',(0.,0.,1.));
#3972=DIRECTION('ref_axis',(1.,0.,0.));
#3973=DIRECTION('center_axis',(0.,0.,1.));
#3974=DIRECTION('ref_axis',(1.,0.,0.));
#3975=DIRECTION('center_axis',(0.,0.,-1.));
#3976=DIRECTION('ref_axis',(1.,0.,0.));
#3977=DIRECTION('center_axis',(0.,0.,1.));
#3978=DIRECTION('ref_axis',(1.,0.,0.));
#3979=DIRECTION('',(0.,0.,1.));
#3980=DIRECTION('center_axis',(0.,0.,1.));
#3981=DIRECTION('ref_axis',(1.,0.,0.));
#4647=CARTESIAN_POINT('',(0.,0.,0.));
#4648=CARTESIAN_POINT('Origin',(5.32620517920381,-3.77615934370129,0.));
#4649=CARTESIAN_POINT('',(4.51042861629926,-3.1977921597985,6.));
#4650=CARTESIAN_POINT('',(4.62971553586298,-4.49372618847532,6.));
#4651=CARTESIAN_POINT('Origin',(5.32620517920381,-3.77615934370129,6.));
#4652=CARTESIAN_POINT('',(4.62971553586298,-4.49372618847532,-1.));
#4653=CARTESIAN_POINT('',(4.62971553586298,-4.49372618847532,0.));
#4654=CARTESIAN_POINT('',(4.51042861629926,-3.1977921597985,-1.));
#4655=CARTESIAN_POINT('Origin',(5.32620517920381,-3.77615934370129,-1.));
#4656=CARTESIAN_POINT('',(4.51042861629926,-3.1977921597985,0.));
#4657=CARTESIAN_POINT('Origin',(6.06863042059311,-5.89037560471067,0.));
#4658=CARTESIAN_POINT('',(6.06863042059311,-5.89037560471067,6.));
#4659=CARTESIAN_POINT('',(3.03431521029655,-2.94518780235533,6.));
#4660=CARTESIAN_POINT('',(6.06863042059311,-5.89037560471067,-1.));
#4661=CARTESIAN_POINT('',(6.06863042059311,-5.89037560471067,0.));
#4662=CARTESIAN_POINT('',(3.03431521029655,-2.94518780235533,-1.));
#4663=CARTESIAN_POINT('Origin',(0.607147330781373,-6.50070866280939,0.));
#4664=CARTESIAN_POINT('',(0.514154938258571,-5.5050418435707,-1.));
#4665=CARTESIAN_POINT('',(1.57682326893955,-6.25631436059049,-1.));
#4666=CARTESIAN_POINT('Origin',(0.607147330781373,-6.50070866280939,-1.));
#4667=CARTESIAN_POINT('',(1.57682326893955,-6.25631436059049,6.));
#4668=CARTESIAN_POINT('',(1.57682326893955,-6.25631436059049,0.));
#4669=CARTESIAN_POINT('',(0.514154938258571,-5.5050418435707,6.));
#4670=CARTESIAN_POINT('Origin',(0.607147330781373,-6.50070866280939,6.));
#4671=CARTESIAN_POINT('',(0.514154938258571,-5.5050418435707,0.));
#4672=CARTESIAN_POINT('Origin',(1.34881215394611,-5.35164150269497,0.));
#4673=CARTESIAN_POINT('',(2.06689970121499,-8.20077591276801,-1.));
#4674=CARTESIAN_POINT('',(0.674406076973055,-2.67582075134748,-1.));
#4675=CARTESIAN_POINT('',(2.06689970121499,-8.20077591276801,6.));
#4676=CARTESIAN_POINT('',(2.06689970121499,-8.20077591276801,0.));
#4677=CARTESIAN_POINT('',(0.674406076973055,-2.67582075134748,6.));
#4678=CARTESIAN_POINT('Origin',(-0.607147330781383,-6.50070866280939,0.));
#4679=CARTESIAN_POINT('',(-0.51415493825858,-5.5050418435707,6.));
#4680=CARTESIAN_POINT('',(-1.57682326893956,-6.25631436059049,6.));
#4681=CARTESIAN_POINT('Origin',(-0.607147330781383,-6.50070866280939,6.));
#4682=CARTESIAN_POINT('',(-1.57682326893956,-6.25631436059049,-1.));
#4683=CARTESIAN_POINT('',(-1.57682326893956,-6.25631436059049,0.));
#4684=CARTESIAN_POINT('',(-0.51415493825858,-5.5050418435707,-1.));
#4685=CARTESIAN_POINT('Origin',(-0.607147330781383,-6.50070866280939,-1.));
#4686=CARTESIAN_POINT('',(-0.51415493825858,-5.5050418435707,0.));
#4687=CARTESIAN_POINT('Origin',(-2.06689970121501,-8.20077591276801,0.));
#4688=CARTESIAN_POINT('',(-2.06689970121501,-8.20077591276801,6.));
#4689=CARTESIAN_POINT('',(-1.0334498506075,-4.100387956384,6.));
#4690=CARTESIAN_POINT('',(-2.06689970121501,-8.20077591276801,-1.));
#4691=CARTESIAN_POINT('',(-2.06689970121501,-8.20077591276801,0.));
#4692=CARTESIAN_POINT('',(-1.0334498506075,-4.100387956384,-1.));
#4693=CARTESIAN_POINT('Origin',(-5.32620517920381,-3.77615934370128,0.));
#4694=CARTESIAN_POINT('',(-4.51042861629926,-3.1977921597985,-1.));
#4695=CARTESIAN_POINT('',(-4.62971553586298,-4.49372618847532,-1.));
#4696=CARTESIAN_POINT('Origin',(-5.32620517920381,-3.77615934370128,-1.));
#4697=CARTESIAN_POINT('',(-4.62971553586298,-4.49372618847532,6.));
#4698=CARTESIAN_POINT('',(-4.62971553586298,-4.49372618847532,0.));
#4699=CARTESIAN_POINT('',(-4.51042861629926,-3.1977921597985,6.));
#4700=CARTESIAN_POINT('Origin',(-5.32620517920381,-3.77615934370128,6.));
#4701=CARTESIAN_POINT('',(-4.51042861629926,-3.1977921597985,0.));
#4702=CARTESIAN_POINT('Origin',(-3.96025141630791,-3.84392634159802,0.));
#4703=CARTESIAN_POINT('',(-6.06863042059311,-5.89037560471066,-1.));
#4704=CARTESIAN_POINT('',(-1.98012570815396,-1.92196317079901,-1.));
#4705=CARTESIAN_POINT('',(-6.06863042059311,-5.89037560471066,6.));
#4706=CARTESIAN_POINT('',(-6.06863042059311,-5.89037560471066,0.));
#4707=CARTESIAN_POINT('',(-1.98012570815396,-1.92196317079901,6.));
#4708=CARTESIAN_POINT('Origin',(-5.93335250998519,-2.72454931910811,0.));
#4709=CARTESIAN_POINT('',(-5.02458355455784,-2.3072496837722,6.));
#4710=CARTESIAN_POINT('',(-6.20653880480254,-1.76258817211517,6.));
#4711=CARTESIAN_POINT('Origin',(-5.93335250998519,-2.72454931910811,6.));
#4712=CARTESIAN_POINT('',(-6.20653880480254,-1.76258817211517,-1.));
#4713=CARTESIAN_POINT('',(-6.20653880480254,-1.76258817211517,0.));
#4714=CARTESIAN_POINT('',(-5.02458355455784,-2.3072496837722,-1.));
#4715=CARTESIAN_POINT('Origin',(-5.93335250998519,-2.72454931910811,-1.));
#4716=CARTESIAN_POINT('',(-5.02458355455784,-2.3072496837722,0.));
#4717=CARTESIAN_POINT('Origin',(-8.13553012180811,-2.31040030805734,0.));
#4718=CARTESIAN_POINT('',(-8.13553012180811,-2.31040030805734,6.));
#4719=CARTESIAN_POINT('',(-4.06776506090406,-1.15520015402867,6.));
#4720=CARTESIAN_POINT('',(-8.13553012180811,-2.31040030805734,-1.));
#4721=CARTESIAN_POINT('',(-8.13553012180811,-2.31040030805734,0.));
#4722=CARTESIAN_POINT('',(-4.06776506090406,-1.15520015402867,-1.));
#4723=CARTESIAN_POINT('Origin',(-5.93335250998519,2.72454931910811,0.));
#4724=CARTESIAN_POINT('',(-5.02458355455784,2.3072496837722,-1.));
#4725=CARTESIAN_POINT('',(-6.20653880480254,1.76258817211517,-1.));
#4726=CARTESIAN_POINT('Origin',(-5.93335250998519,2.72454931910811,-1.));
#4727=CARTESIAN_POINT('',(-6.20653880480254,1.76258817211517,6.));
#4728=CARTESIAN_POINT('',(-6.20653880480254,1.76258817211517,0.));
#4729=CARTESIAN_POINT('',(-5.02458355455784,2.3072496837722,6.));
#4730=CARTESIAN_POINT('Origin',(-5.93335250998519,2.72454931910811,6.));
#4731=CARTESIAN_POINT('',(-5.02458355455784,2.3072496837722,0.));
#4732=CARTESIAN_POINT('Origin',(-5.30906357025402,1.50771516109694,0.));
#4733=CARTESIAN_POINT('',(-8.13553012180811,2.31040030805735,-1.));
#4734=CARTESIAN_POINT('',(-2.65453178512701,0.75385758054847,-1.));
#4735=CARTESIAN_POINT('',(-8.13553012180811,2.31040030805735,6.));
#4736=CARTESIAN_POINT('',(-8.13553012180811,2.31040030805735,0.));
#4737=CARTESIAN_POINT('',(-2.65453178512701,0.75385758054847,6.));
#4738=CARTESIAN_POINT('Origin',(-5.32620517920381,3.77615934370128,0.));
#4739=CARTESIAN_POINT('',(-4.51042861629926,3.1977921597985,6.));
#4740=CARTESIAN_POINT('',(-4.62971553586298,4.49372618847532,6.));
#4741=CARTESIAN_POINT('Origin',(-5.32620517920381,3.77615934370128,6.));
#4742=CARTESIAN_POINT('',(-4.62971553586298,4.49372618847532,-1.));
#4743=CARTESIAN_POINT('',(-4.62971553586298,4.49372618847532,0.));
#4744=CARTESIAN_POINT('',(-4.51042861629926,3.1977921597985,-1.));
#4745=CARTESIAN_POINT('Origin',(-5.32620517920381,3.77615934370128,-1.));
#4746=CARTESIAN_POINT('',(-4.51042861629926,3.1977921597985,0.));
#4747=CARTESIAN_POINT('Origin',(-6.06863042059311,5.89037560471066,0.));
#4748=CARTESIAN_POINT('',(-6.06863042059311,5.89037560471066,6.));
#4749=CARTESIAN_POINT('',(-3.03431521029656,2.94518780235533,6.));
#4750=CARTESIAN_POINT('',(-6.06863042059311,5.89037560471066,-1.));
#4751=CARTESIAN_POINT('',(-6.06863042059311,5.89037560471066,0.));
#4752=CARTESIAN_POINT('',(-3.03431521029656,2.94518780235533,-1.));
#4753=CARTESIAN_POINT('Origin',(-0.607147330781379,6.50070866280939,0.));
#4754=CARTESIAN_POINT('',(-0.514154938258576,5.5050418435707,-1.));
#4755=CARTESIAN_POINT('',(-1.57682326893955,6.25631436059049,-1.));
#4756=CARTESIAN_POINT('Origin',(-0.607147330781379,6.50070866280939,-1.));
#4757=CARTESIAN_POINT('',(-1.57682326893955,6.25631436059049,6.));
#4758=CARTESIAN_POINT('',(-1.57682326893955,6.25631436059049,0.));
#4759=CARTESIAN_POINT('',(-0.514154938258576,5.5050418435707,6.));
#4760=CARTESIAN_POINT('Origin',(-0.607147330781379,6.50070866280939,6.));
#4761=CARTESIAN_POINT('',(-0.514154938258576,5.5050418435707,0.));
#4762=CARTESIAN_POINT('Origin',(-1.34881215394611,5.35164150269497,0.));
#4763=CARTESIAN_POINT('',(-2.066899701215,8.20077591276801,-1.));
#4764=CARTESIAN_POINT('',(-0.674406076973057,2.67582075134748,-1.));
#4765=CARTESIAN_POINT('',(-2.066899701215,8.20077591276801,6.));
#4766=CARTESIAN_POINT('',(-2.066899701215,8.20077591276801,0.));
#4767=CARTESIAN_POINT('',(-0.674406076973057,2.67582075134748,6.));
#4768=CARTESIAN_POINT('Origin',(0.60714733078138,6.50070866280939,0.));
#4769=CARTESIAN_POINT('',(0.514154938258577,5.5050418435707,6.));
#4770=CARTESIAN_POINT('',(1.57682326893956,6.25631436059049,6.));
#4771=CARTESIAN_POINT('Origin',(0.60714733078138,6.50070866280939,6.));
#4772=CARTESIAN_POINT('',(1.57682326893956,6.25631436059049,-1.));
#4773=CARTESIAN_POINT('',(1.57682326893956,6.25631436059049,0.));
#4774=CARTESIAN_POINT('',(0.514154938258577,5.5050418435707,-1.));
#4775=CARTESIAN_POINT('Origin',(0.60714733078138,6.50070866280939,-1.));
#4776=CARTESIAN_POINT('',(0.514154938258577,5.5050418435707,0.));
#4777=CARTESIAN_POINT('Origin',(2.066899701215,8.20077591276801,0.));
#4778=CARTESIAN_POINT('',(2.066899701215,8.20077591276801,6.));
#4779=CARTESIAN_POINT('',(1.0334498506075,4.100387956384,6.));
#4780=CARTESIAN_POINT('',(2.066899701215,8.20077591276801,-1.));
#4781=CARTESIAN_POINT('',(2.066899701215,8.20077591276801,0.));
#4782=CARTESIAN_POINT('',(1.0334498506075,4.100387956384,-1.));
#4783=CARTESIAN_POINT('Origin',(5.32620517920381,3.77615934370128,0.));
#4784=CARTESIAN_POINT('',(4.51042861629926,3.1977921597985,-1.));
#4785=CARTESIAN_POINT('',(4.62971553586298,4.49372618847532,-1.));
#4786=CARTESIAN_POINT('Origin',(5.32620517920381,3.77615934370128,-1.));
#4787=CARTESIAN_POINT('',(4.62971553586298,4.49372618847532,6.));
#4788=CARTESIAN_POINT('',(4.62971553586298,4.49372618847532,0.));
#4789=CARTESIAN_POINT('',(4.51042861629926,3.1977921597985,6.));
#4790=CARTESIAN_POINT('Origin',(5.32620517920381,3.77615934370128,6.));
#4791=CARTESIAN_POINT('',(4.51042861629926,3.1977921597985,0.));
#4792=CARTESIAN_POINT('Origin',(3.96025141630791,3.84392634159803,0.));
#4793=CARTESIAN_POINT('',(6.06863042059311,5.89037560471066,-1.));
#4794=CARTESIAN_POINT('',(1.98012570815396,1.92196317079901,-1.));
#4795=CARTESIAN_POINT('',(6.06863042059311,5.89037560471066,6.));
#4796=CARTESIAN_POINT('',(6.06863042059311,5.89037560471066,0.));
#4797=CARTESIAN_POINT('',(1.98012570815396,1.92196317079901,6.));
#4798=CARTESIAN_POINT('Ctrl Pts',(6.60014603862877,-10.0218796774244,-3.75));
#4799=CARTESIAN_POINT('Ctrl Pts',(6.60014603862877,-10.0218796774244,12.75));
#4800=CARTESIAN_POINT('Ctrl Pts',(6.60293150665658,-10.0085665785717,-3.75));
#4801=CARTESIAN_POINT('Ctrl Pts',(6.60293150665658,-10.0085665785717,12.75));
#4802=CARTESIAN_POINT('Ctrl Pts',(6.60844558393655,-9.98194823089969,-3.75));
#4803=CARTESIAN_POINT('Ctrl Pts',(6.60844558393655,-9.98194823089969,12.75));
#4804=CARTESIAN_POINT('Ctrl Pts',(6.61654612354182,-9.94204425953052,-3.75));
#4805=CARTESIAN_POINT('Ctrl Pts',(6.61654612354182,-9.94204425953052,12.75));
#4806=CARTESIAN_POINT('Ctrl Pts',(6.62700557693595,-9.88888607996273,-3.75));
#4807=CARTESIAN_POINT('Ctrl Pts',(6.62700557693595,-9.88888607996273,12.75));
#4808=CARTESIAN_POINT('Ctrl Pts',(6.63951038900666,-9.82251725114899,-3.75));
#4809=CARTESIAN_POINT('Ctrl Pts',(6.63951038900666,-9.82251725114899,12.75));
#4810=CARTESIAN_POINT('Ctrl Pts',(6.65144464725858,-9.75622826411014,-3.75));
#4811=CARTESIAN_POINT('Ctrl Pts',(6.65144464725858,-9.75622826411014,12.75));
#4812=CARTESIAN_POINT('Ctrl Pts',(6.66280711160719,-9.69002090483258,-3.75));
#4813=CARTESIAN_POINT('Ctrl Pts',(6.66280711160719,-9.69002090483258,12.75));
#4814=CARTESIAN_POINT('Ctrl Pts',(6.6735964736696,-9.62389802250188,-3.75));
#4815=CARTESIAN_POINT('Ctrl Pts',(6.6735964736696,-9.62389802250188,12.75));
#4816=CARTESIAN_POINT('Ctrl Pts',(6.68381150859182,-9.55786385494287,-3.75));
#4817=CARTESIAN_POINT('Ctrl Pts',(6.68381150859182,-9.55786385494287,12.75));
#4818=CARTESIAN_POINT('Ctrl Pts',(6.69345108162376,-9.49192378686254,-3.75));
#4819=CARTESIAN_POINT('Ctrl Pts',(6.69345108162376,-9.49192378686254,12.75));
#4820=CARTESIAN_POINT('Ctrl Pts',(6.70251410760818,-9.42608392519667,-3.75));
#4821=CARTESIAN_POINT('Ctrl Pts',(6.70251410760818,-9.42608392519667,12.75));
#4822=CARTESIAN_POINT('Ctrl Pts',(6.71099953007123,-9.36035072031877,-3.75));
#4823=CARTESIAN_POINT('Ctrl Pts',(6.71099953007123,-9.36035072031877,12.75));
#4824=CARTESIAN_POINT('Ctrl Pts',(6.71890629646186,-9.29473060155551,-3.75));
#4825=CARTESIAN_POINT('Ctrl Pts',(6.71890629646186,-9.29473060155551,12.75));
#4826=CARTESIAN_POINT('Ctrl Pts',(6.72623333926845,-9.22922952332026,-3.75));
#4827=CARTESIAN_POINT('Ctrl Pts',(6.72623333926845,-9.22922952332026,12.75));
#4828=CARTESIAN_POINT('Ctrl Pts',(6.73297955932547,-9.16385288053588,-3.75));
#4829=CARTESIAN_POINT('Ctrl Pts',(6.73297955932547,-9.16385288053588,12.75));
#4830=CARTESIAN_POINT('Ctrl Pts',(6.73914381348522,-9.09860577342166,-3.75));
#4831=CARTESIAN_POINT('Ctrl Pts',(6.73914381348522,-9.09860577342166,12.75));
#4832=CARTESIAN_POINT('Ctrl Pts',(6.74472490424422,-9.03349318036199,-3.75));
#4833=CARTESIAN_POINT('Ctrl Pts',(6.74472490424422,-9.03349318036199,12.75));
#4834=CARTESIAN_POINT('Ctrl Pts',(6.74972157399228,-8.96852015431047,-3.75));
#4835=CARTESIAN_POINT('Ctrl Pts',(6.74972157399228,-8.96852015431047,12.75));
#4836=CARTESIAN_POINT('Ctrl Pts',(6.75413249860575,-8.90369203916218,-3.75));
#4837=CARTESIAN_POINT('Ctrl Pts',(6.75413249860575,-8.90369203916218,12.75));
#4838=CARTESIAN_POINT('Ctrl Pts',(6.75795629519249,-8.83901457377472,-3.75));
#4839=CARTESIAN_POINT('Ctrl Pts',(6.75795629519249,-8.83901457377472,12.75));
#4840=CARTESIAN_POINT('Ctrl Pts',(6.76119155448274,-8.77449374557665,-3.75));
#4841=CARTESIAN_POINT('Ctrl Pts',(6.76119155448274,-8.77449374557665,12.75));
#4842=CARTESIAN_POINT('Ctrl Pts',(6.76383687353852,-8.710135693856,-3.75));
#4843=CARTESIAN_POINT('Ctrl Pts',(6.76383687353852,-8.710135693856,12.75));
#4844=CARTESIAN_POINT('Ctrl Pts',(6.76589088878265,-8.64594659806299,-3.75));
#4845=CARTESIAN_POINT('Ctrl Pts',(6.76589088878265,-8.64594659806299,12.75));
#4846=CARTESIAN_POINT('Ctrl Pts',(6.76735232235634,-8.5819325577994,-3.75));
#4847=CARTESIAN_POINT('Ctrl Pts',(6.76735232235634,-8.5819325577994,12.75));
#4848=CARTESIAN_POINT('Ctrl Pts',(6.76822000004554,-8.51809951610774,-3.75));
#4849=CARTESIAN_POINT('Ctrl Pts',(6.76822000004554,-8.51809951610774,12.75));
#4850=CARTESIAN_POINT('Ctrl Pts',(6.76849272647565,-8.45445340444927,-3.75));
#4851=CARTESIAN_POINT('Ctrl Pts',(6.76849272647565,-8.45445340444927,12.75));
#4852=CARTESIAN_POINT('Ctrl Pts',(6.76816918165127,-8.39100025749019,-3.75));
#4853=CARTESIAN_POINT('Ctrl Pts',(6.76816918165127,-8.39100025749019,12.75));
#4854=CARTESIAN_POINT('Ctrl Pts',(6.76724781676281,-8.32774633509908,-3.75));
#4855=CARTESIAN_POINT('Ctrl Pts',(6.76724781676281,-8.32774633509908,12.75));
#4856=CARTESIAN_POINT('Ctrl Pts',(6.76572674650934,-8.26469824786603,-3.75));
#4857=CARTESIAN_POINT('Ctrl Pts',(6.76572674650934,-8.26469824786603,12.75));
#4858=CARTESIAN_POINT('Ctrl Pts',(6.76360366961639,-8.20186305794855,-3.75));
#4859=CARTESIAN_POINT('Ctrl Pts',(6.76360366961639,-8.20186305794855,12.75));
#4860=CARTESIAN_POINT('Ctrl Pts',(6.76087611417305,-8.13924806419108,-3.75));
#4861=CARTESIAN_POINT('Ctrl Pts',(6.76087611417305,-8.13924806419108,12.75));
#4862=CARTESIAN_POINT('Ctrl Pts',(6.75754166486089,-8.07686060726828,-3.75));
#4863=CARTESIAN_POINT('Ctrl Pts',(6.75754166486089,-8.07686060726828,12.75));
#4864=CARTESIAN_POINT('Ctrl Pts',(6.75359819949754,-8.01470786732019,-3.75));
#4865=CARTESIAN_POINT('Ctrl Pts',(6.75359819949754,-8.01470786732019,12.75));
#4866=CARTESIAN_POINT('Ctrl Pts',(6.7490441308376,-7.95279665937614,-3.75));
#4867=CARTESIAN_POINT('Ctrl Pts',(6.7490441308376,-7.95279665937614,12.75));
#4868=CARTESIAN_POINT('Ctrl Pts',(6.74387863902607,-7.89113323756913,-3.75));
#4869=CARTESIAN_POINT('Ctrl Pts',(6.74387863902607,-7.89113323756913,12.75));
#4870=CARTESIAN_POINT('Ctrl Pts',(6.73810106562748,-7.82972378407325,-3.75));
#4871=CARTESIAN_POINT('Ctrl Pts',(6.73810106562748,-7.82972378407325,12.75));
#4872=CARTESIAN_POINT('Ctrl Pts',(6.73171032576035,-7.76857488460784,-3.75));
#4873=CARTESIAN_POINT('Ctrl Pts',(6.73171032576035,-7.76857488460784,12.75));
#4874=CARTESIAN_POINT('Ctrl Pts',(6.72470431659336,-7.70769400824503,-3.75));
#4875=CARTESIAN_POINT('Ctrl Pts',(6.72470431659336,-7.70769400824503,12.75));
#4876=CARTESIAN_POINT('Ctrl Pts',(6.71707933277187,-7.6470899828899,-3.75));
#4877=CARTESIAN_POINT('Ctrl Pts',(6.71707933277187,-7.6470899828899,12.75));
#4878=CARTESIAN_POINT('Ctrl Pts',(6.70882947565317,-7.58677347699226,-3.75));
#4879=CARTESIAN_POINT('Ctrl Pts',(6.70882947565317,-7.58677347699226,12.75));
#4880=CARTESIAN_POINT('Ctrl Pts',(6.69994799095523,-7.52675593674633,-3.75));
#4881=CARTESIAN_POINT('Ctrl Pts',(6.69994799095523,-7.52675593674633,12.75));
#4882=CARTESIAN_POINT('Ctrl Pts',(6.69042862091103,-7.46704851290035,-3.75));
#4883=CARTESIAN_POINT('Ctrl Pts',(6.69042862091103,-7.46704851290035,12.75));
#4884=CARTESIAN_POINT('Ctrl Pts',(6.68026694677667,-7.40766099640558,-3.75));
#4885=CARTESIAN_POINT('Ctrl Pts',(6.68026694677667,-7.40766099640558,12.75));
#4886=CARTESIAN_POINT('Ctrl Pts',(6.66946176275797,-7.34860073021492,-3.75));
#4887=CARTESIAN_POINT('Ctrl Pts',(6.66946176275797,-7.34860073021492,12.75));
#4888=CARTESIAN_POINT('Ctrl Pts',(6.65801638970246,-7.28987157005224,-3.75));
#4889=CARTESIAN_POINT('Ctrl Pts',(6.65801638970246,-7.28987157005224,12.75));
#4890=CARTESIAN_POINT('Ctrl Pts',(6.64593535561052,-7.23147652896403,-3.75));
#4891=CARTESIAN_POINT('Ctrl Pts',(6.64593535561052,-7.23147652896403,12.75));
#4892=CARTESIAN_POINT('Ctrl Pts',(6.63322107969568,-7.17342042004756,-3.75));
#4893=CARTESIAN_POINT('Ctrl Pts',(6.63322107969568,-7.17342042004756,12.75));
#4894=CARTESIAN_POINT('Ctrl Pts',(6.6198706660591,-7.1157124131703,-3.75));
#4895=CARTESIAN_POINT('Ctrl Pts',(6.6198706660591,-7.1157124131703,12.75));
#4896=CARTESIAN_POINT('Ctrl Pts',(6.60587239994885,-7.05836882883084,-3.75));
#4897=CARTESIAN_POINT('Ctrl Pts',(6.60587239994885,-7.05836882883084,12.75));
#4898=CARTESIAN_POINT('Ctrl Pts',(6.5912030640433,-7.00141528186887,-3.75));
#4899=CARTESIAN_POINT('Ctrl Pts',(6.5912030640433,-7.00141528186887,12.75));
#4900=CARTESIAN_POINT('Ctrl Pts',(6.5758359541656,-6.94488033148854,-3.75));
#4901=CARTESIAN_POINT('Ctrl Pts',(6.5758359541656,-6.94488033148854,12.75));
#4902=CARTESIAN_POINT('Ctrl Pts',(6.55974857229919,-6.88878938806038,-3.75));
#4903=CARTESIAN_POINT('Ctrl Pts',(6.55974857229919,-6.88878938806038,12.75));
#4904=CARTESIAN_POINT('Ctrl Pts',(6.54292981913303,-6.83315901897032,-3.75));
#4905=CARTESIAN_POINT('Ctrl Pts',(6.54292981913303,-6.83315901897032,12.75));
#4906=CARTESIAN_POINT('Ctrl Pts',(6.52538888693355,-6.77798990345397,-3.75));
#4907=CARTESIAN_POINT('Ctrl Pts',(6.52538888693355,-6.77798990345397,12.75));
#4908=CARTESIAN_POINT('Ctrl Pts',(6.50715912032692,-6.72326378902152,-3.75));
#4909=CARTESIAN_POINT('Ctrl Pts',(6.50715912032692,-6.72326378902152,12.75));
#4910=CARTESIAN_POINT('Ctrl Pts',(6.48827758470622,-6.66895976394945,-3.75));
#4911=CARTESIAN_POINT('Ctrl Pts',(6.48827758470622,-6.66895976394945,12.75));
#4912=CARTESIAN_POINT('Ctrl Pts',(6.46876645798848,-6.61506907935741,-3.75));
#4913=CARTESIAN_POINT('Ctrl Pts',(6.46876645798848,-6.61506907935741,12.75));
#4914=CARTESIAN_POINT('Ctrl Pts',(6.44861636238489,-6.56160843323029,-3.75));
#4915=CARTESIAN_POINT('Ctrl Pts',(6.44861636238489,-6.56160843323029,12.75));
#4916=CARTESIAN_POINT('Ctrl Pts',(6.42776254872513,-6.50863892931077,-3.75));
#4917=CARTESIAN_POINT('Ctrl Pts',(6.42776254872513,-6.50863892931077,12.75));
#4918=CARTESIAN_POINT('Ctrl Pts',(6.40608444337877,-6.45626649182453,-3.75));
#4919=CARTESIAN_POINT('Ctrl Pts',(6.40608444337877,-6.45626649182453,12.75));
#4920=CARTESIAN_POINT('Ctrl Pts',(6.38345478017075,-6.404602962683,-3.75));
#4921=CARTESIAN_POINT('Ctrl Pts',(6.38345478017075,-6.404602962683,12.75));
#4922=CARTESIAN_POINT('Ctrl Pts',(6.35978286360965,-6.35373180396277,-3.75));
#4923=CARTESIAN_POINT('Ctrl Pts',(6.35978286360965,-6.35373180396277,12.75));
#4924=CARTESIAN_POINT('Ctrl Pts',(6.33505137069502,-6.30367904881887,-3.75));
#4925=CARTESIAN_POINT('Ctrl Pts',(6.33505137069502,-6.30367904881887,12.75));
#4926=CARTESIAN_POINT('Ctrl Pts',(6.309377504208,-6.25436463761971,-3.75));
#4927=CARTESIAN_POINT('Ctrl Pts',(6.309377504208,-6.25436463761971,12.75));
#4928=CARTESIAN_POINT('Ctrl Pts',(6.28297985424307,-6.20562962932065,-3.75));
#4929=CARTESIAN_POINT('Ctrl Pts',(6.28297985424307,-6.20562962932065,12.75));
#4930=CARTESIAN_POINT('Ctrl Pts',(6.25605474467853,-6.15733614814836,-3.75));
#4931=CARTESIAN_POINT('Ctrl Pts',(6.25605474467853,-6.15733614814836,12.75));
#4932=CARTESIAN_POINT('Ctrl Pts',(6.22866991793491,-6.10945353793714,-3.75));
#4933=CARTESIAN_POINT('Ctrl Pts',(6.22866991793491,-6.10945353793714,12.75));
#4934=CARTESIAN_POINT('Ctrl Pts',(6.20066685685754,-6.06213722636287,-3.75));
#4935=CARTESIAN_POINT('Ctrl Pts',(6.20066685685754,-6.06213722636287,12.75));
#4936=CARTESIAN_POINT('Ctrl Pts',(6.17151878498998,-6.01584411654484,-3.75));
#4937=CARTESIAN_POINT('Ctrl Pts',(6.17151878498998,-6.01584411654484,12.75));
#4938=CARTESIAN_POINT('Ctrl Pts',(6.14045331140033,-5.97123031969247,-3.75));
#4939=CARTESIAN_POINT('Ctrl Pts',(6.14045331140033,-5.97123031969247,12.75));
#4940=CARTESIAN_POINT('Ctrl Pts',(6.11342775487885,-5.9374218385168,-3.75));
#4941=CARTESIAN_POINT('Ctrl Pts',(6.11342775487885,-5.9374218385168,12.75));
#4942=CARTESIAN_POINT('Ctrl Pts',(6.09164867072823,-5.91336588048664,-3.75));
#4943=CARTESIAN_POINT('Ctrl Pts',(6.09164867072823,-5.91336588048664,12.75));
#4944=CARTESIAN_POINT('Ctrl Pts',(6.07642118935899,-5.89793753402585,-3.75));
#4945=CARTESIAN_POINT('Ctrl Pts',(6.07642118935899,-5.89793753402585,12.75));
#4946=CARTESIAN_POINT('Ctrl Pts',(6.06863042059311,-5.89037560471067,-3.75));
#4947=CARTESIAN_POINT('Ctrl Pts',(6.06863042059311,-5.89037560471067,12.75));
#4948=CARTESIAN_POINT('',(6.60014603862874,-10.0218796774245,-1.));
#4949=CARTESIAN_POINT('Ctrl Pts',(6.60014603862877,-10.0218796774244,-1.));
#4950=CARTESIAN_POINT('Ctrl Pts',(6.60293150665658,-10.0085665785717,-1.));
#4951=CARTESIAN_POINT('Ctrl Pts',(6.60844558393655,-9.98194823089969,-1.));
#4952=CARTESIAN_POINT('Ctrl Pts',(6.61654612354182,-9.94204425953052,-1.));
#4953=CARTESIAN_POINT('Ctrl Pts',(6.62700557693595,-9.88888607996273,-1.));
#4954=CARTESIAN_POINT('Ctrl Pts',(6.63951038900666,-9.82251725114899,-1.));
#4955=CARTESIAN_POINT('Ctrl Pts',(6.65144464725858,-9.75622826411014,-1.));
#4956=CARTESIAN_POINT('Ctrl Pts',(6.66280711160719,-9.69002090483258,-1.));
#4957=CARTESIAN_POINT('Ctrl Pts',(6.6735964736696,-9.62389802250188,-1.));
#4958=CARTESIAN_POINT('Ctrl Pts',(6.68381150859182,-9.55786385494287,-1.));
#4959=CARTESIAN_POINT('Ctrl Pts',(6.69345108162376,-9.49192378686254,-1.));
#4960=CARTESIAN_POINT('Ctrl Pts',(6.70251410760818,-9.42608392519667,-1.));
#4961=CARTESIAN_POINT('Ctrl Pts',(6.71099953007123,-9.36035072031877,-1.));
#4962=CARTESIAN_POINT('Ctrl Pts',(6.71890629646186,-9.29473060155551,-1.));
#4963=CARTESIAN_POINT('Ctrl Pts',(6.72623333926845,-9.22922952332026,-1.));
#4964=CARTESIAN_POINT('Ctrl Pts',(6.73297955932547,-9.16385288053588,-1.));
#4965=CARTESIAN_POINT('Ctrl Pts',(6.73914381348522,-9.09860577342166,-1.));
#4966=CARTESIAN_POINT('Ctrl Pts',(6.74472490424422,-9.03349318036199,-1.));
#4967=CARTESIAN_POINT('Ctrl Pts',(6.74972157399228,-8.96852015431047,-1.));
#4968=CARTESIAN_POINT('Ctrl Pts',(6.75413249860575,-8.90369203916218,-1.));
#4969=CARTESIAN_POINT('Ctrl Pts',(6.75795629519249,-8.83901457377472,-1.));
#4970=CARTESIAN_POINT('Ctrl Pts',(6.76119155448274,-8.77449374557665,-1.));
#4971=CARTESIAN_POINT('Ctrl Pts',(6.76383687353852,-8.710135693856,-1.));
#4972=CARTESIAN_POINT('Ctrl Pts',(6.76589088878265,-8.64594659806299,-1.));
#4973=CARTESIAN_POINT('Ctrl Pts',(6.76735232235634,-8.5819325577994,-1.));
#4974=CARTESIAN_POINT('Ctrl Pts',(6.76822000004554,-8.51809951610774,-1.));
#4975=CARTESIAN_POINT('Ctrl Pts',(6.76849272647565,-8.45445340444927,-1.));
#4976=CARTESIAN_POINT('Ctrl Pts',(6.76816918165127,-8.39100025749019,-1.));
#4977=CARTESIAN_POINT('Ctrl Pts',(6.76724781676281,-8.32774633509908,-1.));
#4978=CARTESIAN_POINT('Ctrl Pts',(6.76572674650934,-8.26469824786603,-1.));
#4979=CARTESIAN_POINT('Ctrl Pts',(6.76360366961639,-8.20186305794855,-1.));
#4980=CARTESIAN_POINT('Ctrl Pts',(6.76087611417305,-8.13924806419108,-1.));
#4981=CARTESIAN_POINT('Ctrl Pts',(6.75754166486089,-8.07686060726828,-1.));
#4982=CARTESIAN_POINT('Ctrl Pts',(6.75359819949754,-8.01470786732019,-1.));
#4983=CARTESIAN_POINT('Ctrl Pts',(6.7490441308376,-7.95279665937614,-1.));
#4984=CARTESIAN_POINT('Ctrl Pts',(6.74387863902607,-7.89113323756913,-1.));
#4985=CARTESIAN_POINT('Ctrl Pts',(6.73810106562748,-7.82972378407325,-1.));
#4986=CARTESIAN_POINT('Ctrl Pts',(6.73171032576035,-7.76857488460784,-1.));
#4987=CARTESIAN_POINT('Ctrl Pts',(6.72470431659336,-7.70769400824503,-1.));
#4988=CARTESIAN_POINT('Ctrl Pts',(6.71707933277187,-7.6470899828899,-1.));
#4989=CARTESIAN_POINT('Ctrl Pts',(6.70882947565317,-7.58677347699226,-1.));
#4990=CARTESIAN_POINT('Ctrl Pts',(6.69994799095523,-7.52675593674633,-1.));
#4991=CARTESIAN_POINT('Ctrl Pts',(6.69042862091103,-7.46704851290035,-1.));
#4992=CARTESIAN_POINT('Ctrl Pts',(6.68026694677667,-7.40766099640558,-1.));
#4993=CARTESIAN_POINT('Ctrl Pts',(6.66946176275797,-7.34860073021492,-1.));
#4994=CARTESIAN_POINT('Ctrl Pts',(6.65801638970246,-7.28987157005224,-1.));
#4995=CARTESIAN_POINT('Ctrl Pts',(6.64593535561052,-7.23147652896403,-1.));
#4996=CARTESIAN_POINT('Ctrl Pts',(6.63322107969568,-7.17342042004756,-1.));
#4997=CARTESIAN_POINT('Ctrl Pts',(6.6198706660591,-7.1157124131703,-1.));
#4998=CARTESIAN_POINT('Ctrl Pts',(6.60587239994885,-7.05836882883084,-1.));
#4999=CARTESIAN_POINT('Ctrl Pts',(6.5912030640433,-7.00141528186887,-1.));
#5000=CARTESIAN_POINT('Ctrl Pts',(6.5758359541656,-6.94488033148854,-1.));
#5001=CARTESIAN_POINT('Ctrl Pts',(6.55974857229919,-6.88878938806038,-1.));
#5002=CARTESIAN_POINT('Ctrl Pts',(6.54292981913303,-6.83315901897032,-1.));
#5003=CARTESIAN_POINT('Ctrl Pts',(6.52538888693355,-6.77798990345397,-1.));
#5004=CARTESIAN_POINT('Ctrl Pts',(6.50715912032692,-6.72326378902152,-1.));
#5005=CARTESIAN_POINT('Ctrl Pts',(6.48827758470622,-6.66895976394945,-1.));
#5006=CARTESIAN_POINT('Ctrl Pts',(6.46876645798848,-6.61506907935741,-1.));
#5007=CARTESIAN_POINT('Ctrl Pts',(6.44861636238489,-6.56160843323029,-1.));
#5008=CARTESIAN_POINT('Ctrl Pts',(6.42776254872513,-6.50863892931077,-1.));
#5009=CARTESIAN_POINT('Ctrl Pts',(6.40608444337877,-6.45626649182453,-1.));
#5010=CARTESIAN_POINT('Ctrl Pts',(6.38345478017075,-6.404602962683,-1.));
#5011=CARTESIAN_POINT('Ctrl Pts',(6.35978286360965,-6.35373180396277,-1.));
#5012=CARTESIAN_POINT('Ctrl Pts',(6.33505137069502,-6.30367904881887,-1.));
#5013=CARTESIAN_POINT('Ctrl Pts',(6.309377504208,-6.25436463761971,-1.));
#5014=CARTESIAN_POINT('Ctrl Pts',(6.28297985424307,-6.20562962932065,-1.));
#5015=CARTESIAN_POINT('Ctrl Pts',(6.25605474467853,-6.15733614814836,-1.));
#5016=CARTESIAN_POINT('Ctrl Pts',(6.22866991793491,-6.10945353793714,-1.));
#5017=CARTESIAN_POINT('Ctrl Pts',(6.20066685685754,-6.06213722636287,-1.));
#5018=CARTESIAN_POINT('Ctrl Pts',(6.17151878498998,-6.01584411654484,-1.));
#5019=CARTESIAN_POINT('Ctrl Pts',(6.14045331140033,-5.97123031969247,-1.));
#5020=CARTESIAN_POINT('Ctrl Pts',(6.11342775487885,-5.9374218385168,-1.));
#5021=CARTESIAN_POINT('Ctrl Pts',(6.09164867072823,-5.91336588048664,-1.));
#5022=CARTESIAN_POINT('Ctrl Pts',(6.07642118935899,-5.89793753402585,-1.));
#5023=CARTESIAN_POINT('Ctrl Pts',(6.06863042059311,-5.89037560471067,-1.));
#5024=CARTESIAN_POINT('',(6.60014603862874,-10.0218796774245,6.));
#5025=CARTESIAN_POINT('Ctrl Pts',(6.60014603862877,-10.0218796774244,6.));
#5026=CARTESIAN_POINT('Ctrl Pts',(6.60293150665658,-10.0085665785717,6.));
#5027=CARTESIAN_POINT('Ctrl Pts',(6.60844558393655,-9.98194823089969,6.));
#5028=CARTESIAN_POINT('Ctrl Pts',(6.61654612354182,-9.94204425953052,6.));
#5029=CARTESIAN_POINT('Ctrl Pts',(6.62700557693595,-9.88888607996273,6.));
#5030=CARTESIAN_POINT('Ctrl Pts',(6.63951038900666,-9.82251725114899,6.));
#5031=CARTESIAN_POINT('Ctrl Pts',(6.65144464725858,-9.75622826411014,6.));
#5032=CARTESIAN_POINT('Ctrl Pts',(6.66280711160719,-9.69002090483258,6.));
#5033=CARTESIAN_POINT('Ctrl Pts',(6.6735964736696,-9.62389802250188,6.));
#5034=CARTESIAN_POINT('Ctrl Pts',(6.68381150859182,-9.55786385494287,6.));
#5035=CARTESIAN_POINT('Ctrl Pts',(6.69345108162376,-9.49192378686254,6.));
#5036=CARTESIAN_POINT('Ctrl Pts',(6.70251410760818,-9.42608392519667,6.));
#5037=CARTESIAN_POINT('Ctrl Pts',(6.71099953007123,-9.36035072031877,6.));
#5038=CARTESIAN_POINT('Ctrl Pts',(6.71890629646186,-9.29473060155551,6.));
#5039=CARTESIAN_POINT('Ctrl Pts',(6.72623333926845,-9.22922952332026,6.));
#5040=CARTESIAN_POINT('Ctrl Pts',(6.73297955932547,-9.16385288053588,6.));
#5041=CARTESIAN_POINT('Ctrl Pts',(6.73914381348522,-9.09860577342166,6.));
#5042=CARTESIAN_POINT('Ctrl Pts',(6.74472490424422,-9.03349318036199,6.));
#5043=CARTESIAN_POINT('Ctrl Pts',(6.74972157399228,-8.96852015431047,6.));
#5044=CARTESIAN_POINT('Ctrl Pts',(6.75413249860575,-8.90369203916218,6.));
#5045=CARTESIAN_POINT('Ctrl Pts',(6.75795629519249,-8.83901457377472,6.));
#5046=CARTESIAN_POINT('Ctrl Pts',(6.76119155448274,-8.77449374557665,6.));
#5047=CARTESIAN_POINT('Ctrl Pts',(6.76383687353852,-8.710135693856,6.));
#5048=CARTESIAN_POINT('Ctrl Pts',(6.76589088878265,-8.64594659806299,6.));
#5049=CARTESIAN_POINT('Ctrl Pts',(6.76735232235634,-8.5819325577994,6.));
#5050=CARTESIAN_POINT('Ctrl Pts',(6.76822000004554,-8.51809951610774,6.));
#5051=CARTESIAN_POINT('Ctrl Pts',(6.76849272647565,-8.45445340444927,6.));
#5052=CARTESIAN_POINT('Ctrl Pts',(6.76816918165127,-8.39100025749019,6.));
#5053=CARTESIAN_POINT('Ctrl Pts',(6.76724781676281,-8.32774633509908,6.));
#5054=CARTESIAN_POINT('Ctrl Pts',(6.76572674650934,-8.26469824786603,6.));
#5055=CARTESIAN_POINT('Ctrl Pts',(6.76360366961639,-8.20186305794855,6.));
#5056=CARTESIAN_POINT('Ctrl Pts',(6.76087611417305,-8.13924806419108,6.));
#5057=CARTESIAN_POINT('Ctrl Pts',(6.75754166486089,-8.07686060726828,6.));
#5058=CARTESIAN_POINT('Ctrl Pts',(6.75359819949754,-8.01470786732019,6.));
#5059=CARTESIAN_POINT('Ctrl Pts',(6.7490441308376,-7.95279665937614,6.));
#5060=CARTESIAN_POINT('Ctrl Pts',(6.74387863902607,-7.89113323756913,6.));
#5061=CARTESIAN_POINT('Ctrl Pts',(6.73810106562748,-7.82972378407325,6.));
#5062=CARTESIAN_POINT('Ctrl Pts',(6.73171032576035,-7.76857488460784,6.));
#5063=CARTESIAN_POINT('Ctrl Pts',(6.72470431659336,-7.70769400824503,6.));
#5064=CARTESIAN_POINT('Ctrl Pts',(6.71707933277187,-7.6470899828899,6.));
#5065=CARTESIAN_POINT('Ctrl Pts',(6.70882947565317,-7.58677347699226,6.));
#5066=CARTESIAN_POINT('Ctrl Pts',(6.69994799095523,-7.52675593674633,6.));
#5067=CARTESIAN_POINT('Ctrl Pts',(6.69042862091103,-7.46704851290035,6.));
#5068=CARTESIAN_POINT('Ctrl Pts',(6.68026694677667,-7.40766099640558,6.));
#5069=CARTESIAN_POINT('Ctrl Pts',(6.66946176275797,-7.34860073021492,6.));
#5070=CARTESIAN_POINT('Ctrl Pts',(6.65801638970246,-7.28987157005224,6.));
#5071=CARTESIAN_POINT('Ctrl Pts',(6.64593535561052,-7.23147652896403,6.));
#5072=CARTESIAN_POINT('Ctrl Pts',(6.63322107969568,-7.17342042004756,6.));
#5073=CARTESIAN_POINT('Ctrl Pts',(6.6198706660591,-7.1157124131703,6.));
#5074=CARTESIAN_POINT('Ctrl Pts',(6.60587239994885,-7.05836882883084,6.));
#5075=CARTESIAN_POINT('Ctrl Pts',(6.5912030640433,-7.00141528186887,6.));
#5076=CARTESIAN_POINT('Ctrl Pts',(6.5758359541656,-6.94488033148854,6.));
#5077=CARTESIAN_POINT('Ctrl Pts',(6.55974857229919,-6.88878938806038,6.));
#5078=CARTESIAN_POINT('Ctrl Pts',(6.54292981913303,-6.83315901897032,6.));
#5079=CARTESIAN_POINT('Ctrl Pts',(6.52538888693355,-6.77798990345397,6.));
#5080=CARTESIAN_POINT('Ctrl Pts',(6.50715912032692,-6.72326378902152,6.));
#5081=CARTESIAN_POINT('Ctrl Pts',(6.48827758470622,-6.66895976394945,6.));
#5082=CARTESIAN_POINT('Ctrl Pts',(6.46876645798848,-6.61506907935741,6.));
#5083=CARTESIAN_POINT('Ctrl Pts',(6.44861636238489,-6.56160843323029,6.));
#5084=CARTESIAN_POINT('Ctrl Pts',(6.42776254872513,-6.50863892931077,6.));
#5085=CARTESIAN_POINT('Ctrl Pts',(6.40608444337877,-6.45626649182453,6.));
#5086=CARTESIAN_POINT('Ctrl Pts',(6.38345478017075,-6.404602962683,6.));
#5087=CARTESIAN_POINT('Ctrl Pts',(6.35978286360965,-6.35373180396277,6.));
#5088=CARTESIAN_POINT('Ctrl Pts',(6.33505137069502,-6.30367904881887,6.));
#5089=CARTESIAN_POINT('Ctrl Pts',(6.309377504208,-6.25436463761971,6.));
#5090=CARTESIAN_POINT('Ctrl Pts',(6.28297985424307,-6.20562962932065,6.));
#5091=CARTESIAN_POINT('Ctrl Pts',(6.25605474467853,-6.15733614814836,6.));
#5092=CARTESIAN_POINT('Ctrl Pts',(6.22866991793491,-6.10945353793714,6.));
#5093=CARTESIAN_POINT('Ctrl Pts',(6.20066685685754,-6.06213722636287,6.));
#5094=CARTESIAN_POINT('Ctrl Pts',(6.17151878498998,-6.01584411654484,6.));
#5095=CARTESIAN_POINT('Ctrl Pts',(6.14045331140033,-5.97123031969247,6.));
#5096=CARTESIAN_POINT('Ctrl Pts',(6.11342775487885,-5.9374218385168,6.));
#5097=CARTESIAN_POINT('Ctrl Pts',(6.09164867072823,-5.91336588048664,6.));
#5098=CARTESIAN_POINT('Ctrl Pts',(6.07642118935899,-5.89793753402585,6.));
#5099=CARTESIAN_POINT('Ctrl Pts',(6.06863042059311,-5.89037560471067,6.));
#5100=CARTESIAN_POINT('',(6.60014603862874,-10.0218796774245,0.));
#5101=CARTESIAN_POINT('Origin',(1.99840144432528E-13,-3.46133283549042E-13,
0.));
#5102=CARTESIAN_POINT('',(5.37912937500616,-10.726833976852,-1.));
#5103=CARTESIAN_POINT('Origin',(1.99840144432528E-13,-3.46133283549042E-13,
-1.));
#5104=CARTESIAN_POINT('',(5.37912937500616,-10.726833976852,6.));
#5105=CARTESIAN_POINT('Origin',(1.99840144432528E-13,-3.46133283549042E-13,
6.));
#5106=CARTESIAN_POINT('',(5.37912937500616,-10.726833976852,0.));
#5107=CARTESIAN_POINT('Ctrl Pts',(2.06689970121499,-8.20077591276801,-3.75));
#5108=CARTESIAN_POINT('Ctrl Pts',(2.06689970121499,-8.20077591276801,12.75));
#5109=CARTESIAN_POINT('Ctrl Pts',(2.06955313972063,-8.21130388109186,-3.75));
#5110=CARTESIAN_POINT('Ctrl Pts',(2.06955313972063,-8.21130388109186,12.75));
#5111=CARTESIAN_POINT('Ctrl Pts',(2.07530073900943,-8.23220544002367,-3.75));
#5112=CARTESIAN_POINT('Ctrl Pts',(2.07530073900943,-8.23220544002367,12.75));
#5113=CARTESIAN_POINT('Ctrl Pts',(2.08524426770062,-8.26309465918435,-3.75));
#5114=CARTESIAN_POINT('Ctrl Pts',(2.08524426770062,-8.26309465918435,12.75));
#5115=CARTESIAN_POINT('Ctrl Pts',(2.10101049300138,-8.3034037182712,-3.75));
#5116=CARTESIAN_POINT('Ctrl Pts',(2.10101049300138,-8.3034037182712,12.75));
#5117=CARTESIAN_POINT('Ctrl Pts',(2.12411443763998,-8.35261410600662,-3.75));
#5118=CARTESIAN_POINT('Ctrl Pts',(2.12411443763998,-8.35261410600662,12.75));
#5119=CARTESIAN_POINT('Ctrl Pts',(2.14963141082879,-8.40100363162428,-3.75));
#5120=CARTESIAN_POINT('Ctrl Pts',(2.14963141082879,-8.40100363162428,12.75));
#5121=CARTESIAN_POINT('Ctrl Pts',(2.17660700812681,-8.44891314968814,-3.75));
#5122=CARTESIAN_POINT('Ctrl Pts',(2.17660700812681,-8.44891314968814,12.75));
#5123=CARTESIAN_POINT('Ctrl Pts',(2.20438215159743,-8.49657041043196,-3.75));
#5124=CARTESIAN_POINT('Ctrl Pts',(2.20438215159743,-8.49657041043196,12.75));
#5125=CARTESIAN_POINT('Ctrl Pts',(2.23274297834755,-8.54403497990068,-3.75));
#5126=CARTESIAN_POINT('Ctrl Pts',(2.23274297834755,-8.54403497990068,12.75));
#5127=CARTESIAN_POINT('Ctrl Pts',(2.26174990860571,-8.59126351952005,-3.75));
#5128=CARTESIAN_POINT('Ctrl Pts',(2.26174990860571,-8.59126351952005,12.75));
#5129=CARTESIAN_POINT('Ctrl Pts',(2.29162050823335,-8.63815494571075,-3.75));
#5130=CARTESIAN_POINT('Ctrl Pts',(2.29162050823335,-8.63815494571075,12.75));
#5131=CARTESIAN_POINT('Ctrl Pts',(2.32260171926005,-8.68459942442029,-3.75));
#5132=CARTESIAN_POINT('Ctrl Pts',(2.32260171926005,-8.68459942442029,12.75));
#5133=CARTESIAN_POINT('Ctrl Pts',(2.35482147675117,-8.73053548487858,-3.75));
#5134=CARTESIAN_POINT('Ctrl Pts',(2.35482147675117,-8.73053548487858,12.75));
#5135=CARTESIAN_POINT('Ctrl Pts',(2.38824857383288,-8.77596511266658,-3.75));
#5136=CARTESIAN_POINT('Ctrl Pts',(2.38824857383288,-8.77596511266658,12.75));
#5137=CARTESIAN_POINT('Ctrl Pts',(2.4227653824809,-8.82092512134556,-3.75));
#5138=CARTESIAN_POINT('Ctrl Pts',(2.4227653824809,-8.82092512134556,12.75));
#5139=CARTESIAN_POINT('Ctrl Pts',(2.45821141167118,-8.86546980570045,-3.75));
#5140=CARTESIAN_POINT('Ctrl Pts',(2.45821141167118,-8.86546980570045,12.75));
#5141=CARTESIAN_POINT('Ctrl Pts',(2.4944346415182,-8.90965062344542,-3.75));
#5142=CARTESIAN_POINT('Ctrl Pts',(2.4944346415182,-8.90965062344542,12.75));
#5143=CARTESIAN_POINT('Ctrl Pts',(2.53134978004337,-8.95349309713545,-3.75));
#5144=CARTESIAN_POINT('Ctrl Pts',(2.53134978004337,-8.95349309713545,12.75));
#5145=CARTESIAN_POINT('Ctrl Pts',(2.56893767747318,-8.99699699918147,-3.75));
#5146=CARTESIAN_POINT('Ctrl Pts',(2.56893767747318,-8.99699699918147,12.75));
#5147=CARTESIAN_POINT('Ctrl Pts',(2.60721699951878,-9.0401474973841,-3.75));
#5148=CARTESIAN_POINT('Ctrl Pts',(2.60721699951878,-9.0401474973841,12.75));
#5149=CARTESIAN_POINT('Ctrl Pts',(2.64622438896051,-9.08292294803309,-3.75));
#5150=CARTESIAN_POINT('Ctrl Pts',(2.64622438896051,-9.08292294803309,12.75));
#5151=CARTESIAN_POINT('Ctrl Pts',(2.68599232523133,-9.12530360007999,-3.75));
#5152=CARTESIAN_POINT('Ctrl Pts',(2.68599232523133,-9.12530360007999,12.75));
#5153=CARTESIAN_POINT('Ctrl Pts',(2.72652481622915,-9.16728115317077,-3.75));
#5154=CARTESIAN_POINT('Ctrl Pts',(2.72652481622915,-9.16728115317077,12.75));
#5155=CARTESIAN_POINT('Ctrl Pts',(2.76780196452136,-9.20885693589776,-3.75));
#5156=CARTESIAN_POINT('Ctrl Pts',(2.76780196452136,-9.20885693589776,12.75));
#5157=CARTESIAN_POINT('Ctrl Pts',(2.80979051507329,-9.25003772692961,-3.75));
#5158=CARTESIAN_POINT('Ctrl Pts',(2.80979051507329,-9.25003772692961,12.75));
#5159=CARTESIAN_POINT('Ctrl Pts',(2.85245238280019,-9.29083237315975,-3.75));
#5160=CARTESIAN_POINT('Ctrl Pts',(2.85245238280019,-9.29083237315975,12.75));
#5161=CARTESIAN_POINT('Ctrl Pts',(2.89575377593937,-9.33124817395869,-3.75));
#5162=CARTESIAN_POINT('Ctrl Pts',(2.89575377593937,-9.33124817395869,12.75));
#5163=CARTESIAN_POINT('Ctrl Pts',(2.93967470314849,-9.3712871143499,-3.75));
#5164=CARTESIAN_POINT('Ctrl Pts',(2.93967470314849,-9.3712871143499,12.75));
#5165=CARTESIAN_POINT('Ctrl Pts',(2.98420577513995,-9.4109471173216,-3.75));
#5166=CARTESIAN_POINT('Ctrl Pts',(2.98420577513995,-9.4109471173216,12.75));
#5167=CARTESIAN_POINT('Ctrl Pts',(3.029344033256,-9.45022368122481,-3.75));
#5168=CARTESIAN_POINT('Ctrl Pts',(3.029344033256,-9.45022368122481,12.75));
#5169=CARTESIAN_POINT('Ctrl Pts',(3.07508913212203,-9.4891113781729,-3.75));
#5170=CARTESIAN_POINT('Ctrl Pts',(3.07508913212203,-9.4891113781729,12.75));
#5171=CARTESIAN_POINT('Ctrl Pts',(3.12143939300698,-9.52760540436562,-3.75));
#5172=CARTESIAN_POINT('Ctrl Pts',(3.12143939300698,-9.52760540436562,12.75));
#5173=CARTESIAN_POINT('Ctrl Pts',(3.16838785383003,-9.56570313257491,-3.75));
#5174=CARTESIAN_POINT('Ctrl Pts',(3.16838785383003,-9.56570313257491,12.75));
#5175=CARTESIAN_POINT('Ctrl Pts',(3.21592382600669,-9.60340349406962,-3.75));
#5176=CARTESIAN_POINT('Ctrl Pts',(3.21592382600669,-9.60340349406962,12.75));
#5177=CARTESIAN_POINT('Ctrl Pts',(3.26403452382221,-9.64070633286082,-3.75));
#5178=CARTESIAN_POINT('Ctrl Pts',(3.26403452382221,-9.64070633286082,12.75));
#5179=CARTESIAN_POINT('Ctrl Pts',(3.31270665744061,-9.67761177523124,-3.75));
#5180=CARTESIAN_POINT('Ctrl Pts',(3.31270665744061,-9.67761177523124,12.75));
#5181=CARTESIAN_POINT('Ctrl Pts',(3.36192803839196,-9.71411959533041,-3.75));
#5182=CARTESIAN_POINT('Ctrl Pts',(3.36192803839196,-9.71411959533041,12.75));
#5183=CARTESIAN_POINT('Ctrl Pts',(3.4116891688089,-9.75022858813702,-3.75));
#5184=CARTESIAN_POINT('Ctrl Pts',(3.4116891688089,-9.75022858813702,12.75));
#5185=CARTESIAN_POINT('Ctrl Pts',(3.46198252886956,-9.78593684022038,-3.75));
#5186=CARTESIAN_POINT('Ctrl Pts',(3.46198252886956,-9.78593684022038,12.75));
#5187=CARTESIAN_POINT('Ctrl Pts',(3.51280187273294,-9.8212419982557,-3.75));
#5188=CARTESIAN_POINT('Ctrl Pts',(3.51280187273294,-9.8212419982557,12.75));
#5189=CARTESIAN_POINT('Ctrl Pts',(3.5641415172615,-9.85614154137781,-3.75));
#5190=CARTESIAN_POINT('Ctrl Pts',(3.5641415172615,-9.85614154137781,12.75));
#5191=CARTESIAN_POINT('Ctrl Pts',(3.61599563628968,-9.89063305253546,-3.75));
#5192=CARTESIAN_POINT('Ctrl Pts',(3.61599563628968,-9.89063305253546,12.75));
#5193=CARTESIAN_POINT('Ctrl Pts',(3.66835753420625,-9.92471449880883,-3.75));
#5194=CARTESIAN_POINT('Ctrl Pts',(3.66835753420625,-9.92471449880883,12.75));
#5195=CARTESIAN_POINT('Ctrl Pts',(3.72121993173636,-9.95838412799173,-3.75));
#5196=CARTESIAN_POINT('Ctrl Pts',(3.72121993173636,-9.95838412799173,12.75));
#5197=CARTESIAN_POINT('Ctrl Pts',(3.77457526401003,-9.99164036147395,-3.75));
#5198=CARTESIAN_POINT('Ctrl Pts',(3.77457526401003,-9.99164036147395,12.75));
#5199=CARTESIAN_POINT('Ctrl Pts',(3.82841597408714,-10.0244816905709,-3.75));
#5200=CARTESIAN_POINT('Ctrl Pts',(3.82841597408714,-10.0244816905709,12.75));
#5201=CARTESIAN_POINT('Ctrl Pts',(3.88273479532262,-10.056906577166,-3.75));
#5202=CARTESIAN_POINT('Ctrl Pts',(3.88273479532262,-10.056906577166,12.75));
#5203=CARTESIAN_POINT('Ctrl Pts',(3.93752506012706,-10.0889133486827,-3.75));
#5204=CARTESIAN_POINT('Ctrl Pts',(3.93752506012706,-10.0889133486827,12.75));
#5205=CARTESIAN_POINT('Ctrl Pts',(3.99278057289045,-10.1205002164952,-3.75));
#5206=CARTESIAN_POINT('Ctrl Pts',(3.99278057289045,-10.1205002164952,12.75));
#5207=CARTESIAN_POINT('Ctrl Pts',(4.04849544744086,-10.1516653064199,-3.75));
#5208=CARTESIAN_POINT('Ctrl Pts',(4.04849544744086,-10.1516653064199,12.75));
#5209=CARTESIAN_POINT('Ctrl Pts',(4.10466394929485,-10.1824066879509,-3.75));
#5210=CARTESIAN_POINT('Ctrl Pts',(4.10466394929485,-10.1824066879509,12.75));
#5211=CARTESIAN_POINT('Ctrl Pts',(4.16128034451961,-10.2127224064663,-3.75));
#5212=CARTESIAN_POINT('Ctrl Pts',(4.16128034451961,-10.2127224064663,12.75));
#5213=CARTESIAN_POINT('Ctrl Pts',(4.21833871177566,-10.2426105188232,-3.75));
#5214=CARTESIAN_POINT('Ctrl Pts',(4.21833871177566,-10.2426105188232,12.75));
#5215=CARTESIAN_POINT('Ctrl Pts',(4.27583301771352,-10.272069116189,-3.75));
#5216=CARTESIAN_POINT('Ctrl Pts',(4.27583301771352,-10.272069116189,12.75));
#5217=CARTESIAN_POINT('Ctrl Pts',(4.33375724408483,-10.3010963438997,-3.75));
#5218=CARTESIAN_POINT('Ctrl Pts',(4.33375724408483,-10.3010963438997,12.75));
#5219=CARTESIAN_POINT('Ctrl Pts',(4.39210550098944,-10.3296904287044,-3.75));
#5220=CARTESIAN_POINT('Ctrl Pts',(4.39210550098944,-10.3296904287044,12.75));
#5221=CARTESIAN_POINT('Ctrl Pts',(4.45087212698484,-10.3578496987941,-3.75));
#5222=CARTESIAN_POINT('Ctrl Pts',(4.45087212698484,-10.3578496987941,12.75));
#5223=CARTESIAN_POINT('Ctrl Pts',(4.51005183206029,-10.3855726289458,-3.75));
#5224=CARTESIAN_POINT('Ctrl Pts',(4.51005183206029,-10.3855726289458,12.75));
#5225=CARTESIAN_POINT('Ctrl Pts',(4.56963961142453,-10.4128577818052,-3.75));
#5226=CARTESIAN_POINT('Ctrl Pts',(4.56963961142453,-10.4128577818052,12.75));
#5227=CARTESIAN_POINT('Ctrl Pts',(4.62963055491845,-10.4397037052485,-3.75));
#5228=CARTESIAN_POINT('Ctrl Pts',(4.62963055491845,-10.4397037052485,12.75));
#5229=CARTESIAN_POINT('Ctrl Pts',(4.69001967404874,-10.466108839161,-3.75));
#5230=CARTESIAN_POINT('Ctrl Pts',(4.69001967404874,-10.466108839161,12.75));
#5231=CARTESIAN_POINT('Ctrl Pts',(4.75080174709239,-10.4920714379865,-3.75));
#5232=CARTESIAN_POINT('Ctrl Pts',(4.75080174709239,-10.4920714379865,12.75));
#5233=CARTESIAN_POINT('Ctrl Pts',(4.81197108362034,-10.5175894490106,-3.75));
#5234=CARTESIAN_POINT('Ctrl Pts',(4.81197108362034,-10.5175894490106,12.75));
#5235=CARTESIAN_POINT('Ctrl Pts',(4.87352158939685,-10.5426605691059,-3.75));
#5236=CARTESIAN_POINT('Ctrl Pts',(4.87352158939685,-10.5426605691059,12.75));
#5237=CARTESIAN_POINT('Ctrl Pts',(4.93544714999767,-10.5672824880187,-3.75));
#5238=CARTESIAN_POINT('Ctrl Pts',(4.93544714999767,-10.5672824880187,12.75));
#5239=CARTESIAN_POINT('Ctrl Pts',(4.99774193408263,-10.5914530920551,-3.75));
#5240=CARTESIAN_POINT('Ctrl Pts',(4.99774193408263,-10.5914530920551,12.75));
#5241=CARTESIAN_POINT('Ctrl Pts',(5.06040071098368,-10.6151706715837,-3.75));
#5242=CARTESIAN_POINT('Ctrl Pts',(5.06040071098368,-10.6151706715837,12.75));
#5243=CARTESIAN_POINT('Ctrl Pts',(5.12341919820983,-10.638434168447,-3.75));
#5244=CARTESIAN_POINT('Ctrl Pts',(5.12341919820983,-10.638434168447,12.75));
#5245=CARTESIAN_POINT('Ctrl Pts',(5.18679427410257,-10.661243291145,-3.75));
#5246=CARTESIAN_POINT('Ctrl Pts',(5.18679427410257,-10.661243291145,12.75));
#5247=CARTESIAN_POINT('Ctrl Pts',(5.25052377191005,-10.6835982206291,-3.75));
#5248=CARTESIAN_POINT('Ctrl Pts',(5.25052377191005,-10.6835982206291,12.75));
#5249=CARTESIAN_POINT('Ctrl Pts',(5.30178983253175,-10.7011191580639,-3.75));
#5250=CARTESIAN_POINT('Ctrl Pts',(5.30178983253175,-10.7011191580639,12.75));
#5251=CARTESIAN_POINT('Ctrl Pts',(5.34039795525197,-10.714055870666,-3.75));
#5252=CARTESIAN_POINT('Ctrl Pts',(5.34039795525197,-10.714055870666,12.75));
#5253=CARTESIAN_POINT('Ctrl Pts',(5.3662071591827,-10.7225897134991,-3.75));
#5254=CARTESIAN_POINT('Ctrl Pts',(5.3662071591827,-10.7225897134991,12.75));
#5255=CARTESIAN_POINT('Ctrl Pts',(5.37912937500616,-10.726833976852,-3.75));
#5256=CARTESIAN_POINT('Ctrl Pts',(5.37912937500616,-10.726833976852,12.75));
#5257=CARTESIAN_POINT('Ctrl Pts',(2.06689970121499,-8.20077591276801,-1.));
#5258=CARTESIAN_POINT('Ctrl Pts',(2.06955313972063,-8.21130388109186,-1.));
#5259=CARTESIAN_POINT('Ctrl Pts',(2.07530073900943,-8.23220544002367,-1.));
#5260=CARTESIAN_POINT('Ctrl Pts',(2.08524426770062,-8.26309465918435,-1.));
#5261=CARTESIAN_POINT('Ctrl Pts',(2.10101049300138,-8.3034037182712,-1.));
#5262=CARTESIAN_POINT('Ctrl Pts',(2.12411443763998,-8.35261410600662,-1.));
#5263=CARTESIAN_POINT('Ctrl Pts',(2.14963141082879,-8.40100363162428,-1.));
#5264=CARTESIAN_POINT('Ctrl Pts',(2.17660700812681,-8.44891314968814,-1.));
#5265=CARTESIAN_POINT('Ctrl Pts',(2.20438215159743,-8.49657041043196,-1.));
#5266=CARTESIAN_POINT('Ctrl Pts',(2.23274297834755,-8.54403497990068,-1.));
#5267=CARTESIAN_POINT('Ctrl Pts',(2.26174990860571,-8.59126351952005,-1.));
#5268=CARTESIAN_POINT('Ctrl Pts',(2.29162050823335,-8.63815494571075,-1.));
#5269=CARTESIAN_POINT('Ctrl Pts',(2.32260171926005,-8.68459942442029,-1.));
#5270=CARTESIAN_POINT('Ctrl Pts',(2.35482147675117,-8.73053548487858,-1.));
#5271=CARTESIAN_POINT('Ctrl Pts',(2.38824857383288,-8.77596511266658,-1.));
#5272=CARTESIAN_POINT('Ctrl Pts',(2.4227653824809,-8.82092512134556,-1.));
#5273=CARTESIAN_POINT('Ctrl Pts',(2.45821141167118,-8.86546980570045,-1.));
#5274=CARTESIAN_POINT('Ctrl Pts',(2.4944346415182,-8.90965062344542,-1.));
#5275=CARTESIAN_POINT('Ctrl Pts',(2.53134978004337,-8.95349309713545,-1.));
#5276=CARTESIAN_POINT('Ctrl Pts',(2.56893767747318,-8.99699699918147,-1.));
#5277=CARTESIAN_POINT('Ctrl Pts',(2.60721699951878,-9.0401474973841,-1.));
#5278=CARTESIAN_POINT('Ctrl Pts',(2.64622438896051,-9.08292294803309,-1.));
#5279=CARTESIAN_POINT('Ctrl Pts',(2.68599232523133,-9.12530360007999,-1.));
#5280=CARTESIAN_POINT('Ctrl Pts',(2.72652481622915,-9.16728115317077,-1.));
#5281=CARTESIAN_POINT('Ctrl Pts',(2.76780196452136,-9.20885693589776,-1.));
#5282=CARTESIAN_POINT('Ctrl Pts',(2.80979051507329,-9.25003772692961,-1.));
#5283=CARTESIAN_POINT('Ctrl Pts',(2.85245238280019,-9.29083237315975,-1.));
#5284=CARTESIAN_POINT('Ctrl Pts',(2.89575377593937,-9.33124817395869,-1.));
#5285=CARTESIAN_POINT('Ctrl Pts',(2.93967470314849,-9.3712871143499,-1.));
#5286=CARTESIAN_POINT('Ctrl Pts',(2.98420577513995,-9.4109471173216,-1.));
#5287=CARTESIAN_POINT('Ctrl Pts',(3.029344033256,-9.45022368122481,-1.));
#5288=CARTESIAN_POINT('Ctrl Pts',(3.07508913212203,-9.4891113781729,-1.));
#5289=CARTESIAN_POINT('Ctrl Pts',(3.12143939300698,-9.52760540436562,-1.));
#5290=CARTESIAN_POINT('Ctrl Pts',(3.16838785383003,-9.56570313257491,-1.));
#5291=CARTESIAN_POINT('Ctrl Pts',(3.21592382600669,-9.60340349406962,-1.));
#5292=CARTESIAN_POINT('Ctrl Pts',(3.26403452382221,-9.64070633286082,-1.));
#5293=CARTESIAN_POINT('Ctrl Pts',(3.31270665744061,-9.67761177523124,-1.));
#5294=CARTESIAN_POINT('Ctrl Pts',(3.36192803839196,-9.71411959533041,-1.));
#5295=CARTESIAN_POINT('Ctrl Pts',(3.4116891688089,-9.75022858813702,-1.));
#5296=CARTESIAN_POINT('Ctrl Pts',(3.46198252886956,-9.78593684022038,-1.));
#5297=CARTESIAN_POINT('Ctrl Pts',(3.51280187273294,-9.8212419982557,-1.));
#5298=CARTESIAN_POINT('Ctrl Pts',(3.5641415172615,-9.85614154137781,-1.));
#5299=CARTESIAN_POINT('Ctrl Pts',(3.61599563628968,-9.89063305253546,-1.));
#5300=CARTESIAN_POINT('Ctrl Pts',(3.66835753420625,-9.92471449880883,-1.));
#5301=CARTESIAN_POINT('Ctrl Pts',(3.72121993173636,-9.95838412799173,-1.));
#5302=CARTESIAN_POINT('Ctrl Pts',(3.77457526401003,-9.99164036147395,-1.));
#5303=CARTESIAN_POINT('Ctrl Pts',(3.82841597408714,-10.0244816905709,-1.));
#5304=CARTESIAN_POINT('Ctrl Pts',(3.88273479532262,-10.056906577166,-1.));
#5305=CARTESIAN_POINT('Ctrl Pts',(3.93752506012706,-10.0889133486827,-1.));
#5306=CARTESIAN_POINT('Ctrl Pts',(3.99278057289045,-10.1205002164952,-1.));
#5307=CARTESIAN_POINT('Ctrl Pts',(4.04849544744086,-10.1516653064199,-1.));
#5308=CARTESIAN_POINT('Ctrl Pts',(4.10466394929485,-10.1824066879509,-1.));
#5309=CARTESIAN_POINT('Ctrl Pts',(4.16128034451961,-10.2127224064663,-1.));
#5310=CARTESIAN_POINT('Ctrl Pts',(4.21833871177566,-10.2426105188232,-1.));
#5311=CARTESIAN_POINT('Ctrl Pts',(4.27583301771352,-10.272069116189,-1.));
#5312=CARTESIAN_POINT('Ctrl Pts',(4.33375724408483,-10.3010963438997,-1.));
#5313=CARTESIAN_POINT('Ctrl Pts',(4.39210550098944,-10.3296904287044,-1.));
#5314=CARTESIAN_POINT('Ctrl Pts',(4.45087212698484,-10.3578496987941,-1.));
#5315=CARTESIAN_POINT('Ctrl Pts',(4.51005183206029,-10.3855726289458,-1.));
#5316=CARTESIAN_POINT('Ctrl Pts',(4.56963961142453,-10.4128577818052,-1.));
#5317=CARTESIAN_POINT('Ctrl Pts',(4.62963055491845,-10.4397037052485,-1.));
#5318=CARTESIAN_POINT('Ctrl Pts',(4.69001967404874,-10.466108839161,-1.));
#5319=CARTESIAN_POINT('Ctrl Pts',(4.75080174709239,-10.4920714379865,-1.));
#5320=CARTESIAN_POINT('Ctrl Pts',(4.81197108362034,-10.5175894490106,-1.));
#5321=CARTESIAN_POINT('Ctrl Pts',(4.87352158939685,-10.5426605691059,-1.));
#5322=CARTESIAN_POINT('Ctrl Pts',(4.93544714999767,-10.5672824880187,-1.));
#5323=CARTESIAN_POINT('Ctrl Pts',(4.99774193408263,-10.5914530920551,-1.));
#5324=CARTESIAN_POINT('Ctrl Pts',(5.06040071098368,-10.6151706715837,-1.));
#5325=CARTESIAN_POINT('Ctrl Pts',(5.12341919820983,-10.638434168447,-1.));
#5326=CARTESIAN_POINT('Ctrl Pts',(5.18679427410257,-10.661243291145,-1.));
#5327=CARTESIAN_POINT('Ctrl Pts',(5.25052377191005,-10.6835982206291,-1.));
#5328=CARTESIAN_POINT('Ctrl Pts',(5.30178983253175,-10.7011191580639,-1.));
#5329=CARTESIAN_POINT('Ctrl Pts',(5.34039795525197,-10.714055870666,-1.));
#5330=CARTESIAN_POINT('Ctrl Pts',(5.3662071591827,-10.7225897134991,-1.));
#5331=CARTESIAN_POINT('Ctrl Pts',(5.37912937500616,-10.726833976852,-1.));
#5332=CARTESIAN_POINT('Ctrl Pts',(2.06689970121499,-8.20077591276801,6.));
#5333=CARTESIAN_POINT('Ctrl Pts',(2.06955313972063,-8.21130388109186,6.));
#5334=CARTESIAN_POINT('Ctrl Pts',(2.07530073900943,-8.23220544002367,6.));
#5335=CARTESIAN_POINT('Ctrl Pts',(2.08524426770062,-8.26309465918435,6.));
#5336=CARTESIAN_POINT('Ctrl Pts',(2.10101049300138,-8.3034037182712,6.));
#5337=CARTESIAN_POINT('Ctrl Pts',(2.12411443763998,-8.35261410600662,6.));
#5338=CARTESIAN_POINT('Ctrl Pts',(2.14963141082879,-8.40100363162428,6.));
#5339=CARTESIAN_POINT('Ctrl Pts',(2.17660700812681,-8.44891314968814,6.));
#5340=CARTESIAN_POINT('Ctrl Pts',(2.20438215159743,-8.49657041043196,6.));
#5341=CARTESIAN_POINT('Ctrl Pts',(2.23274297834755,-8.54403497990068,6.));
#5342=CARTESIAN_POINT('Ctrl Pts',(2.26174990860571,-8.59126351952005,6.));
#5343=CARTESIAN_POINT('Ctrl Pts',(2.29162050823335,-8.63815494571075,6.));
#5344=CARTESIAN_POINT('Ctrl Pts',(2.32260171926005,-8.68459942442029,6.));
#5345=CARTESIAN_POINT('Ctrl Pts',(2.35482147675117,-8.73053548487858,6.));
#5346=CARTESIAN_POINT('Ctrl Pts',(2.38824857383288,-8.77596511266658,6.));
#5347=CARTESIAN_POINT('Ctrl Pts',(2.4227653824809,-8.82092512134556,6.));
#5348=CARTESIAN_POINT('Ctrl Pts',(2.45821141167118,-8.86546980570045,6.));
#5349=CARTESIAN_POINT('Ctrl Pts',(2.4944346415182,-8.90965062344542,6.));
#5350=CARTESIAN_POINT('Ctrl Pts',(2.53134978004337,-8.95349309713545,6.));
#5351=CARTESIAN_POINT('Ctrl Pts',(2.56893767747318,-8.99699699918147,6.));
#5352=CARTESIAN_POINT('Ctrl Pts',(2.60721699951878,-9.0401474973841,6.));
#5353=CARTESIAN_POINT('Ctrl Pts',(2.64622438896051,-9.08292294803309,6.));
#5354=CARTESIAN_POINT('Ctrl Pts',(2.68599232523133,-9.12530360007999,6.));
#5355=CARTESIAN_POINT('Ctrl Pts',(2.72652481622915,-9.16728115317077,6.));
#5356=CARTESIAN_POINT('Ctrl Pts',(2.76780196452136,-9.20885693589776,6.));
#5357=CARTESIAN_POINT('Ctrl Pts',(2.80979051507329,-9.25003772692961,6.));
#5358=CARTESIAN_POINT('Ctrl Pts',(2.85245238280019,-9.29083237315975,6.));
#5359=CARTESIAN_POINT('Ctrl Pts',(2.89575377593937,-9.33124817395869,6.));
#5360=CARTESIAN_POINT('Ctrl Pts',(2.93967470314849,-9.3712871143499,6.));
#5361=CARTESIAN_POINT('Ctrl Pts',(2.98420577513995,-9.4109471173216,6.));
#5362=CARTESIAN_POINT('Ctrl Pts',(3.029344033256,-9.45022368122481,6.));
#5363=CARTESIAN_POINT('Ctrl Pts',(3.07508913212203,-9.4891113781729,6.));
#5364=CARTESIAN_POINT('Ctrl Pts',(3.12143939300698,-9.52760540436562,6.));
#5365=CARTESIAN_POINT('Ctrl Pts',(3.16838785383003,-9.56570313257491,6.));
#5366=CARTESIAN_POINT('Ctrl Pts',(3.21592382600669,-9.60340349406962,6.));
#5367=CARTESIAN_POINT('Ctrl Pts',(3.26403452382221,-9.64070633286082,6.));
#5368=CARTESIAN_POINT('Ctrl Pts',(3.31270665744061,-9.67761177523124,6.));
#5369=CARTESIAN_POINT('Ctrl Pts',(3.36192803839196,-9.71411959533041,6.));
#5370=CARTESIAN_POINT('Ctrl Pts',(3.4116891688089,-9.75022858813702,6.));
#5371=CARTESIAN_POINT('Ctrl Pts',(3.46198252886956,-9.78593684022038,6.));
#5372=CARTESIAN_POINT('Ctrl Pts',(3.51280187273294,-9.8212419982557,6.));
#5373=CARTESIAN_POINT('Ctrl Pts',(3.5641415172615,-9.85614154137781,6.));
#5374=CARTESIAN_POINT('Ctrl Pts',(3.61599563628968,-9.89063305253546,6.));
#5375=CARTESIAN_POINT('Ctrl Pts',(3.66835753420625,-9.92471449880883,6.));
#5376=CARTESIAN_POINT('Ctrl Pts',(3.72121993173636,-9.95838412799173,6.));
#5377=CARTESIAN_POINT('Ctrl Pts',(3.77457526401003,-9.99164036147395,6.));
#5378=CARTESIAN_POINT('Ctrl Pts',(3.82841597408714,-10.0244816905709,6.));
#5379=CARTESIAN_POINT('Ctrl Pts',(3.88273479532262,-10.056906577166,6.));
#5380=CARTESIAN_POINT('Ctrl Pts',(3.93752506012706,-10.0889133486827,6.));
#5381=CARTESIAN_POINT('Ctrl Pts',(3.99278057289045,-10.1205002164952,6.));
#5382=CARTESIAN_POINT('Ctrl Pts',(4.04849544744086,-10.1516653064199,6.));
#5383=CARTESIAN_POINT('Ctrl Pts',(4.10466394929485,-10.1824066879509,6.));
#5384=CARTESIAN_POINT('Ctrl Pts',(4.16128034451961,-10.2127224064663,6.));
#5385=CARTESIAN_POINT('Ctrl Pts',(4.21833871177566,-10.2426105188232,6.));
#5386=CARTESIAN_POINT('Ctrl Pts',(4.27583301771352,-10.272069116189,6.));
#5387=CARTESIAN_POINT('Ctrl Pts',(4.33375724408483,-10.3010963438997,6.));
#5388=CARTESIAN_POINT('Ctrl Pts',(4.39210550098944,-10.3296904287044,6.));
#5389=CARTESIAN_POINT('Ctrl Pts',(4.45087212698484,-10.3578496987941,6.));
#5390=CARTESIAN_POINT('Ctrl Pts',(4.51005183206029,-10.3855726289458,6.));
#5391=CARTESIAN_POINT('Ctrl Pts',(4.56963961142453,-10.4128577818052,6.));
#5392=CARTESIAN_POINT('Ctrl Pts',(4.62963055491845,-10.4397037052485,6.));
#5393=CARTESIAN_POINT('Ctrl Pts',(4.69001967404874,-10.466108839161,6.));
#5394=CARTESIAN_POINT('Ctrl Pts',(4.75080174709239,-10.4920714379865,6.));
#5395=CARTESIAN_POINT('Ctrl Pts',(4.81197108362034,-10.5175894490106,6.));
#5396=CARTESIAN_POINT('Ctrl Pts',(4.87352158939685,-10.5426605691059,6.));
#5397=CARTESIAN_POINT('Ctrl Pts',(4.93544714999767,-10.5672824880187,6.));
#5398=CARTESIAN_POINT('Ctrl Pts',(4.99774193408263,-10.5914530920551,6.));
#5399=CARTESIAN_POINT('Ctrl Pts',(5.06040071098368,-10.6151706715837,6.));
#5400=CARTESIAN_POINT('Ctrl Pts',(5.12341919820983,-10.638434168447,6.));
#5401=CARTESIAN_POINT('Ctrl Pts',(5.18679427410257,-10.661243291145,6.));
#5402=CARTESIAN_POINT('Ctrl Pts',(5.25052377191005,-10.6835982206291,6.));
#5403=CARTESIAN_POINT('Ctrl Pts',(5.30178983253175,-10.7011191580639,6.));
#5404=CARTESIAN_POINT('Ctrl Pts',(5.34039795525197,-10.714055870666,6.));
#5405=CARTESIAN_POINT('Ctrl Pts',(5.3662071591827,-10.7225897134991,6.));
#5406=CARTESIAN_POINT('Ctrl Pts',(5.37912937500616,-10.726833976852,6.));
#5407=CARTESIAN_POINT('Ctrl Pts',(-5.37912937500618,-10.726833976852,-3.75));
#5408=CARTESIAN_POINT('Ctrl Pts',(-5.37912937500618,-10.726833976852,12.75));
#5409=CARTESIAN_POINT('Ctrl Pts',(-5.36620715918271,-10.7225897134991,-3.75));
#5410=CARTESIAN_POINT('Ctrl Pts',(-5.36620715918271,-10.7225897134991,12.75));
#5411=CARTESIAN_POINT('Ctrl Pts',(-5.34039795525199,-10.714055870666,-3.75));
#5412=CARTESIAN_POINT('Ctrl Pts',(-5.34039795525199,-10.714055870666,12.75));
#5413=CARTESIAN_POINT('Ctrl Pts',(-5.30178983253177,-10.7011191580639,-3.75));
#5414=CARTESIAN_POINT('Ctrl Pts',(-5.30178983253177,-10.7011191580639,12.75));
#5415=CARTESIAN_POINT('Ctrl Pts',(-5.25052377191006,-10.6835982206291,-3.75));
#5416=CARTESIAN_POINT('Ctrl Pts',(-5.25052377191006,-10.6835982206291,12.75));
#5417=CARTESIAN_POINT('Ctrl Pts',(-5.18679427410258,-10.661243291145,-3.75));
#5418=CARTESIAN_POINT('Ctrl Pts',(-5.18679427410258,-10.661243291145,12.75));
#5419=CARTESIAN_POINT('Ctrl Pts',(-5.12341919820984,-10.638434168447,-3.75));
#5420=CARTESIAN_POINT('Ctrl Pts',(-5.12341919820984,-10.638434168447,12.75));
#5421=CARTESIAN_POINT('Ctrl Pts',(-5.06040071098369,-10.6151706715837,-3.75));
#5422=CARTESIAN_POINT('Ctrl Pts',(-5.06040071098369,-10.6151706715837,12.75));
#5423=CARTESIAN_POINT('Ctrl Pts',(-4.99774193408265,-10.5914530920551,-3.75));
#5424=CARTESIAN_POINT('Ctrl Pts',(-4.99774193408265,-10.5914530920551,12.75));
#5425=CARTESIAN_POINT('Ctrl Pts',(-4.93544714999768,-10.5672824880187,-3.75));
#5426=CARTESIAN_POINT('Ctrl Pts',(-4.93544714999768,-10.5672824880187,12.75));
#5427=CARTESIAN_POINT('Ctrl Pts',(-4.87352158939686,-10.5426605691059,-3.75));
#5428=CARTESIAN_POINT('Ctrl Pts',(-4.87352158939686,-10.5426605691059,12.75));
#5429=CARTESIAN_POINT('Ctrl Pts',(-4.81197108362036,-10.5175894490106,-3.75));
#5430=CARTESIAN_POINT('Ctrl Pts',(-4.81197108362036,-10.5175894490106,12.75));
#5431=CARTESIAN_POINT('Ctrl Pts',(-4.7508017470924,-10.4920714379865,-3.75));
#5432=CARTESIAN_POINT('Ctrl Pts',(-4.7508017470924,-10.4920714379865,12.75));
#5433=CARTESIAN_POINT('Ctrl Pts',(-4.69001967404875,-10.4661088391609,-3.75));
#5434=CARTESIAN_POINT('Ctrl Pts',(-4.69001967404875,-10.4661088391609,12.75));
#5435=CARTESIAN_POINT('Ctrl Pts',(-4.62963055491846,-10.4397037052484,-3.75));
#5436=CARTESIAN_POINT('Ctrl Pts',(-4.62963055491846,-10.4397037052484,12.75));
#5437=CARTESIAN_POINT('Ctrl Pts',(-4.56963961142454,-10.4128577818052,-3.75));
#5438=CARTESIAN_POINT('Ctrl Pts',(-4.56963961142454,-10.4128577818052,12.75));
#5439=CARTESIAN_POINT('Ctrl Pts',(-4.5100518320603,-10.3855726289458,-3.75));
#5440=CARTESIAN_POINT('Ctrl Pts',(-4.5100518320603,-10.3855726289458,12.75));
#5441=CARTESIAN_POINT('Ctrl Pts',(-4.45087212698486,-10.3578496987941,-3.75));
#5442=CARTESIAN_POINT('Ctrl Pts',(-4.45087212698486,-10.3578496987941,12.75));
#5443=CARTESIAN_POINT('Ctrl Pts',(-4.39210550098945,-10.3296904287044,-3.75));
#5444=CARTESIAN_POINT('Ctrl Pts',(-4.39210550098945,-10.3296904287044,12.75));
#5445=CARTESIAN_POINT('Ctrl Pts',(-4.33375724408484,-10.3010963438997,-3.75));
#5446=CARTESIAN_POINT('Ctrl Pts',(-4.33375724408484,-10.3010963438997,12.75));
#5447=CARTESIAN_POINT('Ctrl Pts',(-4.27583301771354,-10.272069116189,-3.75));
#5448=CARTESIAN_POINT('Ctrl Pts',(-4.27583301771354,-10.272069116189,12.75));
#5449=CARTESIAN_POINT('Ctrl Pts',(-4.21833871177567,-10.2426105188232,-3.75));
#5450=CARTESIAN_POINT('Ctrl Pts',(-4.21833871177567,-10.2426105188232,12.75));
#5451=CARTESIAN_POINT('Ctrl Pts',(-4.16128034451963,-10.2127224064663,-3.75));
#5452=CARTESIAN_POINT('Ctrl Pts',(-4.16128034451963,-10.2127224064663,12.75));
#5453=CARTESIAN_POINT('Ctrl Pts',(-4.10466394929486,-10.1824066879509,-3.75));
#5454=CARTESIAN_POINT('Ctrl Pts',(-4.10466394929486,-10.1824066879509,12.75));
#5455=CARTESIAN_POINT('Ctrl Pts',(-4.04849544744087,-10.1516653064199,-3.75));
#5456=CARTESIAN_POINT('Ctrl Pts',(-4.04849544744087,-10.1516653064199,12.75));
#5457=CARTESIAN_POINT('Ctrl Pts',(-3.99278057289047,-10.1205002164952,-3.75));
#5458=CARTESIAN_POINT('Ctrl Pts',(-3.99278057289047,-10.1205002164952,12.75));
#5459=CARTESIAN_POINT('Ctrl Pts',(-3.93752506012707,-10.0889133486827,-3.75));
#5460=CARTESIAN_POINT('Ctrl Pts',(-3.93752506012707,-10.0889133486827,12.75));
#5461=CARTESIAN_POINT('Ctrl Pts',(-3.88273479532263,-10.056906577166,-3.75));
#5462=CARTESIAN_POINT('Ctrl Pts',(-3.88273479532263,-10.056906577166,12.75));
#5463=CARTESIAN_POINT('Ctrl Pts',(-3.82841597408715,-10.0244816905709,-3.75));
#5464=CARTESIAN_POINT('Ctrl Pts',(-3.82841597408715,-10.0244816905709,12.75));
#5465=CARTESIAN_POINT('Ctrl Pts',(-3.77457526401005,-9.99164036147395,-3.75));
#5466=CARTESIAN_POINT('Ctrl Pts',(-3.77457526401005,-9.99164036147395,12.75));
#5467=CARTESIAN_POINT('Ctrl Pts',(-3.72121993173637,-9.95838412799172,-3.75));
#5468=CARTESIAN_POINT('Ctrl Pts',(-3.72121993173637,-9.95838412799172,12.75));
#5469=CARTESIAN_POINT('Ctrl Pts',(-3.66835753420626,-9.92471449880882,-3.75));
#5470=CARTESIAN_POINT('Ctrl Pts',(-3.66835753420626,-9.92471449880882,12.75));
#5471=CARTESIAN_POINT('Ctrl Pts',(-3.61599563628969,-9.89063305253546,-3.75));
#5472=CARTESIAN_POINT('Ctrl Pts',(-3.61599563628969,-9.89063305253546,12.75));
#5473=CARTESIAN_POINT('Ctrl Pts',(-3.56414151726151,-9.8561415413778,-3.75));
#5474=CARTESIAN_POINT('Ctrl Pts',(-3.56414151726151,-9.8561415413778,12.75));
#5475=CARTESIAN_POINT('Ctrl Pts',(-3.51280187273296,-9.8212419982557,-3.75));
#5476=CARTESIAN_POINT('Ctrl Pts',(-3.51280187273296,-9.8212419982557,12.75));
#5477=CARTESIAN_POINT('Ctrl Pts',(-3.46198252886957,-9.78593684022037,-3.75));
#5478=CARTESIAN_POINT('Ctrl Pts',(-3.46198252886957,-9.78593684022037,12.75));
#5479=CARTESIAN_POINT('Ctrl Pts',(-3.41168916880891,-9.75022858813702,-3.75));
#5480=CARTESIAN_POINT('Ctrl Pts',(-3.41168916880891,-9.75022858813702,12.75));
#5481=CARTESIAN_POINT('Ctrl Pts',(-3.36192803839197,-9.7141195953304,-3.75));
#5482=CARTESIAN_POINT('Ctrl Pts',(-3.36192803839197,-9.7141195953304,12.75));
#5483=CARTESIAN_POINT('Ctrl Pts',(-3.31270665744062,-9.67761177523123,-3.75));
#5484=CARTESIAN_POINT('Ctrl Pts',(-3.31270665744062,-9.67761177523123,12.75));
#5485=CARTESIAN_POINT('Ctrl Pts',(-3.26403452382223,-9.64070633286081,-3.75));
#5486=CARTESIAN_POINT('Ctrl Pts',(-3.26403452382223,-9.64070633286081,12.75));
#5487=CARTESIAN_POINT('Ctrl Pts',(-3.2159238260067,-9.60340349406962,-3.75));
#5488=CARTESIAN_POINT('Ctrl Pts',(-3.2159238260067,-9.60340349406962,12.75));
#5489=CARTESIAN_POINT('Ctrl Pts',(-3.16838785383004,-9.56570313257491,-3.75));
#5490=CARTESIAN_POINT('Ctrl Pts',(-3.16838785383004,-9.56570313257491,12.75));
#5491=CARTESIAN_POINT('Ctrl Pts',(-3.121439393007,-9.52760540436562,-3.75));
#5492=CARTESIAN_POINT('Ctrl Pts',(-3.121439393007,-9.52760540436562,12.75));
#5493=CARTESIAN_POINT('Ctrl Pts',(-3.07508913212204,-9.4891113781729,-3.75));
#5494=CARTESIAN_POINT('Ctrl Pts',(-3.07508913212204,-9.4891113781729,12.75));
#5495=CARTESIAN_POINT('Ctrl Pts',(-3.02934403325601,-9.4502236812248,-3.75));
#5496=CARTESIAN_POINT('Ctrl Pts',(-3.02934403325601,-9.4502236812248,12.75));
#5497=CARTESIAN_POINT('Ctrl Pts',(-2.98420577513996,-9.4109471173216,-3.75));
#5498=CARTESIAN_POINT('Ctrl Pts',(-2.98420577513996,-9.4109471173216,12.75));
#5499=CARTESIAN_POINT('Ctrl Pts',(-2.9396747031485,-9.3712871143499,-3.75));
#5500=CARTESIAN_POINT('Ctrl Pts',(-2.9396747031485,-9.3712871143499,12.75));
#5501=CARTESIAN_POINT('Ctrl Pts',(-2.89575377593938,-9.33124817395868,-3.75));
#5502=CARTESIAN_POINT('Ctrl Pts',(-2.89575377593938,-9.33124817395868,12.75));
#5503=CARTESIAN_POINT('Ctrl Pts',(-2.8524523828002,-9.29083237315974,-3.75));
#5504=CARTESIAN_POINT('Ctrl Pts',(-2.8524523828002,-9.29083237315974,12.75));
#5505=CARTESIAN_POINT('Ctrl Pts',(-2.8097905150733,-9.2500377269296,-3.75));
#5506=CARTESIAN_POINT('Ctrl Pts',(-2.8097905150733,-9.2500377269296,12.75));
#5507=CARTESIAN_POINT('Ctrl Pts',(-2.76780196452137,-9.20885693589776,-3.75));
#5508=CARTESIAN_POINT('Ctrl Pts',(-2.76780196452137,-9.20885693589776,12.75));
#5509=CARTESIAN_POINT('Ctrl Pts',(-2.72652481622917,-9.16728115317076,-3.75));
#5510=CARTESIAN_POINT('Ctrl Pts',(-2.72652481622917,-9.16728115317076,12.75));
#5511=CARTESIAN_POINT('Ctrl Pts',(-2.68599232523134,-9.12530360007999,-3.75));
#5512=CARTESIAN_POINT('Ctrl Pts',(-2.68599232523134,-9.12530360007999,12.75));
#5513=CARTESIAN_POINT('Ctrl Pts',(-2.64622438896053,-9.08292294803309,-3.75));
#5514=CARTESIAN_POINT('Ctrl Pts',(-2.64622438896053,-9.08292294803309,12.75));
#5515=CARTESIAN_POINT('Ctrl Pts',(-2.6072169995188,-9.0401474973841,-3.75));
#5516=CARTESIAN_POINT('Ctrl Pts',(-2.6072169995188,-9.0401474973841,12.75));
#5517=CARTESIAN_POINT('Ctrl Pts',(-2.5689376774732,-8.99699699918147,-3.75));
#5518=CARTESIAN_POINT('Ctrl Pts',(-2.5689376774732,-8.99699699918147,12.75));
#5519=CARTESIAN_POINT('Ctrl Pts',(-2.53134978004338,-8.95349309713545,-3.75));
#5520=CARTESIAN_POINT('Ctrl Pts',(-2.53134978004338,-8.95349309713545,12.75));
#5521=CARTESIAN_POINT('Ctrl Pts',(-2.49443464151821,-8.90965062344541,-3.75));
#5522=CARTESIAN_POINT('Ctrl Pts',(-2.49443464151821,-8.90965062344541,12.75));
#5523=CARTESIAN_POINT('Ctrl Pts',(-2.45821141167119,-8.86546980570045,-3.75));
#5524=CARTESIAN_POINT('Ctrl Pts',(-2.45821141167119,-8.86546980570045,12.75));
#5525=CARTESIAN_POINT('Ctrl Pts',(-2.42276538248091,-8.82092512134555,-3.75));
#5526=CARTESIAN_POINT('Ctrl Pts',(-2.42276538248091,-8.82092512134555,12.75));
#5527=CARTESIAN_POINT('Ctrl Pts',(-2.38824857383289,-8.77596511266658,-3.75));
#5528=CARTESIAN_POINT('Ctrl Pts',(-2.38824857383289,-8.77596511266658,12.75));
#5529=CARTESIAN_POINT('Ctrl Pts',(-2.35482147675118,-8.73053548487858,-3.75));
#5530=CARTESIAN_POINT('Ctrl Pts',(-2.35482147675118,-8.73053548487858,12.75));
#5531=CARTESIAN_POINT('Ctrl Pts',(-2.32260171926006,-8.68459942442028,-3.75));
#5532=CARTESIAN_POINT('Ctrl Pts',(-2.32260171926006,-8.68459942442028,12.75));
#5533=CARTESIAN_POINT('Ctrl Pts',(-2.29162050823336,-8.63815494571075,-3.75));
#5534=CARTESIAN_POINT('Ctrl Pts',(-2.29162050823336,-8.63815494571075,12.75));
#5535=CARTESIAN_POINT('Ctrl Pts',(-2.26174990860572,-8.59126351952004,-3.75));
#5536=CARTESIAN_POINT('Ctrl Pts',(-2.26174990860572,-8.59126351952004,12.75));
#5537=CARTESIAN_POINT('Ctrl Pts',(-2.23274297834756,-8.54403497990068,-3.75));
#5538=CARTESIAN_POINT('Ctrl Pts',(-2.23274297834756,-8.54403497990068,12.75));
#5539=CARTESIAN_POINT('Ctrl Pts',(-2.20438215159744,-8.49657041043195,-3.75));
#5540=CARTESIAN_POINT('Ctrl Pts',(-2.20438215159744,-8.49657041043195,12.75));
#5541=CARTESIAN_POINT('Ctrl Pts',(-2.17660700812682,-8.44891314968814,-3.75));
#5542=CARTESIAN_POINT('Ctrl Pts',(-2.17660700812682,-8.44891314968814,12.75));
#5543=CARTESIAN_POINT('Ctrl Pts',(-2.1496314108288,-8.40100363162428,-3.75));
#5544=CARTESIAN_POINT('Ctrl Pts',(-2.1496314108288,-8.40100363162428,12.75));
#5545=CARTESIAN_POINT('Ctrl Pts',(-2.12411443763999,-8.35261410600662,-3.75));
#5546=CARTESIAN_POINT('Ctrl Pts',(-2.12411443763999,-8.35261410600662,12.75));
#5547=CARTESIAN_POINT('Ctrl Pts',(-2.10101049300139,-8.3034037182712,-3.75));
#5548=CARTESIAN_POINT('Ctrl Pts',(-2.10101049300139,-8.3034037182712,12.75));
#5549=CARTESIAN_POINT('Ctrl Pts',(-2.08524426770063,-8.26309465918435,-3.75));
#5550=CARTESIAN_POINT('Ctrl Pts',(-2.08524426770063,-8.26309465918435,12.75));
#5551=CARTESIAN_POINT('Ctrl Pts',(-2.07530073900945,-8.23220544002367,-3.75));
#5552=CARTESIAN_POINT('Ctrl Pts',(-2.07530073900945,-8.23220544002367,12.75));
#5553=CARTESIAN_POINT('Ctrl Pts',(-2.06955313972064,-8.21130388109186,-3.75));
#5554=CARTESIAN_POINT('Ctrl Pts',(-2.06955313972064,-8.21130388109186,12.75));
#5555=CARTESIAN_POINT('Ctrl Pts',(-2.06689970121501,-8.20077591276801,-3.75));
#5556=CARTESIAN_POINT('Ctrl Pts',(-2.06689970121501,-8.20077591276801,12.75));
#5557=CARTESIAN_POINT('',(-5.3791293750062,-10.7268339768519,-1.));
#5558=CARTESIAN_POINT('Ctrl Pts',(-5.37912937500618,-10.726833976852,-1.));
#5559=CARTESIAN_POINT('Ctrl Pts',(-5.36620715918271,-10.7225897134991,-1.));
#5560=CARTESIAN_POINT('Ctrl Pts',(-5.34039795525199,-10.714055870666,-1.));
#5561=CARTESIAN_POINT('Ctrl Pts',(-5.30178983253177,-10.7011191580639,-1.));
#5562=CARTESIAN_POINT('Ctrl Pts',(-5.25052377191006,-10.6835982206291,-1.));
#5563=CARTESIAN_POINT('Ctrl Pts',(-5.18679427410258,-10.661243291145,-1.));
#5564=CARTESIAN_POINT('Ctrl Pts',(-5.12341919820984,-10.638434168447,-1.));
#5565=CARTESIAN_POINT('Ctrl Pts',(-5.06040071098369,-10.6151706715837,-1.));
#5566=CARTESIAN_POINT('Ctrl Pts',(-4.99774193408265,-10.5914530920551,-1.));
#5567=CARTESIAN_POINT('Ctrl Pts',(-4.93544714999768,-10.5672824880187,-1.));
#5568=CARTESIAN_POINT('Ctrl Pts',(-4.87352158939686,-10.5426605691059,-1.));
#5569=CARTESIAN_POINT('Ctrl Pts',(-4.81197108362036,-10.5175894490106,-1.));
#5570=CARTESIAN_POINT('Ctrl Pts',(-4.7508017470924,-10.4920714379865,-1.));
#5571=CARTESIAN_POINT('Ctrl Pts',(-4.69001967404875,-10.4661088391609,-1.));
#5572=CARTESIAN_POINT('Ctrl Pts',(-4.62963055491846,-10.4397037052484,-1.));
#5573=CARTESIAN_POINT('Ctrl Pts',(-4.56963961142454,-10.4128577818052,-1.));
#5574=CARTESIAN_POINT('Ctrl Pts',(-4.5100518320603,-10.3855726289458,-1.));
#5575=CARTESIAN_POINT('Ctrl Pts',(-4.45087212698486,-10.3578496987941,-1.));
#5576=CARTESIAN_POINT('Ctrl Pts',(-4.39210550098945,-10.3296904287044,-1.));
#5577=CARTESIAN_POINT('Ctrl Pts',(-4.33375724408484,-10.3010963438997,-1.));
#5578=CARTESIAN_POINT('Ctrl Pts',(-4.27583301771354,-10.272069116189,-1.));
#5579=CARTESIAN_POINT('Ctrl Pts',(-4.21833871177567,-10.2426105188232,-1.));
#5580=CARTESIAN_POINT('Ctrl Pts',(-4.16128034451963,-10.2127224064663,-1.));
#5581=CARTESIAN_POINT('Ctrl Pts',(-4.10466394929486,-10.1824066879509,-1.));
#5582=CARTESIAN_POINT('Ctrl Pts',(-4.04849544744087,-10.1516653064199,-1.));
#5583=CARTESIAN_POINT('Ctrl Pts',(-3.99278057289047,-10.1205002164952,-1.));
#5584=CARTESIAN_POINT('Ctrl Pts',(-3.93752506012707,-10.0889133486827,-1.));
#5585=CARTESIAN_POINT('Ctrl Pts',(-3.88273479532263,-10.056906577166,-1.));
#5586=CARTESIAN_POINT('Ctrl Pts',(-3.82841597408715,-10.0244816905709,-1.));
#5587=CARTESIAN_POINT('Ctrl Pts',(-3.77457526401005,-9.99164036147395,-1.));
#5588=CARTESIAN_POINT('Ctrl Pts',(-3.72121993173637,-9.95838412799172,-1.));
#5589=CARTESIAN_POINT('Ctrl Pts',(-3.66835753420626,-9.92471449880882,-1.));
#5590=CARTESIAN_POINT('Ctrl Pts',(-3.61599563628969,-9.89063305253546,-1.));
#5591=CARTESIAN_POINT('Ctrl Pts',(-3.56414151726151,-9.8561415413778,-1.));
#5592=CARTESIAN_POINT('Ctrl Pts',(-3.51280187273296,-9.8212419982557,-1.));
#5593=CARTESIAN_POINT('Ctrl Pts',(-3.46198252886957,-9.78593684022037,-1.));
#5594=CARTESIAN_POINT('Ctrl Pts',(-3.41168916880891,-9.75022858813702,-1.));
#5595=CARTESIAN_POINT('Ctrl Pts',(-3.36192803839197,-9.7141195953304,-1.));
#5596=CARTESIAN_POINT('Ctrl Pts',(-3.31270665744062,-9.67761177523123,-1.));
#5597=CARTESIAN_POINT('Ctrl Pts',(-3.26403452382223,-9.64070633286081,-1.));
#5598=CARTESIAN_POINT('Ctrl Pts',(-3.2159238260067,-9.60340349406962,-1.));
#5599=CARTESIAN_POINT('Ctrl Pts',(-3.16838785383004,-9.56570313257491,-1.));
#5600=CARTESIAN_POINT('Ctrl Pts',(-3.121439393007,-9.52760540436562,-1.));
#5601=CARTESIAN_POINT('Ctrl Pts',(-3.07508913212204,-9.4891113781729,-1.));
#5602=CARTESIAN_POINT('Ctrl Pts',(-3.02934403325601,-9.4502236812248,-1.));
#5603=CARTESIAN_POINT('Ctrl Pts',(-2.98420577513996,-9.4109471173216,-1.));
#5604=CARTESIAN_POINT('Ctrl Pts',(-2.9396747031485,-9.3712871143499,-1.));
#5605=CARTESIAN_POINT('Ctrl Pts',(-2.89575377593938,-9.33124817395868,-1.));
#5606=CARTESIAN_POINT('Ctrl Pts',(-2.8524523828002,-9.29083237315974,-1.));
#5607=CARTESIAN_POINT('Ctrl Pts',(-2.8097905150733,-9.2500377269296,-1.));
#5608=CARTESIAN_POINT('Ctrl Pts',(-2.76780196452137,-9.20885693589776,-1.));
#5609=CARTESIAN_POINT('Ctrl Pts',(-2.72652481622917,-9.16728115317076,-1.));
#5610=CARTESIAN_POINT('Ctrl Pts',(-2.68599232523134,-9.12530360007999,-1.));
#5611=CARTESIAN_POINT('Ctrl Pts',(-2.64622438896053,-9.08292294803309,-1.));
#5612=CARTESIAN_POINT('Ctrl Pts',(-2.6072169995188,-9.0401474973841,-1.));
#5613=CARTESIAN_POINT('Ctrl Pts',(-2.5689376774732,-8.99699699918147,-1.));
#5614=CARTESIAN_POINT('Ctrl Pts',(-2.53134978004338,-8.95349309713545,-1.));
#5615=CARTESIAN_POINT('Ctrl Pts',(-2.49443464151821,-8.90965062344541,-1.));
#5616=CARTESIAN_POINT('Ctrl Pts',(-2.45821141167119,-8.86546980570045,-1.));
#5617=CARTESIAN_POINT('Ctrl Pts',(-2.42276538248091,-8.82092512134555,-1.));
#5618=CARTESIAN_POINT('Ctrl Pts',(-2.38824857383289,-8.77596511266658,-1.));
#5619=CARTESIAN_POINT('Ctrl Pts',(-2.35482147675118,-8.73053548487858,-1.));
#5620=CARTESIAN_POINT('Ctrl Pts',(-2.32260171926006,-8.68459942442028,-1.));
#5621=CARTESIAN_POINT('Ctrl Pts',(-2.29162050823336,-8.63815494571075,-1.));
#5622=CARTESIAN_POINT('Ctrl Pts',(-2.26174990860572,-8.59126351952004,-1.));
#5623=CARTESIAN_POINT('Ctrl Pts',(-2.23274297834756,-8.54403497990068,-1.));
#5624=CARTESIAN_POINT('Ctrl Pts',(-2.20438215159744,-8.49657041043195,-1.));
#5625=CARTESIAN_POINT('Ctrl Pts',(-2.17660700812682,-8.44891314968814,-1.));
#5626=CARTESIAN_POINT('Ctrl Pts',(-2.1496314108288,-8.40100363162428,-1.));
#5627=CARTESIAN_POINT('Ctrl Pts',(-2.12411443763999,-8.35261410600662,-1.));
#5628=CARTESIAN_POINT('Ctrl Pts',(-2.10101049300139,-8.3034037182712,-1.));
#5629=CARTESIAN_POINT('Ctrl Pts',(-2.08524426770063,-8.26309465918435,-1.));
#5630=CARTESIAN_POINT('Ctrl Pts',(-2.07530073900945,-8.23220544002367,-1.));
#5631=CARTESIAN_POINT('Ctrl Pts',(-2.06955313972064,-8.21130388109186,-1.));
#5632=CARTESIAN_POINT('Ctrl Pts',(-2.06689970121501,-8.20077591276801,-1.));
#5633=CARTESIAN_POINT('',(-5.3791293750062,-10.7268339768519,6.));
#5634=CARTESIAN_POINT('Ctrl Pts',(-5.37912937500618,-10.726833976852,6.));
#5635=CARTESIAN_POINT('Ctrl Pts',(-5.36620715918271,-10.7225897134991,6.));
#5636=CARTESIAN_POINT('Ctrl Pts',(-5.34039795525199,-10.714055870666,6.));
#5637=CARTESIAN_POINT('Ctrl Pts',(-5.30178983253177,-10.7011191580639,6.));
#5638=CARTESIAN_POINT('Ctrl Pts',(-5.25052377191006,-10.6835982206291,6.));
#5639=CARTESIAN_POINT('Ctrl Pts',(-5.18679427410258,-10.661243291145,6.));
#5640=CARTESIAN_POINT('Ctrl Pts',(-5.12341919820984,-10.638434168447,6.));
#5641=CARTESIAN_POINT('Ctrl Pts',(-5.06040071098369,-10.6151706715837,6.));
#5642=CARTESIAN_POINT('Ctrl Pts',(-4.99774193408265,-10.5914530920551,6.));
#5643=CARTESIAN_POINT('Ctrl Pts',(-4.93544714999768,-10.5672824880187,6.));
#5644=CARTESIAN_POINT('Ctrl Pts',(-4.87352158939686,-10.5426605691059,6.));
#5645=CARTESIAN_POINT('Ctrl Pts',(-4.81197108362036,-10.5175894490106,6.));
#5646=CARTESIAN_POINT('Ctrl Pts',(-4.7508017470924,-10.4920714379865,6.));
#5647=CARTESIAN_POINT('Ctrl Pts',(-4.69001967404875,-10.4661088391609,6.));
#5648=CARTESIAN_POINT('Ctrl Pts',(-4.62963055491846,-10.4397037052484,6.));
#5649=CARTESIAN_POINT('Ctrl Pts',(-4.56963961142454,-10.4128577818052,6.));
#5650=CARTESIAN_POINT('Ctrl Pts',(-4.5100518320603,-10.3855726289458,6.));
#5651=CARTESIAN_POINT('Ctrl Pts',(-4.45087212698486,-10.3578496987941,6.));
#5652=CARTESIAN_POINT('Ctrl Pts',(-4.39210550098945,-10.3296904287044,6.));
#5653=CARTESIAN_POINT('Ctrl Pts',(-4.33375724408484,-10.3010963438997,6.));
#5654=CARTESIAN_POINT('Ctrl Pts',(-4.27583301771354,-10.272069116189,6.));
#5655=CARTESIAN_POINT('Ctrl Pts',(-4.21833871177567,-10.2426105188232,6.));
#5656=CARTESIAN_POINT('Ctrl Pts',(-4.16128034451963,-10.2127224064663,6.));
#5657=CARTESIAN_POINT('Ctrl Pts',(-4.10466394929486,-10.1824066879509,6.));
#5658=CARTESIAN_POINT('Ctrl Pts',(-4.04849544744087,-10.1516653064199,6.));
#5659=CARTESIAN_POINT('Ctrl Pts',(-3.99278057289047,-10.1205002164952,6.));
#5660=CARTESIAN_POINT('Ctrl Pts',(-3.93752506012707,-10.0889133486827,6.));
#5661=CARTESIAN_POINT('Ctrl Pts',(-3.88273479532263,-10.056906577166,6.));
#5662=CARTESIAN_POINT('Ctrl Pts',(-3.82841597408715,-10.0244816905709,6.));
#5663=CARTESIAN_POINT('Ctrl Pts',(-3.77457526401005,-9.99164036147395,6.));
#5664=CARTESIAN_POINT('Ctrl Pts',(-3.72121993173637,-9.95838412799172,6.));
#5665=CARTESIAN_POINT('Ctrl Pts',(-3.66835753420626,-9.92471449880882,6.));
#5666=CARTESIAN_POINT('Ctrl Pts',(-3.61599563628969,-9.89063305253546,6.));
#5667=CARTESIAN_POINT('Ctrl Pts',(-3.56414151726151,-9.8561415413778,6.));
#5668=CARTESIAN_POINT('Ctrl Pts',(-3.51280187273296,-9.8212419982557,6.));
#5669=CARTESIAN_POINT('Ctrl Pts',(-3.46198252886957,-9.78593684022037,6.));
#5670=CARTESIAN_POINT('Ctrl Pts',(-3.41168916880891,-9.75022858813702,6.));
#5671=CARTESIAN_POINT('Ctrl Pts',(-3.36192803839197,-9.7141195953304,6.));
#5672=CARTESIAN_POINT('Ctrl Pts',(-3.31270665744062,-9.67761177523123,6.));
#5673=CARTESIAN_POINT('Ctrl Pts',(-3.26403452382223,-9.64070633286081,6.));
#5674=CARTESIAN_POINT('Ctrl Pts',(-3.2159238260067,-9.60340349406962,6.));
#5675=CARTESIAN_POINT('Ctrl Pts',(-3.16838785383004,-9.56570313257491,6.));
#5676=CARTESIAN_POINT('Ctrl Pts',(-3.121439393007,-9.52760540436562,6.));
#5677=CARTESIAN_POINT('Ctrl Pts',(-3.07508913212204,-9.4891113781729,6.));
#5678=CARTESIAN_POINT('Ctrl Pts',(-3.02934403325601,-9.4502236812248,6.));
#5679=CARTESIAN_POINT('Ctrl Pts',(-2.98420577513996,-9.4109471173216,6.));
#5680=CARTESIAN_POINT('Ctrl Pts',(-2.9396747031485,-9.3712871143499,6.));
#5681=CARTESIAN_POINT('Ctrl Pts',(-2.89575377593938,-9.33124817395868,6.));
#5682=CARTESIAN_POINT('Ctrl Pts',(-2.8524523828002,-9.29083237315974,6.));
#5683=CARTESIAN_POINT('Ctrl Pts',(-2.8097905150733,-9.2500377269296,6.));
#5684=CARTESIAN_POINT('Ctrl Pts',(-2.76780196452137,-9.20885693589776,6.));
#5685=CARTESIAN_POINT('Ctrl Pts',(-2.72652481622917,-9.16728115317076,6.));
#5686=CARTESIAN_POINT('Ctrl Pts',(-2.68599232523134,-9.12530360007999,6.));
#5687=CARTESIAN_POINT('Ctrl Pts',(-2.64622438896053,-9.08292294803309,6.));
#5688=CARTESIAN_POINT('Ctrl Pts',(-2.6072169995188,-9.0401474973841,6.));
#5689=CARTESIAN_POINT('Ctrl Pts',(-2.5689376774732,-8.99699699918147,6.));
#5690=CARTESIAN_POINT('Ctrl Pts',(-2.53134978004338,-8.95349309713545,6.));
#5691=CARTESIAN_POINT('Ctrl Pts',(-2.49443464151821,-8.90965062344541,6.));
#5692=CARTESIAN_POINT('Ctrl Pts',(-2.45821141167119,-8.86546980570045,6.));
#5693=CARTESIAN_POINT('Ctrl Pts',(-2.42276538248091,-8.82092512134555,6.));
#5694=CARTESIAN_POINT('Ctrl Pts',(-2.38824857383289,-8.77596511266658,6.));
#5695=CARTESIAN_POINT('Ctrl Pts',(-2.35482147675118,-8.73053548487858,6.));
#5696=CARTESIAN_POINT('Ctrl Pts',(-2.32260171926006,-8.68459942442028,6.));
#5697=CARTESIAN_POINT('Ctrl Pts',(-2.29162050823336,-8.63815494571075,6.));
#5698=CARTESIAN_POINT('Ctrl Pts',(-2.26174990860572,-8.59126351952004,6.));
#5699=CARTESIAN_POINT('Ctrl Pts',(-2.23274297834756,-8.54403497990068,6.));
#5700=CARTESIAN_POINT('Ctrl Pts',(-2.20438215159744,-8.49657041043195,6.));
#5701=CARTESIAN_POINT('Ctrl Pts',(-2.17660700812682,-8.44891314968814,6.));
#5702=CARTESIAN_POINT('Ctrl Pts',(-2.1496314108288,-8.40100363162428,6.));
#5703=CARTESIAN_POINT('Ctrl Pts',(-2.12411443763999,-8.35261410600662,6.));
#5704=CARTESIAN_POINT('Ctrl Pts',(-2.10101049300139,-8.3034037182712,6.));
#5705=CARTESIAN_POINT('Ctrl Pts',(-2.08524426770063,-8.26309465918435,6.));
#5706=CARTESIAN_POINT('Ctrl Pts',(-2.07530073900945,-8.23220544002367,6.));
#5707=CARTESIAN_POINT('Ctrl Pts',(-2.06955313972064,-8.21130388109186,6.));
#5708=CARTESIAN_POINT('Ctrl Pts',(-2.06689970121501,-8.20077591276801,6.));
#5709=CARTESIAN_POINT('',(-5.3791293750062,-10.7268339768519,0.));
#5710=CARTESIAN_POINT('Origin',(-1.99840144432528E-13,-3.46133283549041E-13,
0.));
#5711=CARTESIAN_POINT('',(-6.60014603862878,-10.0218796774244,-1.));
#5712=CARTESIAN_POINT('Origin',(-1.99840144432528E-13,-3.46133283549041E-13,
-1.));
#5713=CARTESIAN_POINT('',(-6.60014603862878,-10.0218796774244,6.));
#5714=CARTESIAN_POINT('Origin',(-1.99840144432528E-13,-3.46133283549041E-13,
6.));
#5715=CARTESIAN_POINT('',(-6.60014603862878,-10.0218796774244,0.));
#5716=CARTESIAN_POINT('Ctrl Pts',(-6.06863042059311,-5.89037560471066,-3.75));
#5717=CARTESIAN_POINT('Ctrl Pts',(-6.06863042059311,-5.89037560471066,12.75));
#5718=CARTESIAN_POINT('Ctrl Pts',(-6.076421189359,-5.89793753402584,-3.75));
#5719=CARTESIAN_POINT('Ctrl Pts',(-6.076421189359,-5.89793753402584,12.75));
#5720=CARTESIAN_POINT('Ctrl Pts',(-6.09164867072824,-5.91336588048663,-3.75));
#5721=CARTESIAN_POINT('Ctrl Pts',(-6.09164867072824,-5.91336588048663,12.75));
#5722=CARTESIAN_POINT('Ctrl Pts',(-6.11342775487885,-5.93742183851679,-3.75));
#5723=CARTESIAN_POINT('Ctrl Pts',(-6.11342775487885,-5.93742183851679,12.75));
#5724=CARTESIAN_POINT('Ctrl Pts',(-6.14045331140034,-5.97123031969246,-3.75));
#5725=CARTESIAN_POINT('Ctrl Pts',(-6.14045331140034,-5.97123031969246,12.75));
#5726=CARTESIAN_POINT('Ctrl Pts',(-6.17151878498999,-6.01584411654483,-3.75));
#5727=CARTESIAN_POINT('Ctrl Pts',(-6.17151878498999,-6.01584411654483,12.75));
#5728=CARTESIAN_POINT('Ctrl Pts',(-6.20066685685755,-6.06213722636286,-3.75));
#5729=CARTESIAN_POINT('Ctrl Pts',(-6.20066685685755,-6.06213722636286,12.75));
#5730=CARTESIAN_POINT('Ctrl Pts',(-6.22866991793492,-6.10945353793713,-3.75));
#5731=CARTESIAN_POINT('Ctrl Pts',(-6.22866991793492,-6.10945353793713,12.75));
#5732=CARTESIAN_POINT('Ctrl Pts',(-6.25605474467853,-6.15733614814835,-3.75));
#5733=CARTESIAN_POINT('Ctrl Pts',(-6.25605474467853,-6.15733614814835,12.75));
#5734=CARTESIAN_POINT('Ctrl Pts',(-6.28297985424308,-6.20562962932064,-3.75));
#5735=CARTESIAN_POINT('Ctrl Pts',(-6.28297985424308,-6.20562962932064,12.75));
#5736=CARTESIAN_POINT('Ctrl Pts',(-6.30937750420801,-6.2543646376197,-3.75));
#5737=CARTESIAN_POINT('Ctrl Pts',(-6.30937750420801,-6.2543646376197,12.75));
#5738=CARTESIAN_POINT('Ctrl Pts',(-6.33505137069502,-6.30367904881886,-3.75));
#5739=CARTESIAN_POINT('Ctrl Pts',(-6.33505137069502,-6.30367904881886,12.75));
#5740=CARTESIAN_POINT('Ctrl Pts',(-6.35978286360965,-6.35373180396276,-3.75));
#5741=CARTESIAN_POINT('Ctrl Pts',(-6.35978286360965,-6.35373180396276,12.75));
#5742=CARTESIAN_POINT('Ctrl Pts',(-6.38345478017076,-6.40460296268299,-3.75));
#5743=CARTESIAN_POINT('Ctrl Pts',(-6.38345478017076,-6.40460296268299,12.75));
#5744=CARTESIAN_POINT('Ctrl Pts',(-6.40608444337878,-6.45626649182452,-3.75));
#5745=CARTESIAN_POINT('Ctrl Pts',(-6.40608444337878,-6.45626649182452,12.75));
#5746=CARTESIAN_POINT('Ctrl Pts',(-6.42776254872514,-6.50863892931076,-3.75));
#5747=CARTESIAN_POINT('Ctrl Pts',(-6.42776254872514,-6.50863892931076,12.75));
#5748=CARTESIAN_POINT('Ctrl Pts',(-6.44861636238489,-6.56160843323027,-3.75));
#5749=CARTESIAN_POINT('Ctrl Pts',(-6.44861636238489,-6.56160843323027,12.75));
#5750=CARTESIAN_POINT('Ctrl Pts',(-6.46876645798849,-6.6150690793574,-3.75));
#5751=CARTESIAN_POINT('Ctrl Pts',(-6.46876645798849,-6.6150690793574,12.75));
#5752=CARTESIAN_POINT('Ctrl Pts',(-6.48827758470623,-6.66895976394943,-3.75));
#5753=CARTESIAN_POINT('Ctrl Pts',(-6.48827758470623,-6.66895976394943,12.75));
#5754=CARTESIAN_POINT('Ctrl Pts',(-6.50715912032692,-6.72326378902151,-3.75));
#5755=CARTESIAN_POINT('Ctrl Pts',(-6.50715912032692,-6.72326378902151,12.75));
#5756=CARTESIAN_POINT('Ctrl Pts',(-6.52538888693356,-6.77798990345396,-3.75));
#5757=CARTESIAN_POINT('Ctrl Pts',(-6.52538888693356,-6.77798990345396,12.75));
#5758=CARTESIAN_POINT('Ctrl Pts',(-6.54292981913304,-6.83315901897031,-3.75));
#5759=CARTESIAN_POINT('Ctrl Pts',(-6.54292981913304,-6.83315901897031,12.75));
#5760=CARTESIAN_POINT('Ctrl Pts',(-6.5597485722992,-6.88878938806037,-3.75));
#5761=CARTESIAN_POINT('Ctrl Pts',(-6.5597485722992,-6.88878938806037,12.75));
#5762=CARTESIAN_POINT('Ctrl Pts',(-6.57583595416561,-6.94488033148853,-3.75));
#5763=CARTESIAN_POINT('Ctrl Pts',(-6.57583595416561,-6.94488033148853,12.75));
#5764=CARTESIAN_POINT('Ctrl Pts',(-6.59120306404331,-7.00141528186886,-3.75));
#5765=CARTESIAN_POINT('Ctrl Pts',(-6.59120306404331,-7.00141528186886,12.75));
#5766=CARTESIAN_POINT('Ctrl Pts',(-6.60587239994886,-7.05836882883083,-3.75));
#5767=CARTESIAN_POINT('Ctrl Pts',(-6.60587239994886,-7.05836882883083,12.75));
#5768=CARTESIAN_POINT('Ctrl Pts',(-6.61987066605911,-7.11571241317029,-3.75));
#5769=CARTESIAN_POINT('Ctrl Pts',(-6.61987066605911,-7.11571241317029,12.75));
#5770=CARTESIAN_POINT('Ctrl Pts',(-6.63322107969569,-7.17342042004755,-3.75));
#5771=CARTESIAN_POINT('Ctrl Pts',(-6.63322107969569,-7.17342042004755,12.75));
#5772=CARTESIAN_POINT('Ctrl Pts',(-6.64593535561053,-7.23147652896402,-3.75));
#5773=CARTESIAN_POINT('Ctrl Pts',(-6.64593535561053,-7.23147652896402,12.75));
#5774=CARTESIAN_POINT('Ctrl Pts',(-6.65801638970246,-7.28987157005223,-3.75));
#5775=CARTESIAN_POINT('Ctrl Pts',(-6.65801638970246,-7.28987157005223,12.75));
#5776=CARTESIAN_POINT('Ctrl Pts',(-6.66946176275798,-7.34860073021491,-3.75));
#5777=CARTESIAN_POINT('Ctrl Pts',(-6.66946176275798,-7.34860073021491,12.75));
#5778=CARTESIAN_POINT('Ctrl Pts',(-6.68026694677668,-7.40766099640557,-3.75));
#5779=CARTESIAN_POINT('Ctrl Pts',(-6.68026694677668,-7.40766099640557,12.75));
#5780=CARTESIAN_POINT('Ctrl Pts',(-6.69042862091104,-7.46704851290034,-3.75));
#5781=CARTESIAN_POINT('Ctrl Pts',(-6.69042862091104,-7.46704851290034,12.75));
#5782=CARTESIAN_POINT('Ctrl Pts',(-6.69994799095524,-7.52675593674632,-3.75));
#5783=CARTESIAN_POINT('Ctrl Pts',(-6.69994799095524,-7.52675593674632,12.75));
#5784=CARTESIAN_POINT('Ctrl Pts',(-6.70882947565318,-7.58677347699225,-3.75));
#5785=CARTESIAN_POINT('Ctrl Pts',(-6.70882947565318,-7.58677347699225,12.75));
#5786=CARTESIAN_POINT('Ctrl Pts',(-6.71707933277187,-7.64708998288989,-3.75));
#5787=CARTESIAN_POINT('Ctrl Pts',(-6.71707933277187,-7.64708998288989,12.75));
#5788=CARTESIAN_POINT('Ctrl Pts',(-6.72470431659336,-7.70769400824502,-3.75));
#5789=CARTESIAN_POINT('Ctrl Pts',(-6.72470431659336,-7.70769400824502,12.75));
#5790=CARTESIAN_POINT('Ctrl Pts',(-6.73171032576036,-7.76857488460783,-3.75));
#5791=CARTESIAN_POINT('Ctrl Pts',(-6.73171032576036,-7.76857488460783,12.75));
#5792=CARTESIAN_POINT('Ctrl Pts',(-6.73810106562749,-7.82972378407324,-3.75));
#5793=CARTESIAN_POINT('Ctrl Pts',(-6.73810106562749,-7.82972378407324,12.75));
#5794=CARTESIAN_POINT('Ctrl Pts',(-6.74387863902608,-7.89113323756912,-3.75));
#5795=CARTESIAN_POINT('Ctrl Pts',(-6.74387863902608,-7.89113323756912,12.75));
#5796=CARTESIAN_POINT('Ctrl Pts',(-6.74904413083761,-7.95279665937613,-3.75));
#5797=CARTESIAN_POINT('Ctrl Pts',(-6.74904413083761,-7.95279665937613,12.75));
#5798=CARTESIAN_POINT('Ctrl Pts',(-6.75359819949755,-8.01470786732018,-3.75));
#5799=CARTESIAN_POINT('Ctrl Pts',(-6.75359819949755,-8.01470786732018,12.75));
#5800=CARTESIAN_POINT('Ctrl Pts',(-6.7575416648609,-8.07686060726827,-3.75));
#5801=CARTESIAN_POINT('Ctrl Pts',(-6.7575416648609,-8.07686060726827,12.75));
#5802=CARTESIAN_POINT('Ctrl Pts',(-6.76087611417306,-8.13924806419107,-3.75));
#5803=CARTESIAN_POINT('Ctrl Pts',(-6.76087611417306,-8.13924806419107,12.75));
#5804=CARTESIAN_POINT('Ctrl Pts',(-6.7636036696164,-8.20186305794854,-3.75));
#5805=CARTESIAN_POINT('Ctrl Pts',(-6.7636036696164,-8.20186305794854,12.75));
#5806=CARTESIAN_POINT('Ctrl Pts',(-6.76572674650935,-8.26469824786602,-3.75));
#5807=CARTESIAN_POINT('Ctrl Pts',(-6.76572674650935,-8.26469824786602,12.75));
#5808=CARTESIAN_POINT('Ctrl Pts',(-6.76724781676282,-8.32774633509908,-3.75));
#5809=CARTESIAN_POINT('Ctrl Pts',(-6.76724781676282,-8.32774633509908,12.75));
#5810=CARTESIAN_POINT('Ctrl Pts',(-6.76816918165128,-8.39100025749018,-3.75));
#5811=CARTESIAN_POINT('Ctrl Pts',(-6.76816918165128,-8.39100025749018,12.75));
#5812=CARTESIAN_POINT('Ctrl Pts',(-6.76849272647566,-8.45445340444926,-3.75));
#5813=CARTESIAN_POINT('Ctrl Pts',(-6.76849272647566,-8.45445340444926,12.75));
#5814=CARTESIAN_POINT('Ctrl Pts',(-6.76822000004555,-8.51809951610773,-3.75));
#5815=CARTESIAN_POINT('Ctrl Pts',(-6.76822000004555,-8.51809951610773,12.75));
#5816=CARTESIAN_POINT('Ctrl Pts',(-6.76735232235635,-8.58193255779939,-3.75));
#5817=CARTESIAN_POINT('Ctrl Pts',(-6.76735232235635,-8.58193255779939,12.75));
#5818=CARTESIAN_POINT('Ctrl Pts',(-6.76589088878266,-8.64594659806298,-3.75));
#5819=CARTESIAN_POINT('Ctrl Pts',(-6.76589088878266,-8.64594659806298,12.75));
#5820=CARTESIAN_POINT('Ctrl Pts',(-6.76383687353853,-8.71013569385599,-3.75));
#5821=CARTESIAN_POINT('Ctrl Pts',(-6.76383687353853,-8.71013569385599,12.75));
#5822=CARTESIAN_POINT('Ctrl Pts',(-6.76119155448275,-8.77449374557664,-3.75));
#5823=CARTESIAN_POINT('Ctrl Pts',(-6.76119155448275,-8.77449374557664,12.75));
#5824=CARTESIAN_POINT('Ctrl Pts',(-6.7579562951925,-8.8390145737747,-3.75));
#5825=CARTESIAN_POINT('Ctrl Pts',(-6.7579562951925,-8.8390145737747,12.75));
#5826=CARTESIAN_POINT('Ctrl Pts',(-6.75413249860576,-8.90369203916217,-3.75));
#5827=CARTESIAN_POINT('Ctrl Pts',(-6.75413249860576,-8.90369203916217,12.75));
#5828=CARTESIAN_POINT('Ctrl Pts',(-6.7497215739923,-8.96852015431046,-3.75));
#5829=CARTESIAN_POINT('Ctrl Pts',(-6.7497215739923,-8.96852015431046,12.75));
#5830=CARTESIAN_POINT('Ctrl Pts',(-6.74472490424423,-9.03349318036198,-3.75));
#5831=CARTESIAN_POINT('Ctrl Pts',(-6.74472490424423,-9.03349318036198,12.75));
#5832=CARTESIAN_POINT('Ctrl Pts',(-6.73914381348524,-9.09860577342165,-3.75));
#5833=CARTESIAN_POINT('Ctrl Pts',(-6.73914381348524,-9.09860577342165,12.75));
#5834=CARTESIAN_POINT('Ctrl Pts',(-6.73297955932548,-9.16385288053588,-3.75));
#5835=CARTESIAN_POINT('Ctrl Pts',(-6.73297955932548,-9.16385288053588,12.75));
#5836=CARTESIAN_POINT('Ctrl Pts',(-6.72623333926846,-9.22922952332025,-3.75));
#5837=CARTESIAN_POINT('Ctrl Pts',(-6.72623333926846,-9.22922952332025,12.75));
#5838=CARTESIAN_POINT('Ctrl Pts',(-6.71890629646187,-9.2947306015555,-3.75));
#5839=CARTESIAN_POINT('Ctrl Pts',(-6.71890629646187,-9.2947306015555,12.75));
#5840=CARTESIAN_POINT('Ctrl Pts',(-6.71099953007124,-9.36035072031876,-3.75));
#5841=CARTESIAN_POINT('Ctrl Pts',(-6.71099953007124,-9.36035072031876,12.75));
#5842=CARTESIAN_POINT('Ctrl Pts',(-6.7025141076082,-9.42608392519666,-3.75));
#5843=CARTESIAN_POINT('Ctrl Pts',(-6.7025141076082,-9.42608392519666,12.75));
#5844=CARTESIAN_POINT('Ctrl Pts',(-6.69345108162377,-9.49192378686253,-3.75));
#5845=CARTESIAN_POINT('Ctrl Pts',(-6.69345108162377,-9.49192378686253,12.75));
#5846=CARTESIAN_POINT('Ctrl Pts',(-6.68381150859183,-9.55786385494286,-3.75));
#5847=CARTESIAN_POINT('Ctrl Pts',(-6.68381150859183,-9.55786385494286,12.75));
#5848=CARTESIAN_POINT('Ctrl Pts',(-6.67359647366962,-9.62389802250187,-3.75));
#5849=CARTESIAN_POINT('Ctrl Pts',(-6.67359647366962,-9.62389802250187,12.75));
#5850=CARTESIAN_POINT('Ctrl Pts',(-6.6628071116072,-9.69002090483257,-3.75));
#5851=CARTESIAN_POINT('Ctrl Pts',(-6.6628071116072,-9.69002090483257,12.75));
#5852=CARTESIAN_POINT('Ctrl Pts',(-6.65144464725859,-9.75622826411013,-3.75));
#5853=CARTESIAN_POINT('Ctrl Pts',(-6.65144464725859,-9.75622826411013,12.75));
#5854=CARTESIAN_POINT('Ctrl Pts',(-6.63951038900667,-9.82251725114898,-3.75));
#5855=CARTESIAN_POINT('Ctrl Pts',(-6.63951038900667,-9.82251725114898,12.75));
#5856=CARTESIAN_POINT('Ctrl Pts',(-6.62700557693596,-9.88888607996273,-3.75));
#5857=CARTESIAN_POINT('Ctrl Pts',(-6.62700557693596,-9.88888607996273,12.75));
#5858=CARTESIAN_POINT('Ctrl Pts',(-6.61654612354184,-9.94204425953052,-3.75));
#5859=CARTESIAN_POINT('Ctrl Pts',(-6.61654612354184,-9.94204425953052,12.75));
#5860=CARTESIAN_POINT('Ctrl Pts',(-6.60844558393657,-9.98194823089968,-3.75));
#5861=CARTESIAN_POINT('Ctrl Pts',(-6.60844558393657,-9.98194823089968,12.75));
#5862=CARTESIAN_POINT('Ctrl Pts',(-6.60293150665659,-10.0085665785717,-3.75));
#5863=CARTESIAN_POINT('Ctrl Pts',(-6.60293150665659,-10.0085665785717,12.75));
#5864=CARTESIAN_POINT('Ctrl Pts',(-6.60014603862878,-10.0218796774244,-3.75));
#5865=CARTESIAN_POINT('Ctrl Pts',(-6.60014603862878,-10.0218796774244,12.75));
#5866=CARTESIAN_POINT('Ctrl Pts',(-6.06863042059311,-5.89037560471066,-1.));
#5867=CARTESIAN_POINT('Ctrl Pts',(-6.076421189359,-5.89793753402584,-1.));
#5868=CARTESIAN_POINT('Ctrl Pts',(-6.09164867072824,-5.91336588048663,-1.));
#5869=CARTESIAN_POINT('Ctrl Pts',(-6.11342775487885,-5.93742183851679,-1.));
#5870=CARTESIAN_POINT('Ctrl Pts',(-6.14045331140034,-5.97123031969246,-1.));
#5871=CARTESIAN_POINT('Ctrl Pts',(-6.17151878498999,-6.01584411654483,-1.));
#5872=CARTESIAN_POINT('Ctrl Pts',(-6.20066685685755,-6.06213722636286,-1.));
#5873=CARTESIAN_POINT('Ctrl Pts',(-6.22866991793492,-6.10945353793713,-1.));
#5874=CARTESIAN_POINT('Ctrl Pts',(-6.25605474467853,-6.15733614814835,-1.));
#5875=CARTESIAN_POINT('Ctrl Pts',(-6.28297985424308,-6.20562962932064,-1.));
#5876=CARTESIAN_POINT('Ctrl Pts',(-6.30937750420801,-6.2543646376197,-1.));
#5877=CARTESIAN_POINT('Ctrl Pts',(-6.33505137069502,-6.30367904881886,-1.));
#5878=CARTESIAN_POINT('Ctrl Pts',(-6.35978286360965,-6.35373180396276,-1.));
#5879=CARTESIAN_POINT('Ctrl Pts',(-6.38345478017076,-6.40460296268299,-1.));
#5880=CARTESIAN_POINT('Ctrl Pts',(-6.40608444337878,-6.45626649182452,-1.));
#5881=CARTESIAN_POINT('Ctrl Pts',(-6.42776254872514,-6.50863892931076,-1.));
#5882=CARTESIAN_POINT('Ctrl Pts',(-6.44861636238489,-6.56160843323027,-1.));
#5883=CARTESIAN_POINT('Ctrl Pts',(-6.46876645798849,-6.6150690793574,-1.));
#5884=CARTESIAN_POINT('Ctrl Pts',(-6.48827758470623,-6.66895976394943,-1.));
#5885=CARTESIAN_POINT('Ctrl Pts',(-6.50715912032692,-6.72326378902151,-1.));
#5886=CARTESIAN_POINT('Ctrl Pts',(-6.52538888693356,-6.77798990345396,-1.));
#5887=CARTESIAN_POINT('Ctrl Pts',(-6.54292981913304,-6.83315901897031,-1.));
#5888=CARTESIAN_POINT('Ctrl Pts',(-6.5597485722992,-6.88878938806037,-1.));
#5889=CARTESIAN_POINT('Ctrl Pts',(-6.57583595416561,-6.94488033148853,-1.));
#5890=CARTESIAN_POINT('Ctrl Pts',(-6.59120306404331,-7.00141528186886,-1.));
#5891=CARTESIAN_POINT('Ctrl Pts',(-6.60587239994886,-7.05836882883083,-1.));
#5892=CARTESIAN_POINT('Ctrl Pts',(-6.61987066605911,-7.11571241317029,-1.));
#5893=CARTESIAN_POINT('Ctrl Pts',(-6.63322107969569,-7.17342042004755,-1.));
#5894=CARTESIAN_POINT('Ctrl Pts',(-6.64593535561053,-7.23147652896402,-1.));
#5895=CARTESIAN_POINT('Ctrl Pts',(-6.65801638970246,-7.28987157005223,-1.));
#5896=CARTESIAN_POINT('Ctrl Pts',(-6.66946176275798,-7.34860073021491,-1.));
#5897=CARTESIAN_POINT('Ctrl Pts',(-6.68026694677668,-7.40766099640557,-1.));
#5898=CARTESIAN_POINT('Ctrl Pts',(-6.69042862091104,-7.46704851290034,-1.));
#5899=CARTESIAN_POINT('Ctrl Pts',(-6.69994799095524,-7.52675593674632,-1.));
#5900=CARTESIAN_POINT('Ctrl Pts',(-6.70882947565318,-7.58677347699225,-1.));
#5901=CARTESIAN_POINT('Ctrl Pts',(-6.71707933277187,-7.64708998288989,-1.));
#5902=CARTESIAN_POINT('Ctrl Pts',(-6.72470431659336,-7.70769400824502,-1.));
#5903=CARTESIAN_POINT('Ctrl Pts',(-6.73171032576036,-7.76857488460783,-1.));
#5904=CARTESIAN_POINT('Ctrl Pts',(-6.73810106562749,-7.82972378407324,-1.));
#5905=CARTESIAN_POINT('Ctrl Pts',(-6.74387863902608,-7.89113323756912,-1.));
#5906=CARTESIAN_POINT('Ctrl Pts',(-6.74904413083761,-7.95279665937613,-1.));
#5907=CARTESIAN_POINT('Ctrl Pts',(-6.75359819949755,-8.01470786732018,-1.));
#5908=CARTESIAN_POINT('Ctrl Pts',(-6.7575416648609,-8.07686060726827,-1.));
#5909=CARTESIAN_POINT('Ctrl Pts',(-6.76087611417306,-8.13924806419107,-1.));
#5910=CARTESIAN_POINT('Ctrl Pts',(-6.7636036696164,-8.20186305794854,-1.));
#5911=CARTESIAN_POINT('Ctrl Pts',(-6.76572674650935,-8.26469824786602,-1.));
#5912=CARTESIAN_POINT('Ctrl Pts',(-6.76724781676282,-8.32774633509908,-1.));
#5913=CARTESIAN_POINT('Ctrl Pts',(-6.76816918165128,-8.39100025749018,-1.));
#5914=CARTESIAN_POINT('Ctrl Pts',(-6.76849272647566,-8.45445340444926,-1.));
#5915=CARTESIAN_POINT('Ctrl Pts',(-6.76822000004555,-8.51809951610773,-1.));
#5916=CARTESIAN_POINT('Ctrl Pts',(-6.76735232235635,-8.58193255779939,-1.));
#5917=CARTESIAN_POINT('Ctrl Pts',(-6.76589088878266,-8.64594659806298,-1.));
#5918=CARTESIAN_POINT('Ctrl Pts',(-6.76383687353853,-8.71013569385599,-1.));
#5919=CARTESIAN_POINT('Ctrl Pts',(-6.76119155448275,-8.77449374557664,-1.));
#5920=CARTESIAN_POINT('Ctrl Pts',(-6.7579562951925,-8.8390145737747,-1.));
#5921=CARTESIAN_POINT('Ctrl Pts',(-6.75413249860576,-8.90369203916217,-1.));
#5922=CARTESIAN_POINT('Ctrl Pts',(-6.7497215739923,-8.96852015431046,-1.));
#5923=CARTESIAN_POINT('Ctrl Pts',(-6.74472490424423,-9.03349318036198,-1.));
#5924=CARTESIAN_POINT('Ctrl Pts',(-6.73914381348524,-9.09860577342165,-1.));
#5925=CARTESIAN_POINT('Ctrl Pts',(-6.73297955932548,-9.16385288053588,-1.));
#5926=CARTESIAN_POINT('Ctrl Pts',(-6.72623333926846,-9.22922952332025,-1.));
#5927=CARTESIAN_POINT('Ctrl Pts',(-6.71890629646187,-9.2947306015555,-1.));
#5928=CARTESIAN_POINT('Ctrl Pts',(-6.71099953007124,-9.36035072031876,-1.));
#5929=CARTESIAN_POINT('Ctrl Pts',(-6.7025141076082,-9.42608392519666,-1.));
#5930=CARTESIAN_POINT('Ctrl Pts',(-6.69345108162377,-9.49192378686253,-1.));
#5931=CARTESIAN_POINT('Ctrl Pts',(-6.68381150859183,-9.55786385494286,-1.));
#5932=CARTESIAN_POINT('Ctrl Pts',(-6.67359647366962,-9.62389802250187,-1.));
#5933=CARTESIAN_POINT('Ctrl Pts',(-6.6628071116072,-9.69002090483257,-1.));
#5934=CARTESIAN_POINT('Ctrl Pts',(-6.65144464725859,-9.75622826411013,-1.));
#5935=CARTESIAN_POINT('Ctrl Pts',(-6.63951038900667,-9.82251725114898,-1.));
#5936=CARTESIAN_POINT('Ctrl Pts',(-6.62700557693596,-9.88888607996273,-1.));
#5937=CARTESIAN_POINT('Ctrl Pts',(-6.61654612354184,-9.94204425953052,-1.));
#5938=CARTESIAN_POINT('Ctrl Pts',(-6.60844558393657,-9.98194823089968,-1.));
#5939=CARTESIAN_POINT('Ctrl Pts',(-6.60293150665659,-10.0085665785717,-1.));
#5940=CARTESIAN_POINT('Ctrl Pts',(-6.60014603862878,-10.0218796774244,-1.));
#5941=CARTESIAN_POINT('Ctrl Pts',(-6.06863042059311,-5.89037560471066,6.));
#5942=CARTESIAN_POINT('Ctrl Pts',(-6.076421189359,-5.89793753402584,6.));
#5943=CARTESIAN_POINT('Ctrl Pts',(-6.09164867072824,-5.91336588048663,6.));
#5944=CARTESIAN_POINT('Ctrl Pts',(-6.11342775487885,-5.93742183851679,6.));
#5945=CARTESIAN_POINT('Ctrl Pts',(-6.14045331140034,-5.97123031969246,6.));
#5946=CARTESIAN_POINT('Ctrl Pts',(-6.17151878498999,-6.01584411654483,6.));
#5947=CARTESIAN_POINT('Ctrl Pts',(-6.20066685685755,-6.06213722636286,6.));
#5948=CARTESIAN_POINT('Ctrl Pts',(-6.22866991793492,-6.10945353793713,6.));
#5949=CARTESIAN_POINT('Ctrl Pts',(-6.25605474467853,-6.15733614814835,6.));
#5950=CARTESIAN_POINT('Ctrl Pts',(-6.28297985424308,-6.20562962932064,6.));
#5951=CARTESIAN_POINT('Ctrl Pts',(-6.30937750420801,-6.2543646376197,6.));
#5952=CARTESIAN_POINT('Ctrl Pts',(-6.33505137069502,-6.30367904881886,6.));
#5953=CARTESIAN_POINT('Ctrl Pts',(-6.35978286360965,-6.35373180396276,6.));
#5954=CARTESIAN_POINT('Ctrl Pts',(-6.38345478017076,-6.40460296268299,6.));
#5955=CARTESIAN_POINT('Ctrl Pts',(-6.40608444337878,-6.45626649182452,6.));
#5956=CARTESIAN_POINT('Ctrl Pts',(-6.42776254872514,-6.50863892931076,6.));
#5957=CARTESIAN_POINT('Ctrl Pts',(-6.44861636238489,-6.56160843323027,6.));
#5958=CARTESIAN_POINT('Ctrl Pts',(-6.46876645798849,-6.6150690793574,6.));
#5959=CARTESIAN_POINT('Ctrl Pts',(-6.48827758470623,-6.66895976394943,6.));
#5960=CARTESIAN_POINT('Ctrl Pts',(-6.50715912032692,-6.72326378902151,6.));
#5961=CARTESIAN_POINT('Ctrl Pts',(-6.52538888693356,-6.77798990345396,6.));
#5962=CARTESIAN_POINT('Ctrl Pts',(-6.54292981913304,-6.83315901897031,6.));
#5963=CARTESIAN_POINT('Ctrl Pts',(-6.5597485722992,-6.88878938806037,6.));
#5964=CARTESIAN_POINT('Ctrl Pts',(-6.57583595416561,-6.94488033148853,6.));
#5965=CARTESIAN_POINT('Ctrl Pts',(-6.59120306404331,-7.00141528186886,6.));
#5966=CARTESIAN_POINT('Ctrl Pts',(-6.60587239994886,-7.05836882883083,6.));
#5967=CARTESIAN_POINT('Ctrl Pts',(-6.61987066605911,-7.11571241317029,6.));
#5968=CARTESIAN_POINT('Ctrl Pts',(-6.63322107969569,-7.17342042004755,6.));
#5969=CARTESIAN_POINT('Ctrl Pts',(-6.64593535561053,-7.23147652896402,6.));
#5970=CARTESIAN_POINT('Ctrl Pts',(-6.65801638970246,-7.28987157005223,6.));
#5971=CARTESIAN_POINT('Ctrl Pts',(-6.66946176275798,-7.34860073021491,6.));
#5972=CARTESIAN_POINT('Ctrl Pts',(-6.68026694677668,-7.40766099640557,6.));
#5973=CARTESIAN_POINT('Ctrl Pts',(-6.69042862091104,-7.46704851290034,6.));
#5974=CARTESIAN_POINT('Ctrl Pts',(-6.69994799095524,-7.52675593674632,6.));
#5975=CARTESIAN_POINT('Ctrl Pts',(-6.70882947565318,-7.58677347699225,6.));
#5976=CARTESIAN_POINT('Ctrl Pts',(-6.71707933277187,-7.64708998288989,6.));
#5977=CARTESIAN_POINT('Ctrl Pts',(-6.72470431659336,-7.70769400824502,6.));
#5978=CARTESIAN_POINT('Ctrl Pts',(-6.73171032576036,-7.76857488460783,6.));
#5979=CARTESIAN_POINT('Ctrl Pts',(-6.73810106562749,-7.82972378407324,6.));
#5980=CARTESIAN_POINT('Ctrl Pts',(-6.74387863902608,-7.89113323756912,6.));
#5981=CARTESIAN_POINT('Ctrl Pts',(-6.74904413083761,-7.95279665937613,6.));
#5982=CARTESIAN_POINT('Ctrl Pts',(-6.75359819949755,-8.01470786732018,6.));
#5983=CARTESIAN_POINT('Ctrl Pts',(-6.7575416648609,-8.07686060726827,6.));
#5984=CARTESIAN_POINT('Ctrl Pts',(-6.76087611417306,-8.13924806419107,6.));
#5985=CARTESIAN_POINT('Ctrl Pts',(-6.7636036696164,-8.20186305794854,6.));
#5986=CARTESIAN_POINT('Ctrl Pts',(-6.76572674650935,-8.26469824786602,6.));
#5987=CARTESIAN_POINT('Ctrl Pts',(-6.76724781676282,-8.32774633509908,6.));
#5988=CARTESIAN_POINT('Ctrl Pts',(-6.76816918165128,-8.39100025749018,6.));
#5989=CARTESIAN_POINT('Ctrl Pts',(-6.76849272647566,-8.45445340444926,6.));
#5990=CARTESIAN_POINT('Ctrl Pts',(-6.76822000004555,-8.51809951610773,6.));
#5991=CARTESIAN_POINT('Ctrl Pts',(-6.76735232235635,-8.58193255779939,6.));
#5992=CARTESIAN_POINT('Ctrl Pts',(-6.76589088878266,-8.64594659806298,6.));
#5993=CARTESIAN_POINT('Ctrl Pts',(-6.76383687353853,-8.71013569385599,6.));
#5994=CARTESIAN_POINT('Ctrl Pts',(-6.76119155448275,-8.77449374557664,6.));
#5995=CARTESIAN_POINT('Ctrl Pts',(-6.7579562951925,-8.8390145737747,6.));
#5996=CARTESIAN_POINT('Ctrl Pts',(-6.75413249860576,-8.90369203916217,6.));
#5997=CARTESIAN_POINT('Ctrl Pts',(-6.7497215739923,-8.96852015431046,6.));
#5998=CARTESIAN_POINT('Ctrl Pts',(-6.74472490424423,-9.03349318036198,6.));
#5999=CARTESIAN_POINT('Ctrl Pts',(-6.73914381348524,-9.09860577342165,6.));
#6000=CARTESIAN_POINT('Ctrl Pts',(-6.73297955932548,-9.16385288053588,6.));
#6001=CARTESIAN_POINT('Ctrl Pts',(-6.72623333926846,-9.22922952332025,6.));
#6002=CARTESIAN_POINT('Ctrl Pts',(-6.71890629646187,-9.2947306015555,6.));
#6003=CARTESIAN_POINT('Ctrl Pts',(-6.71099953007124,-9.36035072031876,6.));
#6004=CARTESIAN_POINT('Ctrl Pts',(-6.7025141076082,-9.42608392519666,6.));
#6005=CARTESIAN_POINT('Ctrl Pts',(-6.69345108162377,-9.49192378686253,6.));
#6006=CARTESIAN_POINT('Ctrl Pts',(-6.68381150859183,-9.55786385494286,6.));
#6007=CARTESIAN_POINT('Ctrl Pts',(-6.67359647366962,-9.62389802250187,6.));
#6008=CARTESIAN_POINT('Ctrl Pts',(-6.6628071116072,-9.69002090483257,6.));
#6009=CARTESIAN_POINT('Ctrl Pts',(-6.65144464725859,-9.75622826411013,6.));
#6010=CARTESIAN_POINT('Ctrl Pts',(-6.63951038900667,-9.82251725114898,6.));
#6011=CARTESIAN_POINT('Ctrl Pts',(-6.62700557693596,-9.88888607996273,6.));
#6012=CARTESIAN_POINT('Ctrl Pts',(-6.61654612354184,-9.94204425953052,6.));
#6013=CARTESIAN_POINT('Ctrl Pts',(-6.60844558393657,-9.98194823089968,6.));
#6014=CARTESIAN_POINT('Ctrl Pts',(-6.60293150665659,-10.0085665785717,6.));
#6015=CARTESIAN_POINT('Ctrl Pts',(-6.60014603862878,-10.0218796774244,6.));
#6016=CARTESIAN_POINT('Ctrl Pts',(-11.9792754136349,-0.704954299427526,
-3.75));
#6017=CARTESIAN_POINT('Ctrl Pts',(-11.9792754136349,-0.704954299427526,
12.75));
#6018=CARTESIAN_POINT('Ctrl Pts',(-11.9691386658393,-0.71402313492741,-3.75));
#6019=CARTESIAN_POINT('Ctrl Pts',(-11.9691386658393,-0.71402313492741,12.75));
#6020=CARTESIAN_POINT('Ctrl Pts',(-11.9488435391885,-0.732107639766307,
-3.75));
#6021=CARTESIAN_POINT('Ctrl Pts',(-11.9488435391885,-0.732107639766307,
12.75));
#6022=CARTESIAN_POINT('Ctrl Pts',(-11.9183359560736,-0.759074898533417,
-3.75));
#6023=CARTESIAN_POINT('Ctrl Pts',(-11.9183359560736,-0.759074898533417,
12.75));
#6024=CARTESIAN_POINT('Ctrl Pts',(-11.877529348846,-0.794712140666323,-3.75));
#6025=CARTESIAN_POINT('Ctrl Pts',(-11.877529348846,-0.794712140666323,12.75));
#6026=CARTESIAN_POINT('Ctrl Pts',(-11.8263046631092,-0.838726039995981,
-3.75));
#6027=CARTESIAN_POINT('Ctrl Pts',(-11.8263046631092,-0.838726039995981,
12.75));
#6028=CARTESIAN_POINT('Ctrl Pts',(-11.7748638454684,-0.882205904336895,
-3.75));
#6029=CARTESIAN_POINT('Ctrl Pts',(-11.7748638454684,-0.882205904336895,
12.75));
#6030=CARTESIAN_POINT('Ctrl Pts',(-11.7232078225909,-0.925149766751159,
-3.75));
#6031=CARTESIAN_POINT('Ctrl Pts',(-11.7232078225909,-0.925149766751159,
12.75));
#6032=CARTESIAN_POINT('Ctrl Pts',(-11.6713384077523,-0.96755506955319,-3.75));
#6033=CARTESIAN_POINT('Ctrl Pts',(-11.6713384077523,-0.96755506955319,12.75));
#6034=CARTESIAN_POINT('Ctrl Pts',(-11.6192586585895,-1.00941863307588,-3.75));
#6035=CARTESIAN_POINT('Ctrl Pts',(-11.6192586585895,-1.00941863307588,12.75));
#6036=CARTESIAN_POINT('Ctrl Pts',(-11.5669726710206,-1.05073678224334,-3.75));
#6037=CARTESIAN_POINT('Ctrl Pts',(-11.5669726710206,-1.05073678224334,12.75));
#6038=CARTESIAN_POINT('Ctrl Pts',(-11.5144851912285,-1.09150552381395,-3.75));
#6039=CARTESIAN_POINT('Ctrl Pts',(-11.5144851912285,-1.09150552381395,12.75));
#6040=CARTESIAN_POINT('Ctrl Pts',(-11.4618012771636,-1.13172071766774,-3.75));
#6041=CARTESIAN_POINT('Ctrl Pts',(-11.4618012771636,-1.13172071766774,12.75));
#6042=CARTESIAN_POINT('Ctrl Pts',(-11.4089259705106,-1.17137823760544,-3.75));
#6043=CARTESIAN_POINT('Ctrl Pts',(-11.4089259705106,-1.17137823760544,12.75));
#6044=CARTESIAN_POINT('Ctrl Pts',(-11.3558638941869,-1.21047418192819,-3.75));
#6045=CARTESIAN_POINT('Ctrl Pts',(-11.3558638941869,-1.21047418192819,12.75));
#6046=CARTESIAN_POINT('Ctrl Pts',(-11.30261917075,-1.24900490126927,-3.75));
#6047=CARTESIAN_POINT('Ctrl Pts',(-11.30261917075,-1.24900490126927,12.75));
#6048=CARTESIAN_POINT('Ctrl Pts',(-11.2491956455455,-1.28696685552412,-3.75));
#6049=CARTESIAN_POINT('Ctrl Pts',(-11.2491956455455,-1.28696685552412,12.75));
#6050=CARTESIAN_POINT('Ctrl Pts',(-11.1955970312291,-1.32435651843207,-3.75));
#6051=CARTESIAN_POINT('Ctrl Pts',(-11.1955970312291,-1.32435651843207,12.75));
#6052=CARTESIAN_POINT('Ctrl Pts',(-11.1418270749817,-1.36117027439398,-3.75));
#6053=CARTESIAN_POINT('Ctrl Pts',(-11.1418270749817,-1.36117027439398,12.75));
#6054=CARTESIAN_POINT('Ctrl Pts',(-11.0878897426906,-1.39740430473756,-3.75));
#6055=CARTESIAN_POINT('Ctrl Pts',(-11.0878897426906,-1.39740430473756,12.75));
#6056=CARTESIAN_POINT('Ctrl Pts',(-11.033789312906,-1.43305454241432,-3.75));
#6057=CARTESIAN_POINT('Ctrl Pts',(-11.033789312906,-1.43305454241432,12.75));
#6058=CARTESIAN_POINT('Ctrl Pts',(-10.9795302662584,-1.46811677324654,-3.75));
#6059=CARTESIAN_POINT('Ctrl Pts',(-10.9795302662584,-1.46811677324654,12.75));
#6060=CARTESIAN_POINT('Ctrl Pts',(-10.9251172180581,-1.50258671261028,-3.75));
#6061=CARTESIAN_POINT('Ctrl Pts',(-10.9251172180581,-1.50258671261028,12.75));
#6062=CARTESIAN_POINT('Ctrl Pts',(-10.8705548380775,-1.53646008988796,-3.75));
#6063=CARTESIAN_POINT('Ctrl Pts',(-10.8705548380775,-1.53646008988796,12.75));
#6064=CARTESIAN_POINT('Ctrl Pts',(-10.8158477697972,-1.56973274862051,-3.75));
#6065=CARTESIAN_POINT('Ctrl Pts',(-10.8158477697972,-1.56973274862051,12.75));
#6066=CARTESIAN_POINT('Ctrl Pts',(-10.761000572936,-1.60240070038749,-3.75));
#6067=CARTESIAN_POINT('Ctrl Pts',(-10.761000572936,-1.60240070038749,12.75));
#6068=CARTESIAN_POINT('Ctrl Pts',(-10.7060177866027,-1.63445994423348,-3.75));
#6069=CARTESIAN_POINT('Ctrl Pts',(-10.7060177866027,-1.63445994423348,12.75));
#6070=CARTESIAN_POINT('Ctrl Pts',(-10.6509039769739,-1.66590631967585,-3.75));
#6071=CARTESIAN_POINT('Ctrl Pts',(-10.6509039769739,-1.66590631967585,12.75));
#6072=CARTESIAN_POINT('Ctrl Pts',(-10.59566379085,-1.69673535547184,-3.75));
#6073=CARTESIAN_POINT('Ctrl Pts',(-10.59566379085,-1.69673535547184,12.75));
#6074=CARTESIAN_POINT('Ctrl Pts',(-10.5403020105194,-1.72694211360792,-3.75));
#6075=CARTESIAN_POINT('Ctrl Pts',(-10.5403020105194,-1.72694211360792,12.75));
#6076=CARTESIAN_POINT('Ctrl Pts',(-10.4848236013528,-1.75652107004318,-3.75));
#6077=CARTESIAN_POINT('Ctrl Pts',(-10.4848236013528,-1.75652107004318,12.75));
#6078=CARTESIAN_POINT('Ctrl Pts',(-10.4292336483793,-1.78546643461775,-3.75));
#6079=CARTESIAN_POINT('Ctrl Pts',(-10.4292336483793,-1.78546643461775,12.75));
#6080=CARTESIAN_POINT('Ctrl Pts',(-10.3735373011506,-1.81377244526718,-3.75));
#6081=CARTESIAN_POINT('Ctrl Pts',(-10.3735373011506,-1.81377244526718,12.75));
#6082=CARTESIAN_POINT('Ctrl Pts',(-10.317739716759,-1.84143367405762,-3.75));
#6083=CARTESIAN_POINT('Ctrl Pts',(-10.317739716759,-1.84143367405762,12.75));
#6084=CARTESIAN_POINT('Ctrl Pts',(-10.2618460035706,-1.86844533887956,-3.75));
#6085=CARTESIAN_POINT('Ctrl Pts',(-10.2618460035706,-1.86844533887956,12.75));
#6086=CARTESIAN_POINT('Ctrl Pts',(-10.2058611678956,-1.89480360265125,-3.75));
#6087=CARTESIAN_POINT('Ctrl Pts',(-10.2058611678956,-1.89480360265125,12.75));
#6088=CARTESIAN_POINT('Ctrl Pts',(-10.1497902344364,-1.92050480406378,-3.75));
#6089=CARTESIAN_POINT('Ctrl Pts',(-10.1497902344364,-1.92050480406378,12.75));
#6090=CARTESIAN_POINT('Ctrl Pts',(-10.0936383641523,-1.94554471072257,-3.75));
#6091=CARTESIAN_POINT('Ctrl Pts',(-10.0936383641523,-1.94554471072257,12.75));
#6092=CARTESIAN_POINT('Ctrl Pts',(-10.037410974034,-1.96991776698621,-3.75));
#6093=CARTESIAN_POINT('Ctrl Pts',(-10.037410974034,-1.96991776698621,12.75));
#6094=CARTESIAN_POINT('Ctrl Pts',(-9.98111385659409,-1.99361634997092,-3.75));
#6095=CARTESIAN_POINT('Ctrl Pts',(-9.98111385659409,-1.99361634997092,12.75));
#6096=CARTESIAN_POINT('Ctrl Pts',(-9.92475330165988,-2.01663001707736,-3.75));
#6097=CARTESIAN_POINT('Ctrl Pts',(-9.92475330165988,-2.01663001707736,12.75));
#6098=CARTESIAN_POINT('Ctrl Pts',(-9.86833584478527,-2.03894719582858,-3.75));
#6099=CARTESIAN_POINT('Ctrl Pts',(-9.86833584478527,-2.03894719582858,12.75));
#6100=CARTESIAN_POINT('Ctrl Pts',(-9.81186801391803,-2.06055689146527,-3.75));
#6101=CARTESIAN_POINT('Ctrl Pts',(-9.81186801391803,-2.06055689146527,12.75));
#6102=CARTESIAN_POINT('Ctrl Pts',(-9.75535607889872,-2.08145038176732,-3.75));
#6103=CARTESIAN_POINT('Ctrl Pts',(-9.75535607889872,-2.08145038176732,12.75));
#6104=CARTESIAN_POINT('Ctrl Pts',(-9.69880579601398,-2.10162295100989,-3.75));
#6105=CARTESIAN_POINT('Ctrl Pts',(-9.69880579601398,-2.10162295100989,12.75));
#6106=CARTESIAN_POINT('Ctrl Pts',(-9.64222216484242,-2.12107554726937,-3.75));
#6107=CARTESIAN_POINT('Ctrl Pts',(-9.64222216484242,-2.12107554726937,12.75));
#6108=CARTESIAN_POINT('Ctrl Pts',(-9.58561005875903,-2.13981058538587,-3.75));
#6109=CARTESIAN_POINT('Ctrl Pts',(-9.58561005875903,-2.13981058538587,12.75));
#6110=CARTESIAN_POINT('Ctrl Pts',(-9.52897485563507,-2.15782775391113,-3.75));
#6111=CARTESIAN_POINT('Ctrl Pts',(-9.52897485563507,-2.15782775391113,12.75));
#6112=CARTESIAN_POINT('Ctrl Pts',(-9.4723230488593,-2.17511995998945,-3.75));
#6113=CARTESIAN_POINT('Ctrl Pts',(-9.4723230488593,-2.17511995998945,12.75));
#6114=CARTESIAN_POINT('Ctrl Pts',(-9.41566291502215,-2.19166889809876,-3.75));
#6115=CARTESIAN_POINT('Ctrl Pts',(-9.41566291502215,-2.19166889809876,12.75));
#6116=CARTESIAN_POINT('Ctrl Pts',(-9.35900502856467,-2.2074416540289,-3.75));
#6117=CARTESIAN_POINT('Ctrl Pts',(-9.35900502856467,-2.2074416540289,12.75));
#6118=CARTESIAN_POINT('Ctrl Pts',(-9.30236077039477,-2.22240082168223,-3.75));
#6119=CARTESIAN_POINT('Ctrl Pts',(-9.30236077039477,-2.22240082168223,12.75));
#6120=CARTESIAN_POINT('Ctrl Pts',(-9.24574089753054,-2.23651421201962,-3.75));
#6121=CARTESIAN_POINT('Ctrl Pts',(-9.24574089753054,-2.23651421201962,12.75));
#6122=CARTESIAN_POINT('Ctrl Pts',(-9.18915420809356,-2.24976392906278,-3.75));
#6123=CARTESIAN_POINT('Ctrl Pts',(-9.18915420809356,-2.24976392906278,12.75));
#6124=CARTESIAN_POINT('Ctrl Pts',(-9.13260588645235,-2.26215759393014,-3.75));
#6125=CARTESIAN_POINT('Ctrl Pts',(-9.13260588645235,-2.26215759393014,12.75));
#6126=CARTESIAN_POINT('Ctrl Pts',(-9.07609679780011,-2.27373321015996,-3.75));
#6127=CARTESIAN_POINT('Ctrl Pts',(-9.07609679780011,-2.27373321015996,12.75));
#6128=CARTESIAN_POINT('Ctrl Pts',(-9.0196273647496,-2.28453333318601,-3.75));
#6129=CARTESIAN_POINT('Ctrl Pts',(-9.0196273647496,-2.28453333318601,12.75));
#6130=CARTESIAN_POINT('Ctrl Pts',(-8.96320109950669,-2.29458154408801,-3.75));
#6131=CARTESIAN_POINT('Ctrl Pts',(-8.96320109950669,-2.29458154408801,12.75));
#6132=CARTESIAN_POINT('Ctrl Pts',(-8.90682777405608,-2.30386137247017,-3.75));
#6133=CARTESIAN_POINT('Ctrl Pts',(-8.90682777405608,-2.30386137247017,12.75));
#6134=CARTESIAN_POINT('Ctrl Pts',(-8.85052793120604,-2.31228619203479,-3.75));
#6135=CARTESIAN_POINT('Ctrl Pts',(-8.85052793120604,-2.31228619203479,12.75));
#6136=CARTESIAN_POINT('Ctrl Pts',(-8.79433301721166,-2.31969862084206,-3.75));
#6137=CARTESIAN_POINT('Ctrl Pts',(-8.79433301721166,-2.31969862084206,12.75));
#6138=CARTESIAN_POINT('Ctrl Pts',(-8.73827625692193,-2.32593252219559,-3.75));
#6139=CARTESIAN_POINT('Ctrl Pts',(-8.73827625692193,-2.32593252219559,12.75));
#6140=CARTESIAN_POINT('Ctrl Pts',(-8.68238458286971,-2.33086762045752,-3.75));
#6141=CARTESIAN_POINT('Ctrl Pts',(-8.68238458286971,-2.33086762045752,12.75));
#6142=CARTESIAN_POINT('Ctrl Pts',(-8.62667187892838,-2.33447589689188,-3.75));
#6143=CARTESIAN_POINT('Ctrl Pts',(-8.62667187892838,-2.33447589689188,12.75));
#6144=CARTESIAN_POINT('Ctrl Pts',(-8.57112741281372,-2.33689888190034,-3.75));
#6145=CARTESIAN_POINT('Ctrl Pts',(-8.57112741281372,-2.33689888190034,12.75));
#6146=CARTESIAN_POINT('Ctrl Pts',(-8.51572283259063,-2.33840535058003,-3.75));
#6147=CARTESIAN_POINT('Ctrl Pts',(-8.51572283259063,-2.33840535058003,12.75));
#6148=CARTESIAN_POINT('Ctrl Pts',(-8.46043689627597,-2.3392342622836,-3.75));
#6149=CARTESIAN_POINT('Ctrl Pts',(-8.46043689627597,-2.3392342622836,12.75));
#6150=CARTESIAN_POINT('Ctrl Pts',(-8.40527692606173,-2.339459611751,-3.75));
#6151=CARTESIAN_POINT('Ctrl Pts',(-8.40527692606173,-2.339459611751,12.75));
#6152=CARTESIAN_POINT('Ctrl Pts',(-8.35029826768635,-2.33886640526141,-3.75));
#6153=CARTESIAN_POINT('Ctrl Pts',(-8.35029826768635,-2.33886640526141,12.75));
#6154=CARTESIAN_POINT('Ctrl Pts',(-8.29563322262998,-2.33676998946178,-3.75));
#6155=CARTESIAN_POINT('Ctrl Pts',(-8.29563322262998,-2.33676998946178,12.75));
#6156=CARTESIAN_POINT('Ctrl Pts',(-8.24146380440172,-2.33217339857873,-3.75));
#6157=CARTESIAN_POINT('Ctrl Pts',(-8.24146380440172,-2.33217339857873,12.75));
#6158=CARTESIAN_POINT('Ctrl Pts',(-8.19867202257948,-2.32567282066755,-3.75));
#6159=CARTESIAN_POINT('Ctrl Pts',(-8.19867202257948,-2.32567282066755,12.75));
#6160=CARTESIAN_POINT('Ctrl Pts',(-8.16694940973768,-2.31883955953704,-3.75));
#6161=CARTESIAN_POINT('Ctrl Pts',(-8.16694940973768,-2.31883955953704,12.75));
#6162=CARTESIAN_POINT('Ctrl Pts',(-8.14597432907962,-2.31336634706602,-3.75));
#6163=CARTESIAN_POINT('Ctrl Pts',(-8.14597432907962,-2.31336634706602,12.75));
#6164=CARTESIAN_POINT('Ctrl Pts',(-8.13553012180811,-2.31040030805734,-3.75));
#6165=CARTESIAN_POINT('Ctrl Pts',(-8.13553012180811,-2.31040030805734,12.75));
#6166=CARTESIAN_POINT('',(-11.9792754136349,-0.704954299427494,-1.));
#6167=CARTESIAN_POINT('Ctrl Pts',(-11.9792754136349,-0.704954299427526,
-1.));
#6168=CARTESIAN_POINT('Ctrl Pts',(-11.9691386658393,-0.71402313492741,-1.));
#6169=CARTESIAN_POINT('Ctrl Pts',(-11.9488435391885,-0.732107639766307,
-1.));
#6170=CARTESIAN_POINT('Ctrl Pts',(-11.9183359560736,-0.759074898533417,
-1.));
#6171=CARTESIAN_POINT('Ctrl Pts',(-11.877529348846,-0.794712140666323,-1.));
#6172=CARTESIAN_POINT('Ctrl Pts',(-11.8263046631092,-0.838726039995981,
-1.));
#6173=CARTESIAN_POINT('Ctrl Pts',(-11.7748638454684,-0.882205904336895,
-1.));
#6174=CARTESIAN_POINT('Ctrl Pts',(-11.7232078225909,-0.925149766751159,
-1.));
#6175=CARTESIAN_POINT('Ctrl Pts',(-11.6713384077523,-0.96755506955319,-1.));
#6176=CARTESIAN_POINT('Ctrl Pts',(-11.6192586585895,-1.00941863307588,-1.));
#6177=CARTESIAN_POINT('Ctrl Pts',(-11.5669726710206,-1.05073678224334,-1.));
#6178=CARTESIAN_POINT('Ctrl Pts',(-11.5144851912285,-1.09150552381395,-1.));
#6179=CARTESIAN_POINT('Ctrl Pts',(-11.4618012771636,-1.13172071766774,-1.));
#6180=CARTESIAN_POINT('Ctrl Pts',(-11.4089259705106,-1.17137823760544,-1.));
#6181=CARTESIAN_POINT('Ctrl Pts',(-11.3558638941869,-1.21047418192819,-1.));
#6182=CARTESIAN_POINT('Ctrl Pts',(-11.30261917075,-1.24900490126927,-1.));
#6183=CARTESIAN_POINT('Ctrl Pts',(-11.2491956455455,-1.28696685552412,-1.));
#6184=CARTESIAN_POINT('Ctrl Pts',(-11.1955970312291,-1.32435651843207,-1.));
#6185=CARTESIAN_POINT('Ctrl Pts',(-11.1418270749817,-1.36117027439398,-1.));
#6186=CARTESIAN_POINT('Ctrl Pts',(-11.0878897426906,-1.39740430473756,-1.));
#6187=CARTESIAN_POINT('Ctrl Pts',(-11.033789312906,-1.43305454241432,-1.));
#6188=CARTESIAN_POINT('Ctrl Pts',(-10.9795302662584,-1.46811677324654,-1.));
#6189=CARTESIAN_POINT('Ctrl Pts',(-10.9251172180581,-1.50258671261028,-1.));
#6190=CARTESIAN_POINT('Ctrl Pts',(-10.8705548380775,-1.53646008988796,-1.));
#6191=CARTESIAN_POINT('Ctrl Pts',(-10.8158477697972,-1.56973274862051,-1.));
#6192=CARTESIAN_POINT('Ctrl Pts',(-10.761000572936,-1.60240070038749,-1.));
#6193=CARTESIAN_POINT('Ctrl Pts',(-10.7060177866027,-1.63445994423348,-1.));
#6194=CARTESIAN_POINT('Ctrl Pts',(-10.6509039769739,-1.66590631967585,-1.));
#6195=CARTESIAN_POINT('Ctrl Pts',(-10.59566379085,-1.69673535547184,-1.));
#6196=CARTESIAN_POINT('Ctrl Pts',(-10.5403020105194,-1.72694211360792,-1.));
#6197=CARTESIAN_POINT('Ctrl Pts',(-10.4848236013528,-1.75652107004318,-1.));
#6198=CARTESIAN_POINT('Ctrl Pts',(-10.4292336483793,-1.78546643461775,-1.));
#6199=CARTESIAN_POINT('Ctrl Pts',(-10.3735373011506,-1.81377244526718,-1.));
#6200=CARTESIAN_POINT('Ctrl Pts',(-10.317739716759,-1.84143367405762,-1.));
#6201=CARTESIAN_POINT('Ctrl Pts',(-10.2618460035706,-1.86844533887956,-1.));
#6202=CARTESIAN_POINT('Ctrl Pts',(-10.2058611678956,-1.89480360265125,-1.));
#6203=CARTESIAN_POINT('Ctrl Pts',(-10.1497902344364,-1.92050480406378,-1.));
#6204=CARTESIAN_POINT('Ctrl Pts',(-10.0936383641523,-1.94554471072257,-1.));
#6205=CARTESIAN_POINT('Ctrl Pts',(-10.037410974034,-1.96991776698621,-1.));
#6206=CARTESIAN_POINT('Ctrl Pts',(-9.98111385659409,-1.99361634997092,-1.));
#6207=CARTESIAN_POINT('Ctrl Pts',(-9.92475330165988,-2.01663001707736,-1.));
#6208=CARTESIAN_POINT('Ctrl Pts',(-9.86833584478527,-2.03894719582858,-1.));
#6209=CARTESIAN_POINT('Ctrl Pts',(-9.81186801391803,-2.06055689146527,-1.));
#6210=CARTESIAN_POINT('Ctrl Pts',(-9.75535607889872,-2.08145038176732,-1.));
#6211=CARTESIAN_POINT('Ctrl Pts',(-9.69880579601398,-2.10162295100989,-1.));
#6212=CARTESIAN_POINT('Ctrl Pts',(-9.64222216484242,-2.12107554726937,-1.));
#6213=CARTESIAN_POINT('Ctrl Pts',(-9.58561005875903,-2.13981058538587,-1.));
#6214=CARTESIAN_POINT('Ctrl Pts',(-9.52897485563507,-2.15782775391113,-1.));
#6215=CARTESIAN_POINT('Ctrl Pts',(-9.4723230488593,-2.17511995998945,-1.));
#6216=CARTESIAN_POINT('Ctrl Pts',(-9.41566291502215,-2.19166889809876,-1.));
#6217=CARTESIAN_POINT('Ctrl Pts',(-9.35900502856467,-2.2074416540289,-1.));
#6218=CARTESIAN_POINT('Ctrl Pts',(-9.30236077039477,-2.22240082168223,-1.));
#6219=CARTESIAN_POINT('Ctrl Pts',(-9.24574089753054,-2.23651421201962,-1.));
#6220=CARTESIAN_POINT('Ctrl Pts',(-9.18915420809356,-2.24976392906278,-1.));
#6221=CARTESIAN_POINT('Ctrl Pts',(-9.13260588645235,-2.26215759393014,-1.));
#6222=CARTESIAN_POINT('Ctrl Pts',(-9.07609679780011,-2.27373321015996,-1.));
#6223=CARTESIAN_POINT('Ctrl Pts',(-9.0196273647496,-2.28453333318601,-1.));
#6224=CARTESIAN_POINT('Ctrl Pts',(-8.96320109950669,-2.29458154408801,-1.));
#6225=CARTESIAN_POINT('Ctrl Pts',(-8.90682777405608,-2.30386137247017,-1.));
#6226=CARTESIAN_POINT('Ctrl Pts',(-8.85052793120604,-2.31228619203479,-1.));
#6227=CARTESIAN_POINT('Ctrl Pts',(-8.79433301721166,-2.31969862084206,-1.));
#6228=CARTESIAN_POINT('Ctrl Pts',(-8.73827625692193,-2.32593252219559,-1.));
#6229=CARTESIAN_POINT('Ctrl Pts',(-8.68238458286971,-2.33086762045752,-1.));
#6230=CARTESIAN_POINT('Ctrl Pts',(-8.62667187892838,-2.33447589689188,-1.));
#6231=CARTESIAN_POINT('Ctrl Pts',(-8.57112741281372,-2.33689888190034,-1.));
#6232=CARTESIAN_POINT('Ctrl Pts',(-8.51572283259063,-2.33840535058003,-1.));
#6233=CARTESIAN_POINT('Ctrl Pts',(-8.46043689627597,-2.3392342622836,-1.));
#6234=CARTESIAN_POINT('Ctrl Pts',(-8.40527692606173,-2.339459611751,-1.));
#6235=CARTESIAN_POINT('Ctrl Pts',(-8.35029826768635,-2.33886640526141,-1.));
#6236=CARTESIAN_POINT('Ctrl Pts',(-8.29563322262998,-2.33676998946178,-1.));
#6237=CARTESIAN_POINT('Ctrl Pts',(-8.24146380440172,-2.33217339857873,-1.));
#6238=CARTESIAN_POINT('Ctrl Pts',(-8.19867202257948,-2.32567282066755,-1.));
#6239=CARTESIAN_POINT('Ctrl Pts',(-8.16694940973768,-2.31883955953704,-1.));
#6240=CARTESIAN_POINT('Ctrl Pts',(-8.14597432907962,-2.31336634706602,-1.));
#6241=CARTESIAN_POINT('Ctrl Pts',(-8.13553012180811,-2.31040030805734,-1.));
#6242=CARTESIAN_POINT('',(-11.9792754136349,-0.704954299427494,6.));
#6243=CARTESIAN_POINT('Ctrl Pts',(-11.9792754136349,-0.704954299427526,
6.));
#6244=CARTESIAN_POINT('Ctrl Pts',(-11.9691386658393,-0.71402313492741,6.));
#6245=CARTESIAN_POINT('Ctrl Pts',(-11.9488435391885,-0.732107639766307,
6.));
#6246=CARTESIAN_POINT('Ctrl Pts',(-11.9183359560736,-0.759074898533417,
6.));
#6247=CARTESIAN_POINT('Ctrl Pts',(-11.877529348846,-0.794712140666323,6.));
#6248=CARTESIAN_POINT('Ctrl Pts',(-11.8263046631092,-0.838726039995981,
6.));
#6249=CARTESIAN_POINT('Ctrl Pts',(-11.7748638454684,-0.882205904336895,
6.));
#6250=CARTESIAN_POINT('Ctrl Pts',(-11.7232078225909,-0.925149766751159,
6.));
#6251=CARTESIAN_POINT('Ctrl Pts',(-11.6713384077523,-0.96755506955319,6.));
#6252=CARTESIAN_POINT('Ctrl Pts',(-11.6192586585895,-1.00941863307588,6.));
#6253=CARTESIAN_POINT('Ctrl Pts',(-11.5669726710206,-1.05073678224334,6.));
#6254=CARTESIAN_POINT('Ctrl Pts',(-11.5144851912285,-1.09150552381395,6.));
#6255=CARTESIAN_POINT('Ctrl Pts',(-11.4618012771636,-1.13172071766774,6.));
#6256=CARTESIAN_POINT('Ctrl Pts',(-11.4089259705106,-1.17137823760544,6.));
#6257=CARTESIAN_POINT('Ctrl Pts',(-11.3558638941869,-1.21047418192819,6.));
#6258=CARTESIAN_POINT('Ctrl Pts',(-11.30261917075,-1.24900490126927,6.));
#6259=CARTESIAN_POINT('Ctrl Pts',(-11.2491956455455,-1.28696685552412,6.));
#6260=CARTESIAN_POINT('Ctrl Pts',(-11.1955970312291,-1.32435651843207,6.));
#6261=CARTESIAN_POINT('Ctrl Pts',(-11.1418270749817,-1.36117027439398,6.));
#6262=CARTESIAN_POINT('Ctrl Pts',(-11.0878897426906,-1.39740430473756,6.));
#6263=CARTESIAN_POINT('Ctrl Pts',(-11.033789312906,-1.43305454241432,6.));
#6264=CARTESIAN_POINT('Ctrl Pts',(-10.9795302662584,-1.46811677324654,6.));
#6265=CARTESIAN_POINT('Ctrl Pts',(-10.9251172180581,-1.50258671261028,6.));
#6266=CARTESIAN_POINT('Ctrl Pts',(-10.8705548380775,-1.53646008988796,6.));
#6267=CARTESIAN_POINT('Ctrl Pts',(-10.8158477697972,-1.56973274862051,6.));
#6268=CARTESIAN_POINT('Ctrl Pts',(-10.761000572936,-1.60240070038749,6.));
#6269=CARTESIAN_POINT('Ctrl Pts',(-10.7060177866027,-1.63445994423348,6.));
#6270=CARTESIAN_POINT('Ctrl Pts',(-10.6509039769739,-1.66590631967585,6.));
#6271=CARTESIAN_POINT('Ctrl Pts',(-10.59566379085,-1.69673535547184,6.));
#6272=CARTESIAN_POINT('Ctrl Pts',(-10.5403020105194,-1.72694211360792,6.));
#6273=CARTESIAN_POINT('Ctrl Pts',(-10.4848236013528,-1.75652107004318,6.));
#6274=CARTESIAN_POINT('Ctrl Pts',(-10.4292336483793,-1.78546643461775,6.));
#6275=CARTESIAN_POINT('Ctrl Pts',(-10.3735373011506,-1.81377244526718,6.));
#6276=CARTESIAN_POINT('Ctrl Pts',(-10.317739716759,-1.84143367405762,6.));
#6277=CARTESIAN_POINT('Ctrl Pts',(-10.2618460035706,-1.86844533887956,6.));
#6278=CARTESIAN_POINT('Ctrl Pts',(-10.2058611678956,-1.89480360265125,6.));
#6279=CARTESIAN_POINT('Ctrl Pts',(-10.1497902344364,-1.92050480406378,6.));
#6280=CARTESIAN_POINT('Ctrl Pts',(-10.0936383641523,-1.94554471072257,6.));
#6281=CARTESIAN_POINT('Ctrl Pts',(-10.037410974034,-1.96991776698621,6.));
#6282=CARTESIAN_POINT('Ctrl Pts',(-9.98111385659409,-1.99361634997092,6.));
#6283=CARTESIAN_POINT('Ctrl Pts',(-9.92475330165988,-2.01663001707736,6.));
#6284=CARTESIAN_POINT('Ctrl Pts',(-9.86833584478527,-2.03894719582858,6.));
#6285=CARTESIAN_POINT('Ctrl Pts',(-9.81186801391803,-2.06055689146527,6.));
#6286=CARTESIAN_POINT('Ctrl Pts',(-9.75535607889872,-2.08145038176732,6.));
#6287=CARTESIAN_POINT('Ctrl Pts',(-9.69880579601398,-2.10162295100989,6.));
#6288=CARTESIAN_POINT('Ctrl Pts',(-9.64222216484242,-2.12107554726937,6.));
#6289=CARTESIAN_POINT('Ctrl Pts',(-9.58561005875903,-2.13981058538587,6.));
#6290=CARTESIAN_POINT('Ctrl Pts',(-9.52897485563507,-2.15782775391113,6.));
#6291=CARTESIAN_POINT('Ctrl Pts',(-9.4723230488593,-2.17511995998945,6.));
#6292=CARTESIAN_POINT('Ctrl Pts',(-9.41566291502215,-2.19166889809876,6.));
#6293=CARTESIAN_POINT('Ctrl Pts',(-9.35900502856467,-2.2074416540289,6.));
#6294=CARTESIAN_POINT('Ctrl Pts',(-9.30236077039477,-2.22240082168223,6.));
#6295=CARTESIAN_POINT('Ctrl Pts',(-9.24574089753054,-2.23651421201962,6.));
#6296=CARTESIAN_POINT('Ctrl Pts',(-9.18915420809356,-2.24976392906278,6.));
#6297=CARTESIAN_POINT('Ctrl Pts',(-9.13260588645235,-2.26215759393014,6.));
#6298=CARTESIAN_POINT('Ctrl Pts',(-9.07609679780011,-2.27373321015996,6.));
#6299=CARTESIAN_POINT('Ctrl Pts',(-9.0196273647496,-2.28453333318601,6.));
#6300=CARTESIAN_POINT('Ctrl Pts',(-8.96320109950669,-2.29458154408801,6.));
#6301=CARTESIAN_POINT('Ctrl Pts',(-8.90682777405608,-2.30386137247017,6.));
#6302=CARTESIAN_POINT('Ctrl Pts',(-8.85052793120604,-2.31228619203479,6.));
#6303=CARTESIAN_POINT('Ctrl Pts',(-8.79433301721166,-2.31969862084206,6.));
#6304=CARTESIAN_POINT('Ctrl Pts',(-8.73827625692193,-2.32593252219559,6.));
#6305=CARTESIAN_POINT('Ctrl Pts',(-8.68238458286971,-2.33086762045752,6.));
#6306=CARTESIAN_POINT('Ctrl Pts',(-8.62667187892838,-2.33447589689188,6.));
#6307=CARTESIAN_POINT('Ctrl Pts',(-8.57112741281372,-2.33689888190034,6.));
#6308=CARTESIAN_POINT('Ctrl Pts',(-8.51572283259063,-2.33840535058003,6.));
#6309=CARTESIAN_POINT('Ctrl Pts',(-8.46043689627597,-2.3392342622836,6.));
#6310=CARTESIAN_POINT('Ctrl Pts',(-8.40527692606173,-2.339459611751,6.));
#6311=CARTESIAN_POINT('Ctrl Pts',(-8.35029826768635,-2.33886640526141,6.));
#6312=CARTESIAN_POINT('Ctrl Pts',(-8.29563322262998,-2.33676998946178,6.));
#6313=CARTESIAN_POINT('Ctrl Pts',(-8.24146380440172,-2.33217339857873,6.));
#6314=CARTESIAN_POINT('Ctrl Pts',(-8.19867202257948,-2.32567282066755,6.));
#6315=CARTESIAN_POINT('Ctrl Pts',(-8.16694940973768,-2.31883955953704,6.));
#6316=CARTESIAN_POINT('Ctrl Pts',(-8.14597432907962,-2.31336634706602,6.));
#6317=CARTESIAN_POINT('Ctrl Pts',(-8.13553012180811,-2.31040030805734,6.));
#6318=CARTESIAN_POINT('',(-11.9792754136349,-0.704954299427494,0.));
#6319=CARTESIAN_POINT('Origin',(-3.99680288865056E-13,3.15544362088405E-29,
0.));
#6320=CARTESIAN_POINT('',(-11.9792754136349,0.70495429942753,-1.));
#6321=CARTESIAN_POINT('Origin',(-3.99680288865056E-13,3.15544362088405E-29,
-1.));
#6322=CARTESIAN_POINT('',(-11.9792754136349,0.70495429942753,6.));
#6323=CARTESIAN_POINT('Origin',(-3.99680288865056E-13,3.15544362088405E-29,
6.));
#6324=CARTESIAN_POINT('',(-11.9792754136349,0.70495429942753,0.));
#6325=CARTESIAN_POINT('Ctrl Pts',(-8.13553012180811,2.31040030805735,-3.75));
#6326=CARTESIAN_POINT('Ctrl Pts',(-8.13553012180811,2.31040030805735,12.75));
#6327=CARTESIAN_POINT('Ctrl Pts',(-8.14597432907962,2.31336634706602,-3.75));
#6328=CARTESIAN_POINT('Ctrl Pts',(-8.14597432907962,2.31336634706602,12.75));
#6329=CARTESIAN_POINT('Ctrl Pts',(-8.16694940973767,2.31883955953704,-3.75));
#6330=CARTESIAN_POINT('Ctrl Pts',(-8.16694940973767,2.31883955953704,12.75));
#6331=CARTESIAN_POINT('Ctrl Pts',(-8.19867202257948,2.32567282066756,-3.75));
#6332=CARTESIAN_POINT('Ctrl Pts',(-8.19867202257948,2.32567282066756,12.75));
#6333=CARTESIAN_POINT('Ctrl Pts',(-8.24146380440172,2.33217339857874,-3.75));
#6334=CARTESIAN_POINT('Ctrl Pts',(-8.24146380440172,2.33217339857874,12.75));
#6335=CARTESIAN_POINT('Ctrl Pts',(-8.29563322262998,2.33676998946179,-3.75));
#6336=CARTESIAN_POINT('Ctrl Pts',(-8.29563322262998,2.33676998946179,12.75));
#6337=CARTESIAN_POINT('Ctrl Pts',(-8.35029826768635,2.33886640526142,-3.75));
#6338=CARTESIAN_POINT('Ctrl Pts',(-8.35029826768635,2.33886640526142,12.75));
#6339=CARTESIAN_POINT('Ctrl Pts',(-8.40527692606173,2.33945961175101,-3.75));
#6340=CARTESIAN_POINT('Ctrl Pts',(-8.40527692606173,2.33945961175101,12.75));
#6341=CARTESIAN_POINT('Ctrl Pts',(-8.46043689627596,2.3392342622836,-3.75));
#6342=CARTESIAN_POINT('Ctrl Pts',(-8.46043689627596,2.3392342622836,12.75));
#6343=CARTESIAN_POINT('Ctrl Pts',(-8.51572283259063,2.33840535058003,-3.75));
#6344=CARTESIAN_POINT('Ctrl Pts',(-8.51572283259063,2.33840535058003,12.75));
#6345=CARTESIAN_POINT('Ctrl Pts',(-8.57112741281372,2.33689888190034,-3.75));
#6346=CARTESIAN_POINT('Ctrl Pts',(-8.57112741281372,2.33689888190034,12.75));
#6347=CARTESIAN_POINT('Ctrl Pts',(-8.62667187892838,2.33447589689188,-3.75));
#6348=CARTESIAN_POINT('Ctrl Pts',(-8.62667187892838,2.33447589689188,12.75));
#6349=CARTESIAN_POINT('Ctrl Pts',(-8.68238458286971,2.33086762045752,-3.75));
#6350=CARTESIAN_POINT('Ctrl Pts',(-8.68238458286971,2.33086762045752,12.75));
#6351=CARTESIAN_POINT('Ctrl Pts',(-8.73827625692193,2.32593252219559,-3.75));
#6352=CARTESIAN_POINT('Ctrl Pts',(-8.73827625692193,2.32593252219559,12.75));
#6353=CARTESIAN_POINT('Ctrl Pts',(-8.79433301721166,2.31969862084206,-3.75));
#6354=CARTESIAN_POINT('Ctrl Pts',(-8.79433301721166,2.31969862084206,12.75));
#6355=CARTESIAN_POINT('Ctrl Pts',(-8.85052793120604,2.31228619203479,-3.75));
#6356=CARTESIAN_POINT('Ctrl Pts',(-8.85052793120604,2.31228619203479,12.75));
#6357=CARTESIAN_POINT('Ctrl Pts',(-8.90682777405608,2.30386137247017,-3.75));
#6358=CARTESIAN_POINT('Ctrl Pts',(-8.90682777405608,2.30386137247017,12.75));
#6359=CARTESIAN_POINT('Ctrl Pts',(-8.96320109950669,2.29458154408801,-3.75));
#6360=CARTESIAN_POINT('Ctrl Pts',(-8.96320109950669,2.29458154408801,12.75));
#6361=CARTESIAN_POINT('Ctrl Pts',(-9.0196273647496,2.28453333318601,-3.75));
#6362=CARTESIAN_POINT('Ctrl Pts',(-9.0196273647496,2.28453333318601,12.75));
#6363=CARTESIAN_POINT('Ctrl Pts',(-9.07609679780011,2.27373321015996,-3.75));
#6364=CARTESIAN_POINT('Ctrl Pts',(-9.07609679780011,2.27373321015996,12.75));
#6365=CARTESIAN_POINT('Ctrl Pts',(-9.13260588645235,2.26215759393014,-3.75));
#6366=CARTESIAN_POINT('Ctrl Pts',(-9.13260588645235,2.26215759393014,12.75));
#6367=CARTESIAN_POINT('Ctrl Pts',(-9.18915420809356,2.24976392906278,-3.75));
#6368=CARTESIAN_POINT('Ctrl Pts',(-9.18915420809356,2.24976392906278,12.75));
#6369=CARTESIAN_POINT('Ctrl Pts',(-9.24574089753053,2.23651421201962,-3.75));
#6370=CARTESIAN_POINT('Ctrl Pts',(-9.24574089753053,2.23651421201962,12.75));
#6371=CARTESIAN_POINT('Ctrl Pts',(-9.30236077039476,2.22240082168223,-3.75));
#6372=CARTESIAN_POINT('Ctrl Pts',(-9.30236077039476,2.22240082168223,12.75));
#6373=CARTESIAN_POINT('Ctrl Pts',(-9.35900502856467,2.2074416540289,-3.75));
#6374=CARTESIAN_POINT('Ctrl Pts',(-9.35900502856467,2.2074416540289,12.75));
#6375=CARTESIAN_POINT('Ctrl Pts',(-9.41566291502215,2.19166889809877,-3.75));
#6376=CARTESIAN_POINT('Ctrl Pts',(-9.41566291502215,2.19166889809877,12.75));
#6377=CARTESIAN_POINT('Ctrl Pts',(-9.4723230488593,2.17511995998945,-3.75));
#6378=CARTESIAN_POINT('Ctrl Pts',(-9.4723230488593,2.17511995998945,12.75));
#6379=CARTESIAN_POINT('Ctrl Pts',(-9.52897485563506,2.15782775391113,-3.75));
#6380=CARTESIAN_POINT('Ctrl Pts',(-9.52897485563506,2.15782775391113,12.75));
#6381=CARTESIAN_POINT('Ctrl Pts',(-9.58561005875903,2.13981058538588,-3.75));
#6382=CARTESIAN_POINT('Ctrl Pts',(-9.58561005875903,2.13981058538588,12.75));
#6383=CARTESIAN_POINT('Ctrl Pts',(-9.64222216484242,2.12107554726937,-3.75));
#6384=CARTESIAN_POINT('Ctrl Pts',(-9.64222216484242,2.12107554726937,12.75));
#6385=CARTESIAN_POINT('Ctrl Pts',(-9.69880579601398,2.10162295100989,-3.75));
#6386=CARTESIAN_POINT('Ctrl Pts',(-9.69880579601398,2.10162295100989,12.75));
#6387=CARTESIAN_POINT('Ctrl Pts',(-9.75535607889872,2.08145038176733,-3.75));
#6388=CARTESIAN_POINT('Ctrl Pts',(-9.75535607889872,2.08145038176733,12.75));
#6389=CARTESIAN_POINT('Ctrl Pts',(-9.81186801391803,2.06055689146528,-3.75));
#6390=CARTESIAN_POINT('Ctrl Pts',(-9.81186801391803,2.06055689146528,12.75));
#6391=CARTESIAN_POINT('Ctrl Pts',(-9.86833584478527,2.03894719582859,-3.75));
#6392=CARTESIAN_POINT('Ctrl Pts',(-9.86833584478527,2.03894719582859,12.75));
#6393=CARTESIAN_POINT('Ctrl Pts',(-9.92475330165988,2.01663001707736,-3.75));
#6394=CARTESIAN_POINT('Ctrl Pts',(-9.92475330165988,2.01663001707736,12.75));
#6395=CARTESIAN_POINT('Ctrl Pts',(-9.98111385659409,1.99361634997092,-3.75));
#6396=CARTESIAN_POINT('Ctrl Pts',(-9.98111385659409,1.99361634997092,12.75));
#6397=CARTESIAN_POINT('Ctrl Pts',(-10.037410974034,1.96991776698621,-3.75));
#6398=CARTESIAN_POINT('Ctrl Pts',(-10.037410974034,1.96991776698621,12.75));
#6399=CARTESIAN_POINT('Ctrl Pts',(-10.0936383641523,1.94554471072257,-3.75));
#6400=CARTESIAN_POINT('Ctrl Pts',(-10.0936383641523,1.94554471072257,12.75));
#6401=CARTESIAN_POINT('Ctrl Pts',(-10.1497902344364,1.92050480406378,-3.75));
#6402=CARTESIAN_POINT('Ctrl Pts',(-10.1497902344364,1.92050480406378,12.75));
#6403=CARTESIAN_POINT('Ctrl Pts',(-10.2058611678956,1.89480360265125,-3.75));
#6404=CARTESIAN_POINT('Ctrl Pts',(-10.2058611678956,1.89480360265125,12.75));
#6405=CARTESIAN_POINT('Ctrl Pts',(-10.2618460035706,1.86844533887956,-3.75));
#6406=CARTESIAN_POINT('Ctrl Pts',(-10.2618460035706,1.86844533887956,12.75));
#6407=CARTESIAN_POINT('Ctrl Pts',(-10.317739716759,1.84143367405763,-3.75));
#6408=CARTESIAN_POINT('Ctrl Pts',(-10.317739716759,1.84143367405763,12.75));
#6409=CARTESIAN_POINT('Ctrl Pts',(-10.3735373011506,1.81377244526719,-3.75));
#6410=CARTESIAN_POINT('Ctrl Pts',(-10.3735373011506,1.81377244526719,12.75));
#6411=CARTESIAN_POINT('Ctrl Pts',(-10.4292336483793,1.78546643461776,-3.75));
#6412=CARTESIAN_POINT('Ctrl Pts',(-10.4292336483793,1.78546643461776,12.75));
#6413=CARTESIAN_POINT('Ctrl Pts',(-10.4848236013528,1.75652107004318,-3.75));
#6414=CARTESIAN_POINT('Ctrl Pts',(-10.4848236013528,1.75652107004318,12.75));
#6415=CARTESIAN_POINT('Ctrl Pts',(-10.5403020105194,1.72694211360793,-3.75));
#6416=CARTESIAN_POINT('Ctrl Pts',(-10.5403020105194,1.72694211360793,12.75));
#6417=CARTESIAN_POINT('Ctrl Pts',(-10.59566379085,1.69673535547185,-3.75));
#6418=CARTESIAN_POINT('Ctrl Pts',(-10.59566379085,1.69673535547185,12.75));
#6419=CARTESIAN_POINT('Ctrl Pts',(-10.6509039769739,1.66590631967585,-3.75));
#6420=CARTESIAN_POINT('Ctrl Pts',(-10.6509039769739,1.66590631967585,12.75));
#6421=CARTESIAN_POINT('Ctrl Pts',(-10.7060177866027,1.63445994423349,-3.75));
#6422=CARTESIAN_POINT('Ctrl Pts',(-10.7060177866027,1.63445994423349,12.75));
#6423=CARTESIAN_POINT('Ctrl Pts',(-10.761000572936,1.60240070038749,-3.75));
#6424=CARTESIAN_POINT('Ctrl Pts',(-10.761000572936,1.60240070038749,12.75));
#6425=CARTESIAN_POINT('Ctrl Pts',(-10.8158477697972,1.56973274862052,-3.75));
#6426=CARTESIAN_POINT('Ctrl Pts',(-10.8158477697972,1.56973274862052,12.75));
#6427=CARTESIAN_POINT('Ctrl Pts',(-10.8705548380775,1.53646008988796,-3.75));
#6428=CARTESIAN_POINT('Ctrl Pts',(-10.8705548380775,1.53646008988796,12.75));
#6429=CARTESIAN_POINT('Ctrl Pts',(-10.9251172180581,1.50258671261028,-3.75));
#6430=CARTESIAN_POINT('Ctrl Pts',(-10.9251172180581,1.50258671261028,12.75));
#6431=CARTESIAN_POINT('Ctrl Pts',(-10.9795302662584,1.46811677324654,-3.75));
#6432=CARTESIAN_POINT('Ctrl Pts',(-10.9795302662584,1.46811677324654,12.75));
#6433=CARTESIAN_POINT('Ctrl Pts',(-11.033789312906,1.43305454241432,-3.75));
#6434=CARTESIAN_POINT('Ctrl Pts',(-11.033789312906,1.43305454241432,12.75));
#6435=CARTESIAN_POINT('Ctrl Pts',(-11.0878897426906,1.39740430473757,-3.75));
#6436=CARTESIAN_POINT('Ctrl Pts',(-11.0878897426906,1.39740430473757,12.75));
#6437=CARTESIAN_POINT('Ctrl Pts',(-11.1418270749817,1.36117027439398,-3.75));
#6438=CARTESIAN_POINT('Ctrl Pts',(-11.1418270749817,1.36117027439398,12.75));
#6439=CARTESIAN_POINT('Ctrl Pts',(-11.1955970312291,1.32435651843207,-3.75));
#6440=CARTESIAN_POINT('Ctrl Pts',(-11.1955970312291,1.32435651843207,12.75));
#6441=CARTESIAN_POINT('Ctrl Pts',(-11.2491956455455,1.28696685552412,-3.75));
#6442=CARTESIAN_POINT('Ctrl Pts',(-11.2491956455455,1.28696685552412,12.75));
#6443=CARTESIAN_POINT('Ctrl Pts',(-11.30261917075,1.24900490126928,-3.75));
#6444=CARTESIAN_POINT('Ctrl Pts',(-11.30261917075,1.24900490126928,12.75));
#6445=CARTESIAN_POINT('Ctrl Pts',(-11.3558638941869,1.21047418192819,-3.75));
#6446=CARTESIAN_POINT('Ctrl Pts',(-11.3558638941869,1.21047418192819,12.75));
#6447=CARTESIAN_POINT('Ctrl Pts',(-11.4089259705106,1.17137823760545,-3.75));
#6448=CARTESIAN_POINT('Ctrl Pts',(-11.4089259705106,1.17137823760545,12.75));
#6449=CARTESIAN_POINT('Ctrl Pts',(-11.4618012771636,1.13172071766774,-3.75));
#6450=CARTESIAN_POINT('Ctrl Pts',(-11.4618012771636,1.13172071766774,12.75));
#6451=CARTESIAN_POINT('Ctrl Pts',(-11.5144851912285,1.09150552381395,-3.75));
#6452=CARTESIAN_POINT('Ctrl Pts',(-11.5144851912285,1.09150552381395,12.75));
#6453=CARTESIAN_POINT('Ctrl Pts',(-11.5669726710206,1.05073678224335,-3.75));
#6454=CARTESIAN_POINT('Ctrl Pts',(-11.5669726710206,1.05073678224335,12.75));
#6455=CARTESIAN_POINT('Ctrl Pts',(-11.6192586585895,1.00941863307588,-3.75));
#6456=CARTESIAN_POINT('Ctrl Pts',(-11.6192586585895,1.00941863307588,12.75));
#6457=CARTESIAN_POINT('Ctrl Pts',(-11.6713384077523,0.967555069553195,-3.75));
#6458=CARTESIAN_POINT('Ctrl Pts',(-11.6713384077523,0.967555069553195,12.75));
#6459=CARTESIAN_POINT('Ctrl Pts',(-11.7232078225909,0.925149766751162,-3.75));
#6460=CARTESIAN_POINT('Ctrl Pts',(-11.7232078225909,0.925149766751162,12.75));
#6461=CARTESIAN_POINT('Ctrl Pts',(-11.7748638454684,0.882205904336898,-3.75));
#6462=CARTESIAN_POINT('Ctrl Pts',(-11.7748638454684,0.882205904336898,12.75));
#6463=CARTESIAN_POINT('Ctrl Pts',(-11.8263046631092,0.838726039995983,-3.75));
#6464=CARTESIAN_POINT('Ctrl Pts',(-11.8263046631092,0.838726039995983,12.75));
#6465=CARTESIAN_POINT('Ctrl Pts',(-11.877529348846,0.794712140666327,-3.75));
#6466=CARTESIAN_POINT('Ctrl Pts',(-11.877529348846,0.794712140666327,12.75));
#6467=CARTESIAN_POINT('Ctrl Pts',(-11.9183359560736,0.759074898533419,-3.75));
#6468=CARTESIAN_POINT('Ctrl Pts',(-11.9183359560736,0.759074898533419,12.75));
#6469=CARTESIAN_POINT('Ctrl Pts',(-11.9488435391885,0.732107639766311,-3.75));
#6470=CARTESIAN_POINT('Ctrl Pts',(-11.9488435391885,0.732107639766311,12.75));
#6471=CARTESIAN_POINT('Ctrl Pts',(-11.9691386658393,0.714023134927412,-3.75));
#6472=CARTESIAN_POINT('Ctrl Pts',(-11.9691386658393,0.714023134927412,12.75));
#6473=CARTESIAN_POINT('Ctrl Pts',(-11.9792754136349,0.70495429942753,-3.75));
#6474=CARTESIAN_POINT('Ctrl Pts',(-11.9792754136349,0.70495429942753,12.75));
#6475=CARTESIAN_POINT('Ctrl Pts',(-8.13553012180811,2.31040030805735,-1.));
#6476=CARTESIAN_POINT('Ctrl Pts',(-8.14597432907962,2.31336634706602,-1.));
#6477=CARTESIAN_POINT('Ctrl Pts',(-8.16694940973767,2.31883955953704,-1.));
#6478=CARTESIAN_POINT('Ctrl Pts',(-8.19867202257948,2.32567282066756,-1.));
#6479=CARTESIAN_POINT('Ctrl Pts',(-8.24146380440172,2.33217339857874,-1.));
#6480=CARTESIAN_POINT('Ctrl Pts',(-8.29563322262998,2.33676998946179,-1.));
#6481=CARTESIAN_POINT('Ctrl Pts',(-8.35029826768635,2.33886640526142,-1.));
#6482=CARTESIAN_POINT('Ctrl Pts',(-8.40527692606173,2.33945961175101,-1.));
#6483=CARTESIAN_POINT('Ctrl Pts',(-8.46043689627596,2.3392342622836,-1.));
#6484=CARTESIAN_POINT('Ctrl Pts',(-8.51572283259063,2.33840535058003,-1.));
#6485=CARTESIAN_POINT('Ctrl Pts',(-8.57112741281372,2.33689888190034,-1.));
#6486=CARTESIAN_POINT('Ctrl Pts',(-8.62667187892838,2.33447589689188,-1.));
#6487=CARTESIAN_POINT('Ctrl Pts',(-8.68238458286971,2.33086762045752,-1.));
#6488=CARTESIAN_POINT('Ctrl Pts',(-8.73827625692193,2.32593252219559,-1.));
#6489=CARTESIAN_POINT('Ctrl Pts',(-8.79433301721166,2.31969862084206,-1.));
#6490=CARTESIAN_POINT('Ctrl Pts',(-8.85052793120604,2.31228619203479,-1.));
#6491=CARTESIAN_POINT('Ctrl Pts',(-8.90682777405608,2.30386137247017,-1.));
#6492=CARTESIAN_POINT('Ctrl Pts',(-8.96320109950669,2.29458154408801,-1.));
#6493=CARTESIAN_POINT('Ctrl Pts',(-9.0196273647496,2.28453333318601,-1.));
#6494=CARTESIAN_POINT('Ctrl Pts',(-9.07609679780011,2.27373321015996,-1.));
#6495=CARTESIAN_POINT('Ctrl Pts',(-9.13260588645235,2.26215759393014,-1.));
#6496=CARTESIAN_POINT('Ctrl Pts',(-9.18915420809356,2.24976392906278,-1.));
#6497=CARTESIAN_POINT('Ctrl Pts',(-9.24574089753053,2.23651421201962,-1.));
#6498=CARTESIAN_POINT('Ctrl Pts',(-9.30236077039476,2.22240082168223,-1.));
#6499=CARTESIAN_POINT('Ctrl Pts',(-9.35900502856467,2.2074416540289,-1.));
#6500=CARTESIAN_POINT('Ctrl Pts',(-9.41566291502215,2.19166889809877,-1.));
#6501=CARTESIAN_POINT('Ctrl Pts',(-9.4723230488593,2.17511995998945,-1.));
#6502=CARTESIAN_POINT('Ctrl Pts',(-9.52897485563506,2.15782775391113,-1.));
#6503=CARTESIAN_POINT('Ctrl Pts',(-9.58561005875903,2.13981058538588,-1.));
#6504=CARTESIAN_POINT('Ctrl Pts',(-9.64222216484242,2.12107554726937,-1.));
#6505=CARTESIAN_POINT('Ctrl Pts',(-9.69880579601398,2.10162295100989,-1.));
#6506=CARTESIAN_POINT('Ctrl Pts',(-9.75535607889872,2.08145038176733,-1.));
#6507=CARTESIAN_POINT('Ctrl Pts',(-9.81186801391803,2.06055689146528,-1.));
#6508=CARTESIAN_POINT('Ctrl Pts',(-9.86833584478527,2.03894719582859,-1.));
#6509=CARTESIAN_POINT('Ctrl Pts',(-9.92475330165988,2.01663001707736,-1.));
#6510=CARTESIAN_POINT('Ctrl Pts',(-9.98111385659409,1.99361634997092,-1.));
#6511=CARTESIAN_POINT('Ctrl Pts',(-10.037410974034,1.96991776698621,-1.));
#6512=CARTESIAN_POINT('Ctrl Pts',(-10.0936383641523,1.94554471072257,-1.));
#6513=CARTESIAN_POINT('Ctrl Pts',(-10.1497902344364,1.92050480406378,-1.));
#6514=CARTESIAN_POINT('Ctrl Pts',(-10.2058611678956,1.89480360265125,-1.));
#6515=CARTESIAN_POINT('Ctrl Pts',(-10.2618460035706,1.86844533887956,-1.));
#6516=CARTESIAN_POINT('Ctrl Pts',(-10.317739716759,1.84143367405763,-1.));
#6517=CARTESIAN_POINT('Ctrl Pts',(-10.3735373011506,1.81377244526719,-1.));
#6518=CARTESIAN_POINT('Ctrl Pts',(-10.4292336483793,1.78546643461776,-1.));
#6519=CARTESIAN_POINT('Ctrl Pts',(-10.4848236013528,1.75652107004318,-1.));
#6520=CARTESIAN_POINT('Ctrl Pts',(-10.5403020105194,1.72694211360793,-1.));
#6521=CARTESIAN_POINT('Ctrl Pts',(-10.59566379085,1.69673535547185,-1.));
#6522=CARTESIAN_POINT('Ctrl Pts',(-10.6509039769739,1.66590631967585,-1.));
#6523=CARTESIAN_POINT('Ctrl Pts',(-10.7060177866027,1.63445994423349,-1.));
#6524=CARTESIAN_POINT('Ctrl Pts',(-10.761000572936,1.60240070038749,-1.));
#6525=CARTESIAN_POINT('Ctrl Pts',(-10.8158477697972,1.56973274862052,-1.));
#6526=CARTESIAN_POINT('Ctrl Pts',(-10.8705548380775,1.53646008988796,-1.));
#6527=CARTESIAN_POINT('Ctrl Pts',(-10.9251172180581,1.50258671261028,-1.));
#6528=CARTESIAN_POINT('Ctrl Pts',(-10.9795302662584,1.46811677324654,-1.));
#6529=CARTESIAN_POINT('Ctrl Pts',(-11.033789312906,1.43305454241432,-1.));
#6530=CARTESIAN_POINT('Ctrl Pts',(-11.0878897426906,1.39740430473757,-1.));
#6531=CARTESIAN_POINT('Ctrl Pts',(-11.1418270749817,1.36117027439398,-1.));
#6532=CARTESIAN_POINT('Ctrl Pts',(-11.1955970312291,1.32435651843207,-1.));
#6533=CARTESIAN_POINT('Ctrl Pts',(-11.2491956455455,1.28696685552412,-1.));
#6534=CARTESIAN_POINT('Ctrl Pts',(-11.30261917075,1.24900490126928,-1.));
#6535=CARTESIAN_POINT('Ctrl Pts',(-11.3558638941869,1.21047418192819,-1.));
#6536=CARTESIAN_POINT('Ctrl Pts',(-11.4089259705106,1.17137823760545,-1.));
#6537=CARTESIAN_POINT('Ctrl Pts',(-11.4618012771636,1.13172071766774,-1.));
#6538=CARTESIAN_POINT('Ctrl Pts',(-11.5144851912285,1.09150552381395,-1.));
#6539=CARTESIAN_POINT('Ctrl Pts',(-11.5669726710206,1.05073678224335,-1.));
#6540=CARTESIAN_POINT('Ctrl Pts',(-11.6192586585895,1.00941863307588,-1.));
#6541=CARTESIAN_POINT('Ctrl Pts',(-11.6713384077523,0.967555069553195,-1.));
#6542=CARTESIAN_POINT('Ctrl Pts',(-11.7232078225909,0.925149766751162,-1.));
#6543=CARTESIAN_POINT('Ctrl Pts',(-11.7748638454684,0.882205904336898,-1.));
#6544=CARTESIAN_POINT('Ctrl Pts',(-11.8263046631092,0.838726039995983,-1.));
#6545=CARTESIAN_POINT('Ctrl Pts',(-11.877529348846,0.794712140666327,-1.));
#6546=CARTESIAN_POINT('Ctrl Pts',(-11.9183359560736,0.759074898533419,-1.));
#6547=CARTESIAN_POINT('Ctrl Pts',(-11.9488435391885,0.732107639766311,-1.));
#6548=CARTESIAN_POINT('Ctrl Pts',(-11.9691386658393,0.714023134927412,-1.));
#6549=CARTESIAN_POINT('Ctrl Pts',(-11.9792754136349,0.70495429942753,-1.));
#6550=CARTESIAN_POINT('Ctrl Pts',(-8.13553012180811,2.31040030805735,6.));
#6551=CARTESIAN_POINT('Ctrl Pts',(-8.14597432907962,2.31336634706602,6.));
#6552=CARTESIAN_POINT('Ctrl Pts',(-8.16694940973767,2.31883955953704,6.));
#6553=CARTESIAN_POINT('Ctrl Pts',(-8.19867202257948,2.32567282066756,6.));
#6554=CARTESIAN_POINT('Ctrl Pts',(-8.24146380440172,2.33217339857874,6.));
#6555=CARTESIAN_POINT('Ctrl Pts',(-8.29563322262998,2.33676998946179,6.));
#6556=CARTESIAN_POINT('Ctrl Pts',(-8.35029826768635,2.33886640526142,6.));
#6557=CARTESIAN_POINT('Ctrl Pts',(-8.40527692606173,2.33945961175101,6.));
#6558=CARTESIAN_POINT('Ctrl Pts',(-8.46043689627596,2.3392342622836,6.));
#6559=CARTESIAN_POINT('Ctrl Pts',(-8.51572283259063,2.33840535058003,6.));
#6560=CARTESIAN_POINT('Ctrl Pts',(-8.57112741281372,2.33689888190034,6.));
#6561=CARTESIAN_POINT('Ctrl Pts',(-8.62667187892838,2.33447589689188,6.));
#6562=CARTESIAN_POINT('Ctrl Pts',(-8.68238458286971,2.33086762045752,6.));
#6563=CARTESIAN_POINT('Ctrl Pts',(-8.73827625692193,2.32593252219559,6.));
#6564=CARTESIAN_POINT('Ctrl Pts',(-8.79433301721166,2.31969862084206,6.));
#6565=CARTESIAN_POINT('Ctrl Pts',(-8.85052793120604,2.31228619203479,6.));
#6566=CARTESIAN_POINT('Ctrl Pts',(-8.90682777405608,2.30386137247017,6.));
#6567=CARTESIAN_POINT('Ctrl Pts',(-8.96320109950669,2.29458154408801,6.));
#6568=CARTESIAN_POINT('Ctrl Pts',(-9.0196273647496,2.28453333318601,6.));
#6569=CARTESIAN_POINT('Ctrl Pts',(-9.07609679780011,2.27373321015996,6.));
#6570=CARTESIAN_POINT('Ctrl Pts',(-9.13260588645235,2.26215759393014,6.));
#6571=CARTESIAN_POINT('Ctrl Pts',(-9.18915420809356,2.24976392906278,6.));
#6572=CARTESIAN_POINT('Ctrl Pts',(-9.24574089753053,2.23651421201962,6.));
#6573=CARTESIAN_POINT('Ctrl Pts',(-9.30236077039476,2.22240082168223,6.));
#6574=CARTESIAN_POINT('Ctrl Pts',(-9.35900502856467,2.2074416540289,6.));
#6575=CARTESIAN_POINT('Ctrl Pts',(-9.41566291502215,2.19166889809877,6.));
#6576=CARTESIAN_POINT('Ctrl Pts',(-9.4723230488593,2.17511995998945,6.));
#6577=CARTESIAN_POINT('Ctrl Pts',(-9.52897485563506,2.15782775391113,6.));
#6578=CARTESIAN_POINT('Ctrl Pts',(-9.58561005875903,2.13981058538588,6.));
#6579=CARTESIAN_POINT('Ctrl Pts',(-9.64222216484242,2.12107554726937,6.));
#6580=CARTESIAN_POINT('Ctrl Pts',(-9.69880579601398,2.10162295100989,6.));
#6581=CARTESIAN_POINT('Ctrl Pts',(-9.75535607889872,2.08145038176733,6.));
#6582=CARTESIAN_POINT('Ctrl Pts',(-9.81186801391803,2.06055689146528,6.));
#6583=CARTESIAN_POINT('Ctrl Pts',(-9.86833584478527,2.03894719582859,6.));
#6584=CARTESIAN_POINT('Ctrl Pts',(-9.92475330165988,2.01663001707736,6.));
#6585=CARTESIAN_POINT('Ctrl Pts',(-9.98111385659409,1.99361634997092,6.));
#6586=CARTESIAN_POINT('Ctrl Pts',(-10.037410974034,1.96991776698621,6.));
#6587=CARTESIAN_POINT('Ctrl Pts',(-10.0936383641523,1.94554471072257,6.));
#6588=CARTESIAN_POINT('Ctrl Pts',(-10.1497902344364,1.92050480406378,6.));
#6589=CARTESIAN_POINT('Ctrl Pts',(-10.2058611678956,1.89480360265125,6.));
#6590=CARTESIAN_POINT('Ctrl Pts',(-10.2618460035706,1.86844533887956,6.));
#6591=CARTESIAN_POINT('Ctrl Pts',(-10.317739716759,1.84143367405763,6.));
#6592=CARTESIAN_POINT('Ctrl Pts',(-10.3735373011506,1.81377244526719,6.));
#6593=CARTESIAN_POINT('Ctrl Pts',(-10.4292336483793,1.78546643461776,6.));
#6594=CARTESIAN_POINT('Ctrl Pts',(-10.4848236013528,1.75652107004318,6.));
#6595=CARTESIAN_POINT('Ctrl Pts',(-10.5403020105194,1.72694211360793,6.));
#6596=CARTESIAN_POINT('Ctrl Pts',(-10.59566379085,1.69673535547185,6.));
#6597=CARTESIAN_POINT('Ctrl Pts',(-10.6509039769739,1.66590631967585,6.));
#6598=CARTESIAN_POINT('Ctrl Pts',(-10.7060177866027,1.63445994423349,6.));
#6599=CARTESIAN_POINT('Ctrl Pts',(-10.761000572936,1.60240070038749,6.));
#6600=CARTESIAN_POINT('Ctrl Pts',(-10.8158477697972,1.56973274862052,6.));
#6601=CARTESIAN_POINT('Ctrl Pts',(-10.8705548380775,1.53646008988796,6.));
#6602=CARTESIAN_POINT('Ctrl Pts',(-10.9251172180581,1.50258671261028,6.));
#6603=CARTESIAN_POINT('Ctrl Pts',(-10.9795302662584,1.46811677324654,6.));
#6604=CARTESIAN_POINT('Ctrl Pts',(-11.033789312906,1.43305454241432,6.));
#6605=CARTESIAN_POINT('Ctrl Pts',(-11.0878897426906,1.39740430473757,6.));
#6606=CARTESIAN_POINT('Ctrl Pts',(-11.1418270749817,1.36117027439398,6.));
#6607=CARTESIAN_POINT('Ctrl Pts',(-11.1955970312291,1.32435651843207,6.));
#6608=CARTESIAN_POINT('Ctrl Pts',(-11.2491956455455,1.28696685552412,6.));
#6609=CARTESIAN_POINT('Ctrl Pts',(-11.30261917075,1.24900490126928,6.));
#6610=CARTESIAN_POINT('Ctrl Pts',(-11.3558638941869,1.21047418192819,6.));
#6611=CARTESIAN_POINT('Ctrl Pts',(-11.4089259705106,1.17137823760545,6.));
#6612=CARTESIAN_POINT('Ctrl Pts',(-11.4618012771636,1.13172071766774,6.));
#6613=CARTESIAN_POINT('Ctrl Pts',(-11.5144851912285,1.09150552381395,6.));
#6614=CARTESIAN_POINT('Ctrl Pts',(-11.5669726710206,1.05073678224335,6.));
#6615=CARTESIAN_POINT('Ctrl Pts',(-11.6192586585895,1.00941863307588,6.));
#6616=CARTESIAN_POINT('Ctrl Pts',(-11.6713384077523,0.967555069553195,6.));
#6617=CARTESIAN_POINT('Ctrl Pts',(-11.7232078225909,0.925149766751162,6.));
#6618=CARTESIAN_POINT('Ctrl Pts',(-11.7748638454684,0.882205904336898,6.));
#6619=CARTESIAN_POINT('Ctrl Pts',(-11.8263046631092,0.838726039995983,6.));
#6620=CARTESIAN_POINT('Ctrl Pts',(-11.877529348846,0.794712140666327,6.));
#6621=CARTESIAN_POINT('Ctrl Pts',(-11.9183359560736,0.759074898533419,6.));
#6622=CARTESIAN_POINT('Ctrl Pts',(-11.9488435391885,0.732107639766311,6.));
#6623=CARTESIAN_POINT('Ctrl Pts',(-11.9691386658393,0.714023134927412,6.));
#6624=CARTESIAN_POINT('Ctrl Pts',(-11.9792754136349,0.70495429942753,6.));
#6625=CARTESIAN_POINT('Ctrl Pts',(-6.60014603862877,10.0218796774244,-3.75));
#6626=CARTESIAN_POINT('Ctrl Pts',(-6.60014603862877,10.0218796774244,12.75));
#6627=CARTESIAN_POINT('Ctrl Pts',(-6.60293150665659,10.0085665785717,-3.75));
#6628=CARTESIAN_POINT('Ctrl Pts',(-6.60293150665659,10.0085665785717,12.75));
#6629=CARTESIAN_POINT('Ctrl Pts',(-6.60844558393656,9.98194823089968,-3.75));
#6630=CARTESIAN_POINT('Ctrl Pts',(-6.60844558393656,9.98194823089968,12.75));
#6631=CARTESIAN_POINT('Ctrl Pts',(-6.61654612354183,9.94204425953052,-3.75));
#6632=CARTESIAN_POINT('Ctrl Pts',(-6.61654612354183,9.94204425953052,12.75));
#6633=CARTESIAN_POINT('Ctrl Pts',(-6.62700557693596,9.88888607996273,-3.75));
#6634=CARTESIAN_POINT('Ctrl Pts',(-6.62700557693596,9.88888607996273,12.75));
#6635=CARTESIAN_POINT('Ctrl Pts',(-6.63951038900666,9.82251725114898,-3.75));
#6636=CARTESIAN_POINT('Ctrl Pts',(-6.63951038900666,9.82251725114898,12.75));
#6637=CARTESIAN_POINT('Ctrl Pts',(-6.65144464725859,9.75622826411013,-3.75));
#6638=CARTESIAN_POINT('Ctrl Pts',(-6.65144464725859,9.75622826411013,12.75));
#6639=CARTESIAN_POINT('Ctrl Pts',(-6.66280711160719,9.69002090483258,-3.75));
#6640=CARTESIAN_POINT('Ctrl Pts',(-6.66280711160719,9.69002090483258,12.75));
#6641=CARTESIAN_POINT('Ctrl Pts',(-6.67359647366961,9.62389802250188,-3.75));
#6642=CARTESIAN_POINT('Ctrl Pts',(-6.67359647366961,9.62389802250188,12.75));
#6643=CARTESIAN_POINT('Ctrl Pts',(-6.68381150859182,9.55786385494286,-3.75));
#6644=CARTESIAN_POINT('Ctrl Pts',(-6.68381150859182,9.55786385494286,12.75));
#6645=CARTESIAN_POINT('Ctrl Pts',(-6.69345108162377,9.49192378686253,-3.75));
#6646=CARTESIAN_POINT('Ctrl Pts',(-6.69345108162377,9.49192378686253,12.75));
#6647=CARTESIAN_POINT('Ctrl Pts',(-6.70251410760819,9.42608392519667,-3.75));
#6648=CARTESIAN_POINT('Ctrl Pts',(-6.70251410760819,9.42608392519667,12.75));
#6649=CARTESIAN_POINT('Ctrl Pts',(-6.71099953007123,9.36035072031876,-3.75));
#6650=CARTESIAN_POINT('Ctrl Pts',(-6.71099953007123,9.36035072031876,12.75));
#6651=CARTESIAN_POINT('Ctrl Pts',(-6.71890629646186,9.2947306015555,-3.75));
#6652=CARTESIAN_POINT('Ctrl Pts',(-6.71890629646186,9.2947306015555,12.75));
#6653=CARTESIAN_POINT('Ctrl Pts',(-6.72623333926845,9.22922952332026,-3.75));
#6654=CARTESIAN_POINT('Ctrl Pts',(-6.72623333926845,9.22922952332026,12.75));
#6655=CARTESIAN_POINT('Ctrl Pts',(-6.73297955932547,9.16385288053588,-3.75));
#6656=CARTESIAN_POINT('Ctrl Pts',(-6.73297955932547,9.16385288053588,12.75));
#6657=CARTESIAN_POINT('Ctrl Pts',(-6.73914381348523,9.09860577342166,-3.75));
#6658=CARTESIAN_POINT('Ctrl Pts',(-6.73914381348523,9.09860577342166,12.75));
#6659=CARTESIAN_POINT('Ctrl Pts',(-6.74472490424422,9.03349318036199,-3.75));
#6660=CARTESIAN_POINT('Ctrl Pts',(-6.74472490424422,9.03349318036199,12.75));
#6661=CARTESIAN_POINT('Ctrl Pts',(-6.74972157399229,8.96852015431046,-3.75));
#6662=CARTESIAN_POINT('Ctrl Pts',(-6.74972157399229,8.96852015431046,12.75));
#6663=CARTESIAN_POINT('Ctrl Pts',(-6.75413249860576,8.90369203916218,-3.75));
#6664=CARTESIAN_POINT('Ctrl Pts',(-6.75413249860576,8.90369203916218,12.75));
#6665=CARTESIAN_POINT('Ctrl Pts',(-6.75795629519249,8.83901457377471,-3.75));
#6666=CARTESIAN_POINT('Ctrl Pts',(-6.75795629519249,8.83901457377471,12.75));
#6667=CARTESIAN_POINT('Ctrl Pts',(-6.76119155448275,8.77449374557664,-3.75));
#6668=CARTESIAN_POINT('Ctrl Pts',(-6.76119155448275,8.77449374557664,12.75));
#6669=CARTESIAN_POINT('Ctrl Pts',(-6.76383687353852,8.71013569385599,-3.75));
#6670=CARTESIAN_POINT('Ctrl Pts',(-6.76383687353852,8.71013569385599,12.75));
#6671=CARTESIAN_POINT('Ctrl Pts',(-6.76589088878265,8.64594659806298,-3.75));
#6672=CARTESIAN_POINT('Ctrl Pts',(-6.76589088878265,8.64594659806298,12.75));
#6673=CARTESIAN_POINT('Ctrl Pts',(-6.76735232235634,8.5819325577994,-3.75));
#6674=CARTESIAN_POINT('Ctrl Pts',(-6.76735232235634,8.5819325577994,12.75));
#6675=CARTESIAN_POINT('Ctrl Pts',(-6.76822000004555,8.51809951610774,-3.75));
#6676=CARTESIAN_POINT('Ctrl Pts',(-6.76822000004555,8.51809951610774,12.75));
#6677=CARTESIAN_POINT('Ctrl Pts',(-6.76849272647565,8.45445340444926,-3.75));
#6678=CARTESIAN_POINT('Ctrl Pts',(-6.76849272647565,8.45445340444926,12.75));
#6679=CARTESIAN_POINT('Ctrl Pts',(-6.76816918165128,8.39100025749018,-3.75));
#6680=CARTESIAN_POINT('Ctrl Pts',(-6.76816918165128,8.39100025749018,12.75));
#6681=CARTESIAN_POINT('Ctrl Pts',(-6.76724781676282,8.32774633509908,-3.75));
#6682=CARTESIAN_POINT('Ctrl Pts',(-6.76724781676282,8.32774633509908,12.75));
#6683=CARTESIAN_POINT('Ctrl Pts',(-6.76572674650935,8.26469824786603,-3.75));
#6684=CARTESIAN_POINT('Ctrl Pts',(-6.76572674650935,8.26469824786603,12.75));
#6685=CARTESIAN_POINT('Ctrl Pts',(-6.7636036696164,8.20186305794855,-3.75));
#6686=CARTESIAN_POINT('Ctrl Pts',(-6.7636036696164,8.20186305794855,12.75));
#6687=CARTESIAN_POINT('Ctrl Pts',(-6.76087611417306,8.13924806419107,-3.75));
#6688=CARTESIAN_POINT('Ctrl Pts',(-6.76087611417306,8.13924806419107,12.75));
#6689=CARTESIAN_POINT('Ctrl Pts',(-6.75754166486089,8.07686060726828,-3.75));
#6690=CARTESIAN_POINT('Ctrl Pts',(-6.75754166486089,8.07686060726828,12.75));
#6691=CARTESIAN_POINT('Ctrl Pts',(-6.75359819949754,8.01470786732019,-3.75));
#6692=CARTESIAN_POINT('Ctrl Pts',(-6.75359819949754,8.01470786732019,12.75));
#6693=CARTESIAN_POINT('Ctrl Pts',(-6.7490441308376,7.95279665937614,-3.75));
#6694=CARTESIAN_POINT('Ctrl Pts',(-6.7490441308376,7.95279665937614,12.75));
#6695=CARTESIAN_POINT('Ctrl Pts',(-6.74387863902608,7.89113323756913,-3.75));
#6696=CARTESIAN_POINT('Ctrl Pts',(-6.74387863902608,7.89113323756913,12.75));
#6697=CARTESIAN_POINT('Ctrl Pts',(-6.73810106562748,7.82972378407324,-3.75));
#6698=CARTESIAN_POINT('Ctrl Pts',(-6.73810106562748,7.82972378407324,12.75));
#6699=CARTESIAN_POINT('Ctrl Pts',(-6.73171032576035,7.76857488460784,-3.75));
#6700=CARTESIAN_POINT('Ctrl Pts',(-6.73171032576035,7.76857488460784,12.75));
#6701=CARTESIAN_POINT('Ctrl Pts',(-6.72470431659336,7.70769400824503,-3.75));
#6702=CARTESIAN_POINT('Ctrl Pts',(-6.72470431659336,7.70769400824503,12.75));
#6703=CARTESIAN_POINT('Ctrl Pts',(-6.71707933277187,7.6470899828899,-3.75));
#6704=CARTESIAN_POINT('Ctrl Pts',(-6.71707933277187,7.6470899828899,12.75));
#6705=CARTESIAN_POINT('Ctrl Pts',(-6.70882947565318,7.58677347699226,-3.75));
#6706=CARTESIAN_POINT('Ctrl Pts',(-6.70882947565318,7.58677347699226,12.75));
#6707=CARTESIAN_POINT('Ctrl Pts',(-6.69994799095524,7.52675593674632,-3.75));
#6708=CARTESIAN_POINT('Ctrl Pts',(-6.69994799095524,7.52675593674632,12.75));
#6709=CARTESIAN_POINT('Ctrl Pts',(-6.69042862091104,7.46704851290034,-3.75));
#6710=CARTESIAN_POINT('Ctrl Pts',(-6.69042862091104,7.46704851290034,12.75));
#6711=CARTESIAN_POINT('Ctrl Pts',(-6.68026694677668,7.40766099640558,-3.75));
#6712=CARTESIAN_POINT('Ctrl Pts',(-6.68026694677668,7.40766099640558,12.75));
#6713=CARTESIAN_POINT('Ctrl Pts',(-6.66946176275797,7.34860073021492,-3.75));
#6714=CARTESIAN_POINT('Ctrl Pts',(-6.66946176275797,7.34860073021492,12.75));
#6715=CARTESIAN_POINT('Ctrl Pts',(-6.65801638970246,7.28987157005224,-3.75));
#6716=CARTESIAN_POINT('Ctrl Pts',(-6.65801638970246,7.28987157005224,12.75));
#6717=CARTESIAN_POINT('Ctrl Pts',(-6.64593535561053,7.23147652896403,-3.75));
#6718=CARTESIAN_POINT('Ctrl Pts',(-6.64593535561053,7.23147652896403,12.75));
#6719=CARTESIAN_POINT('Ctrl Pts',(-6.63322107969569,7.17342042004756,-3.75));
#6720=CARTESIAN_POINT('Ctrl Pts',(-6.63322107969569,7.17342042004756,12.75));
#6721=CARTESIAN_POINT('Ctrl Pts',(-6.6198706660591,7.1157124131703,-3.75));
#6722=CARTESIAN_POINT('Ctrl Pts',(-6.6198706660591,7.1157124131703,12.75));
#6723=CARTESIAN_POINT('Ctrl Pts',(-6.60587239994885,7.05836882883084,-3.75));
#6724=CARTESIAN_POINT('Ctrl Pts',(-6.60587239994885,7.05836882883084,12.75));
#6725=CARTESIAN_POINT('Ctrl Pts',(-6.5912030640433,7.00141528186886,-3.75));
#6726=CARTESIAN_POINT('Ctrl Pts',(-6.5912030640433,7.00141528186886,12.75));
#6727=CARTESIAN_POINT('Ctrl Pts',(-6.5758359541656,6.94488033148854,-3.75));
#6728=CARTESIAN_POINT('Ctrl Pts',(-6.5758359541656,6.94488033148854,12.75));
#6729=CARTESIAN_POINT('Ctrl Pts',(-6.55974857229919,6.88878938806037,-3.75));
#6730=CARTESIAN_POINT('Ctrl Pts',(-6.55974857229919,6.88878938806037,12.75));
#6731=CARTESIAN_POINT('Ctrl Pts',(-6.54292981913304,6.83315901897031,-3.75));
#6732=CARTESIAN_POINT('Ctrl Pts',(-6.54292981913304,6.83315901897031,12.75));
#6733=CARTESIAN_POINT('Ctrl Pts',(-6.52538888693355,6.77798990345397,-3.75));
#6734=CARTESIAN_POINT('Ctrl Pts',(-6.52538888693355,6.77798990345397,12.75));
#6735=CARTESIAN_POINT('Ctrl Pts',(-6.50715912032692,6.72326378902152,-3.75));
#6736=CARTESIAN_POINT('Ctrl Pts',(-6.50715912032692,6.72326378902152,12.75));
#6737=CARTESIAN_POINT('Ctrl Pts',(-6.48827758470622,6.66895976394944,-3.75));
#6738=CARTESIAN_POINT('Ctrl Pts',(-6.48827758470622,6.66895976394944,12.75));
#6739=CARTESIAN_POINT('Ctrl Pts',(-6.46876645798849,6.6150690793574,-3.75));
#6740=CARTESIAN_POINT('Ctrl Pts',(-6.46876645798849,6.6150690793574,12.75));
#6741=CARTESIAN_POINT('Ctrl Pts',(-6.44861636238489,6.56160843323028,-3.75));
#6742=CARTESIAN_POINT('Ctrl Pts',(-6.44861636238489,6.56160843323028,12.75));
#6743=CARTESIAN_POINT('Ctrl Pts',(-6.42776254872513,6.50863892931077,-3.75));
#6744=CARTESIAN_POINT('Ctrl Pts',(-6.42776254872513,6.50863892931077,12.75));
#6745=CARTESIAN_POINT('Ctrl Pts',(-6.40608444337878,6.45626649182453,-3.75));
#6746=CARTESIAN_POINT('Ctrl Pts',(-6.40608444337878,6.45626649182453,12.75));
#6747=CARTESIAN_POINT('Ctrl Pts',(-6.38345478017075,6.404602962683,-3.75));
#6748=CARTESIAN_POINT('Ctrl Pts',(-6.38345478017075,6.404602962683,12.75));
#6749=CARTESIAN_POINT('Ctrl Pts',(-6.35978286360965,6.35373180396277,-3.75));
#6750=CARTESIAN_POINT('Ctrl Pts',(-6.35978286360965,6.35373180396277,12.75));
#6751=CARTESIAN_POINT('Ctrl Pts',(-6.33505137069502,6.30367904881887,-3.75));
#6752=CARTESIAN_POINT('Ctrl Pts',(-6.33505137069502,6.30367904881887,12.75));
#6753=CARTESIAN_POINT('Ctrl Pts',(-6.30937750420801,6.2543646376197,-3.75));
#6754=CARTESIAN_POINT('Ctrl Pts',(-6.30937750420801,6.2543646376197,12.75));
#6755=CARTESIAN_POINT('Ctrl Pts',(-6.28297985424307,6.20562962932065,-3.75));
#6756=CARTESIAN_POINT('Ctrl Pts',(-6.28297985424307,6.20562962932065,12.75));
#6757=CARTESIAN_POINT('Ctrl Pts',(-6.25605474467853,6.15733614814836,-3.75));
#6758=CARTESIAN_POINT('Ctrl Pts',(-6.25605474467853,6.15733614814836,12.75));
#6759=CARTESIAN_POINT('Ctrl Pts',(-6.22866991793491,6.10945353793714,-3.75));
#6760=CARTESIAN_POINT('Ctrl Pts',(-6.22866991793491,6.10945353793714,12.75));
#6761=CARTESIAN_POINT('Ctrl Pts',(-6.20066685685755,6.06213722636286,-3.75));
#6762=CARTESIAN_POINT('Ctrl Pts',(-6.20066685685755,6.06213722636286,12.75));
#6763=CARTESIAN_POINT('Ctrl Pts',(-6.17151878498999,6.01584411654484,-3.75));
#6764=CARTESIAN_POINT('Ctrl Pts',(-6.17151878498999,6.01584411654484,12.75));
#6765=CARTESIAN_POINT('Ctrl Pts',(-6.14045331140033,5.97123031969247,-3.75));
#6766=CARTESIAN_POINT('Ctrl Pts',(-6.14045331140033,5.97123031969247,12.75));
#6767=CARTESIAN_POINT('Ctrl Pts',(-6.11342775487885,5.9374218385168,-3.75));
#6768=CARTESIAN_POINT('Ctrl Pts',(-6.11342775487885,5.9374218385168,12.75));
#6769=CARTESIAN_POINT('Ctrl Pts',(-6.09164867072823,5.91336588048663,-3.75));
#6770=CARTESIAN_POINT('Ctrl Pts',(-6.09164867072823,5.91336588048663,12.75));
#6771=CARTESIAN_POINT('Ctrl Pts',(-6.07642118935899,5.89793753402585,-3.75));
#6772=CARTESIAN_POINT('Ctrl Pts',(-6.07642118935899,5.89793753402585,12.75));
#6773=CARTESIAN_POINT('Ctrl Pts',(-6.06863042059311,5.89037560471066,-3.75));
#6774=CARTESIAN_POINT('Ctrl Pts',(-6.06863042059311,5.89037560471066,12.75));
#6775=CARTESIAN_POINT('',(-6.60014603862874,10.0218796774245,-1.));
#6776=CARTESIAN_POINT('Ctrl Pts',(-6.60014603862877,10.0218796774244,-1.));
#6777=CARTESIAN_POINT('Ctrl Pts',(-6.60293150665659,10.0085665785717,-1.));
#6778=CARTESIAN_POINT('Ctrl Pts',(-6.60844558393656,9.98194823089968,-1.));
#6779=CARTESIAN_POINT('Ctrl Pts',(-6.61654612354183,9.94204425953052,-1.));
#6780=CARTESIAN_POINT('Ctrl Pts',(-6.62700557693596,9.88888607996273,-1.));
#6781=CARTESIAN_POINT('Ctrl Pts',(-6.63951038900666,9.82251725114898,-1.));
#6782=CARTESIAN_POINT('Ctrl Pts',(-6.65144464725859,9.75622826411013,-1.));
#6783=CARTESIAN_POINT('Ctrl Pts',(-6.66280711160719,9.69002090483258,-1.));
#6784=CARTESIAN_POINT('Ctrl Pts',(-6.67359647366961,9.62389802250188,-1.));
#6785=CARTESIAN_POINT('Ctrl Pts',(-6.68381150859182,9.55786385494286,-1.));
#6786=CARTESIAN_POINT('Ctrl Pts',(-6.69345108162377,9.49192378686253,-1.));
#6787=CARTESIAN_POINT('Ctrl Pts',(-6.70251410760819,9.42608392519667,-1.));
#6788=CARTESIAN_POINT('Ctrl Pts',(-6.71099953007123,9.36035072031876,-1.));
#6789=CARTESIAN_POINT('Ctrl Pts',(-6.71890629646186,9.2947306015555,-1.));
#6790=CARTESIAN_POINT('Ctrl Pts',(-6.72623333926845,9.22922952332026,-1.));
#6791=CARTESIAN_POINT('Ctrl Pts',(-6.73297955932547,9.16385288053588,-1.));
#6792=CARTESIAN_POINT('Ctrl Pts',(-6.73914381348523,9.09860577342166,-1.));
#6793=CARTESIAN_POINT('Ctrl Pts',(-6.74472490424422,9.03349318036199,-1.));
#6794=CARTESIAN_POINT('Ctrl Pts',(-6.74972157399229,8.96852015431046,-1.));
#6795=CARTESIAN_POINT('Ctrl Pts',(-6.75413249860576,8.90369203916218,-1.));
#6796=CARTESIAN_POINT('Ctrl Pts',(-6.75795629519249,8.83901457377471,-1.));
#6797=CARTESIAN_POINT('Ctrl Pts',(-6.76119155448275,8.77449374557664,-1.));
#6798=CARTESIAN_POINT('Ctrl Pts',(-6.76383687353852,8.71013569385599,-1.));
#6799=CARTESIAN_POINT('Ctrl Pts',(-6.76589088878265,8.64594659806298,-1.));
#6800=CARTESIAN_POINT('Ctrl Pts',(-6.76735232235634,8.5819325577994,-1.));
#6801=CARTESIAN_POINT('Ctrl Pts',(-6.76822000004555,8.51809951610774,-1.));
#6802=CARTESIAN_POINT('Ctrl Pts',(-6.76849272647565,8.45445340444926,-1.));
#6803=CARTESIAN_POINT('Ctrl Pts',(-6.76816918165128,8.39100025749018,-1.));
#6804=CARTESIAN_POINT('Ctrl Pts',(-6.76724781676282,8.32774633509908,-1.));
#6805=CARTESIAN_POINT('Ctrl Pts',(-6.76572674650935,8.26469824786603,-1.));
#6806=CARTESIAN_POINT('Ctrl Pts',(-6.7636036696164,8.20186305794855,-1.));
#6807=CARTESIAN_POINT('Ctrl Pts',(-6.76087611417306,8.13924806419107,-1.));
#6808=CARTESIAN_POINT('Ctrl Pts',(-6.75754166486089,8.07686060726828,-1.));
#6809=CARTESIAN_POINT('Ctrl Pts',(-6.75359819949754,8.01470786732019,-1.));
#6810=CARTESIAN_POINT('Ctrl Pts',(-6.7490441308376,7.95279665937614,-1.));
#6811=CARTESIAN_POINT('Ctrl Pts',(-6.74387863902608,7.89113323756913,-1.));
#6812=CARTESIAN_POINT('Ctrl Pts',(-6.73810106562748,7.82972378407324,-1.));
#6813=CARTESIAN_POINT('Ctrl Pts',(-6.73171032576035,7.76857488460784,-1.));
#6814=CARTESIAN_POINT('Ctrl Pts',(-6.72470431659336,7.70769400824503,-1.));
#6815=CARTESIAN_POINT('Ctrl Pts',(-6.71707933277187,7.6470899828899,-1.));
#6816=CARTESIAN_POINT('Ctrl Pts',(-6.70882947565318,7.58677347699226,-1.));
#6817=CARTESIAN_POINT('Ctrl Pts',(-6.69994799095524,7.52675593674632,-1.));
#6818=CARTESIAN_POINT('Ctrl Pts',(-6.69042862091104,7.46704851290034,-1.));
#6819=CARTESIAN_POINT('Ctrl Pts',(-6.68026694677668,7.40766099640558,-1.));
#6820=CARTESIAN_POINT('Ctrl Pts',(-6.66946176275797,7.34860073021492,-1.));
#6821=CARTESIAN_POINT('Ctrl Pts',(-6.65801638970246,7.28987157005224,-1.));
#6822=CARTESIAN_POINT('Ctrl Pts',(-6.64593535561053,7.23147652896403,-1.));
#6823=CARTESIAN_POINT('Ctrl Pts',(-6.63322107969569,7.17342042004756,-1.));
#6824=CARTESIAN_POINT('Ctrl Pts',(-6.6198706660591,7.1157124131703,-1.));
#6825=CARTESIAN_POINT('Ctrl Pts',(-6.60587239994885,7.05836882883084,-1.));
#6826=CARTESIAN_POINT('Ctrl Pts',(-6.5912030640433,7.00141528186886,-1.));
#6827=CARTESIAN_POINT('Ctrl Pts',(-6.5758359541656,6.94488033148854,-1.));
#6828=CARTESIAN_POINT('Ctrl Pts',(-6.55974857229919,6.88878938806037,-1.));
#6829=CARTESIAN_POINT('Ctrl Pts',(-6.54292981913304,6.83315901897031,-1.));
#6830=CARTESIAN_POINT('Ctrl Pts',(-6.52538888693355,6.77798990345397,-1.));
#6831=CARTESIAN_POINT('Ctrl Pts',(-6.50715912032692,6.72326378902152,-1.));
#6832=CARTESIAN_POINT('Ctrl Pts',(-6.48827758470622,6.66895976394944,-1.));
#6833=CARTESIAN_POINT('Ctrl Pts',(-6.46876645798849,6.6150690793574,-1.));
#6834=CARTESIAN_POINT('Ctrl Pts',(-6.44861636238489,6.56160843323028,-1.));
#6835=CARTESIAN_POINT('Ctrl Pts',(-6.42776254872513,6.50863892931077,-1.));
#6836=CARTESIAN_POINT('Ctrl Pts',(-6.40608444337878,6.45626649182453,-1.));
#6837=CARTESIAN_POINT('Ctrl Pts',(-6.38345478017075,6.404602962683,-1.));
#6838=CARTESIAN_POINT('Ctrl Pts',(-6.35978286360965,6.35373180396277,-1.));
#6839=CARTESIAN_POINT('Ctrl Pts',(-6.33505137069502,6.30367904881887,-1.));
#6840=CARTESIAN_POINT('Ctrl Pts',(-6.30937750420801,6.2543646376197,-1.));
#6841=CARTESIAN_POINT('Ctrl Pts',(-6.28297985424307,6.20562962932065,-1.));
#6842=CARTESIAN_POINT('Ctrl Pts',(-6.25605474467853,6.15733614814836,-1.));
#6843=CARTESIAN_POINT('Ctrl Pts',(-6.22866991793491,6.10945353793714,-1.));
#6844=CARTESIAN_POINT('Ctrl Pts',(-6.20066685685755,6.06213722636286,-1.));
#6845=CARTESIAN_POINT('Ctrl Pts',(-6.17151878498999,6.01584411654484,-1.));
#6846=CARTESIAN_POINT('Ctrl Pts',(-6.14045331140033,5.97123031969247,-1.));
#6847=CARTESIAN_POINT('Ctrl Pts',(-6.11342775487885,5.9374218385168,-1.));
#6848=CARTESIAN_POINT('Ctrl Pts',(-6.09164867072823,5.91336588048663,-1.));
#6849=CARTESIAN_POINT('Ctrl Pts',(-6.07642118935899,5.89793753402585,-1.));
#6850=CARTESIAN_POINT('Ctrl Pts',(-6.06863042059311,5.89037560471066,-1.));
#6851=CARTESIAN_POINT('',(-6.60014603862874,10.0218796774245,6.));
#6852=CARTESIAN_POINT('Ctrl Pts',(-6.60014603862877,10.0218796774244,6.));
#6853=CARTESIAN_POINT('Ctrl Pts',(-6.60293150665659,10.0085665785717,6.));
#6854=CARTESIAN_POINT('Ctrl Pts',(-6.60844558393656,9.98194823089968,6.));
#6855=CARTESIAN_POINT('Ctrl Pts',(-6.61654612354183,9.94204425953052,6.));
#6856=CARTESIAN_POINT('Ctrl Pts',(-6.62700557693596,9.88888607996273,6.));
#6857=CARTESIAN_POINT('Ctrl Pts',(-6.63951038900666,9.82251725114898,6.));
#6858=CARTESIAN_POINT('Ctrl Pts',(-6.65144464725859,9.75622826411013,6.));
#6859=CARTESIAN_POINT('Ctrl Pts',(-6.66280711160719,9.69002090483258,6.));
#6860=CARTESIAN_POINT('Ctrl Pts',(-6.67359647366961,9.62389802250188,6.));
#6861=CARTESIAN_POINT('Ctrl Pts',(-6.68381150859182,9.55786385494286,6.));
#6862=CARTESIAN_POINT('Ctrl Pts',(-6.69345108162377,9.49192378686253,6.));
#6863=CARTESIAN_POINT('Ctrl Pts',(-6.70251410760819,9.42608392519667,6.));
#6864=CARTESIAN_POINT('Ctrl Pts',(-6.71099953007123,9.36035072031876,6.));
#6865=CARTESIAN_POINT('Ctrl Pts',(-6.71890629646186,9.2947306015555,6.));
#6866=CARTESIAN_POINT('Ctrl Pts',(-6.72623333926845,9.22922952332026,6.));
#6867=CARTESIAN_POINT('Ctrl Pts',(-6.73297955932547,9.16385288053588,6.));
#6868=CARTESIAN_POINT('Ctrl Pts',(-6.73914381348523,9.09860577342166,6.));
#6869=CARTESIAN_POINT('Ctrl Pts',(-6.74472490424422,9.03349318036199,6.));
#6870=CARTESIAN_POINT('Ctrl Pts',(-6.74972157399229,8.96852015431046,6.));
#6871=CARTESIAN_POINT('Ctrl Pts',(-6.75413249860576,8.90369203916218,6.));
#6872=CARTESIAN_POINT('Ctrl Pts',(-6.75795629519249,8.83901457377471,6.));
#6873=CARTESIAN_POINT('Ctrl Pts',(-6.76119155448275,8.77449374557664,6.));
#6874=CARTESIAN_POINT('Ctrl Pts',(-6.76383687353852,8.71013569385599,6.));
#6875=CARTESIAN_POINT('Ctrl Pts',(-6.76589088878265,8.64594659806298,6.));
#6876=CARTESIAN_POINT('Ctrl Pts',(-6.76735232235634,8.5819325577994,6.));
#6877=CARTESIAN_POINT('Ctrl Pts',(-6.76822000004555,8.51809951610774,6.));
#6878=CARTESIAN_POINT('Ctrl Pts',(-6.76849272647565,8.45445340444926,6.));
#6879=CARTESIAN_POINT('Ctrl Pts',(-6.76816918165128,8.39100025749018,6.));
#6880=CARTESIAN_POINT('Ctrl Pts',(-6.76724781676282,8.32774633509908,6.));
#6881=CARTESIAN_POINT('Ctrl Pts',(-6.76572674650935,8.26469824786603,6.));
#6882=CARTESIAN_POINT('Ctrl Pts',(-6.7636036696164,8.20186305794855,6.));
#6883=CARTESIAN_POINT('Ctrl Pts',(-6.76087611417306,8.13924806419107,6.));
#6884=CARTESIAN_POINT('Ctrl Pts',(-6.75754166486089,8.07686060726828,6.));
#6885=CARTESIAN_POINT('Ctrl Pts',(-6.75359819949754,8.01470786732019,6.));
#6886=CARTESIAN_POINT('Ctrl Pts',(-6.7490441308376,7.95279665937614,6.));
#6887=CARTESIAN_POINT('Ctrl Pts',(-6.74387863902608,7.89113323756913,6.));
#6888=CARTESIAN_POINT('Ctrl Pts',(-6.73810106562748,7.82972378407324,6.));
#6889=CARTESIAN_POINT('Ctrl Pts',(-6.73171032576035,7.76857488460784,6.));
#6890=CARTESIAN_POINT('Ctrl Pts',(-6.72470431659336,7.70769400824503,6.));
#6891=CARTESIAN_POINT('Ctrl Pts',(-6.71707933277187,7.6470899828899,6.));
#6892=CARTESIAN_POINT('Ctrl Pts',(-6.70882947565318,7.58677347699226,6.));
#6893=CARTESIAN_POINT('Ctrl Pts',(-6.69994799095524,7.52675593674632,6.));
#6894=CARTESIAN_POINT('Ctrl Pts',(-6.69042862091104,7.46704851290034,6.));
#6895=CARTESIAN_POINT('Ctrl Pts',(-6.68026694677668,7.40766099640558,6.));
#6896=CARTESIAN_POINT('Ctrl Pts',(-6.66946176275797,7.34860073021492,6.));
#6897=CARTESIAN_POINT('Ctrl Pts',(-6.65801638970246,7.28987157005224,6.));
#6898=CARTESIAN_POINT('Ctrl Pts',(-6.64593535561053,7.23147652896403,6.));
#6899=CARTESIAN_POINT('Ctrl Pts',(-6.63322107969569,7.17342042004756,6.));
#6900=CARTESIAN_POINT('Ctrl Pts',(-6.6198706660591,7.1157124131703,6.));
#6901=CARTESIAN_POINT('Ctrl Pts',(-6.60587239994885,7.05836882883084,6.));
#6902=CARTESIAN_POINT('Ctrl Pts',(-6.5912030640433,7.00141528186886,6.));
#6903=CARTESIAN_POINT('Ctrl Pts',(-6.5758359541656,6.94488033148854,6.));
#6904=CARTESIAN_POINT('Ctrl Pts',(-6.55974857229919,6.88878938806037,6.));
#6905=CARTESIAN_POINT('Ctrl Pts',(-6.54292981913304,6.83315901897031,6.));
#6906=CARTESIAN_POINT('Ctrl Pts',(-6.52538888693355,6.77798990345397,6.));
#6907=CARTESIAN_POINT('Ctrl Pts',(-6.50715912032692,6.72326378902152,6.));
#6908=CARTESIAN_POINT('Ctrl Pts',(-6.48827758470622,6.66895976394944,6.));
#6909=CARTESIAN_POINT('Ctrl Pts',(-6.46876645798849,6.6150690793574,6.));
#6910=CARTESIAN_POINT('Ctrl Pts',(-6.44861636238489,6.56160843323028,6.));
#6911=CARTESIAN_POINT('Ctrl Pts',(-6.42776254872513,6.50863892931077,6.));
#6912=CARTESIAN_POINT('Ctrl Pts',(-6.40608444337878,6.45626649182453,6.));
#6913=CARTESIAN_POINT('Ctrl Pts',(-6.38345478017075,6.404602962683,6.));
#6914=CARTESIAN_POINT('Ctrl Pts',(-6.35978286360965,6.35373180396277,6.));
#6915=CARTESIAN_POINT('Ctrl Pts',(-6.33505137069502,6.30367904881887,6.));
#6916=CARTESIAN_POINT('Ctrl Pts',(-6.30937750420801,6.2543646376197,6.));
#6917=CARTESIAN_POINT('Ctrl Pts',(-6.28297985424307,6.20562962932065,6.));
#6918=CARTESIAN_POINT('Ctrl Pts',(-6.25605474467853,6.15733614814836,6.));
#6919=CARTESIAN_POINT('Ctrl Pts',(-6.22866991793491,6.10945353793714,6.));
#6920=CARTESIAN_POINT('Ctrl Pts',(-6.20066685685755,6.06213722636286,6.));
#6921=CARTESIAN_POINT('Ctrl Pts',(-6.17151878498999,6.01584411654484,6.));
#6922=CARTESIAN_POINT('Ctrl Pts',(-6.14045331140033,5.97123031969247,6.));
#6923=CARTESIAN_POINT('Ctrl Pts',(-6.11342775487885,5.9374218385168,6.));
#6924=CARTESIAN_POINT('Ctrl Pts',(-6.09164867072823,5.91336588048663,6.));
#6925=CARTESIAN_POINT('Ctrl Pts',(-6.07642118935899,5.89793753402585,6.));
#6926=CARTESIAN_POINT('Ctrl Pts',(-6.06863042059311,5.89037560471066,6.));
#6927=CARTESIAN_POINT('',(-6.60014603862874,10.0218796774245,0.));
#6928=CARTESIAN_POINT('Origin',(-1.99840144432528E-13,3.46133283549042E-13,
0.));
#6929=CARTESIAN_POINT('',(-5.37912937500617,10.726833976852,-1.));
#6930=CARTESIAN_POINT('Origin',(-1.99840144432528E-13,3.46133283549042E-13,
-1.));
#6931=CARTESIAN_POINT('',(-5.37912937500617,10.726833976852,6.));
#6932=CARTESIAN_POINT('Origin',(-1.99840144432528E-13,3.46133283549042E-13,
6.));
#6933=CARTESIAN_POINT('',(-5.37912937500617,10.726833976852,0.));
#6934=CARTESIAN_POINT('Ctrl Pts',(-2.066899701215,8.20077591276801,-3.75));
#6935=CARTESIAN_POINT('Ctrl Pts',(-2.066899701215,8.20077591276801,12.75));
#6936=CARTESIAN_POINT('Ctrl Pts',(-2.06955313972063,8.21130388109186,-3.75));
#6937=CARTESIAN_POINT('Ctrl Pts',(-2.06955313972063,8.21130388109186,12.75));
#6938=CARTESIAN_POINT('Ctrl Pts',(-2.07530073900944,8.23220544002367,-3.75));
#6939=CARTESIAN_POINT('Ctrl Pts',(-2.07530073900944,8.23220544002367,12.75));
#6940=CARTESIAN_POINT('Ctrl Pts',(-2.08524426770062,8.26309465918435,-3.75));
#6941=CARTESIAN_POINT('Ctrl Pts',(-2.08524426770062,8.26309465918435,12.75));
#6942=CARTESIAN_POINT('Ctrl Pts',(-2.10101049300138,8.3034037182712,-3.75));
#6943=CARTESIAN_POINT('Ctrl Pts',(-2.10101049300138,8.3034037182712,12.75));
#6944=CARTESIAN_POINT('Ctrl Pts',(-2.12411443763999,8.35261410600662,-3.75));
#6945=CARTESIAN_POINT('Ctrl Pts',(-2.12411443763999,8.35261410600662,12.75));
#6946=CARTESIAN_POINT('Ctrl Pts',(-2.1496314108288,8.40100363162428,-3.75));
#6947=CARTESIAN_POINT('Ctrl Pts',(-2.1496314108288,8.40100363162428,12.75));
#6948=CARTESIAN_POINT('Ctrl Pts',(-2.17660700812681,8.44891314968814,-3.75));
#6949=CARTESIAN_POINT('Ctrl Pts',(-2.17660700812681,8.44891314968814,12.75));
#6950=CARTESIAN_POINT('Ctrl Pts',(-2.20438215159743,8.49657041043196,-3.75));
#6951=CARTESIAN_POINT('Ctrl Pts',(-2.20438215159743,8.49657041043196,12.75));
#6952=CARTESIAN_POINT('Ctrl Pts',(-2.23274297834755,8.54403497990068,-3.75));
#6953=CARTESIAN_POINT('Ctrl Pts',(-2.23274297834755,8.54403497990068,12.75));
#6954=CARTESIAN_POINT('Ctrl Pts',(-2.26174990860571,8.59126351952004,-3.75));
#6955=CARTESIAN_POINT('Ctrl Pts',(-2.26174990860571,8.59126351952004,12.75));
#6956=CARTESIAN_POINT('Ctrl Pts',(-2.29162050823335,8.63815494571075,-3.75));
#6957=CARTESIAN_POINT('Ctrl Pts',(-2.29162050823335,8.63815494571075,12.75));
#6958=CARTESIAN_POINT('Ctrl Pts',(-2.32260171926006,8.68459942442029,-3.75));
#6959=CARTESIAN_POINT('Ctrl Pts',(-2.32260171926006,8.68459942442029,12.75));
#6960=CARTESIAN_POINT('Ctrl Pts',(-2.35482147675117,8.73053548487858,-3.75));
#6961=CARTESIAN_POINT('Ctrl Pts',(-2.35482147675117,8.73053548487858,12.75));
#6962=CARTESIAN_POINT('Ctrl Pts',(-2.38824857383288,8.77596511266658,-3.75));
#6963=CARTESIAN_POINT('Ctrl Pts',(-2.38824857383288,8.77596511266658,12.75));
#6964=CARTESIAN_POINT('Ctrl Pts',(-2.4227653824809,8.82092512134556,-3.75));
#6965=CARTESIAN_POINT('Ctrl Pts',(-2.4227653824809,8.82092512134556,12.75));
#6966=CARTESIAN_POINT('Ctrl Pts',(-2.45821141167118,8.86546980570045,-3.75));
#6967=CARTESIAN_POINT('Ctrl Pts',(-2.45821141167118,8.86546980570045,12.75));
#6968=CARTESIAN_POINT('Ctrl Pts',(-2.4944346415182,8.90965062344541,-3.75));
#6969=CARTESIAN_POINT('Ctrl Pts',(-2.4944346415182,8.90965062344541,12.75));
#6970=CARTESIAN_POINT('Ctrl Pts',(-2.53134978004337,8.95349309713545,-3.75));
#6971=CARTESIAN_POINT('Ctrl Pts',(-2.53134978004337,8.95349309713545,12.75));
#6972=CARTESIAN_POINT('Ctrl Pts',(-2.56893767747319,8.99699699918147,-3.75));
#6973=CARTESIAN_POINT('Ctrl Pts',(-2.56893767747319,8.99699699918147,12.75));
#6974=CARTESIAN_POINT('Ctrl Pts',(-2.60721699951879,9.0401474973841,-3.75));
#6975=CARTESIAN_POINT('Ctrl Pts',(-2.60721699951879,9.0401474973841,12.75));
#6976=CARTESIAN_POINT('Ctrl Pts',(-2.64622438896052,9.08292294803309,-3.75));
#6977=CARTESIAN_POINT('Ctrl Pts',(-2.64622438896052,9.08292294803309,12.75));
#6978=CARTESIAN_POINT('Ctrl Pts',(-2.68599232523134,9.12530360007999,-3.75));
#6979=CARTESIAN_POINT('Ctrl Pts',(-2.68599232523134,9.12530360007999,12.75));
#6980=CARTESIAN_POINT('Ctrl Pts',(-2.72652481622916,9.16728115317076,-3.75));
#6981=CARTESIAN_POINT('Ctrl Pts',(-2.72652481622916,9.16728115317076,12.75));
#6982=CARTESIAN_POINT('Ctrl Pts',(-2.76780196452137,9.20885693589776,-3.75));
#6983=CARTESIAN_POINT('Ctrl Pts',(-2.76780196452137,9.20885693589776,12.75));
#6984=CARTESIAN_POINT('Ctrl Pts',(-2.80979051507329,9.2500377269296,-3.75));
#6985=CARTESIAN_POINT('Ctrl Pts',(-2.80979051507329,9.2500377269296,12.75));
#6986=CARTESIAN_POINT('Ctrl Pts',(-2.85245238280019,9.29083237315974,-3.75));
#6987=CARTESIAN_POINT('Ctrl Pts',(-2.85245238280019,9.29083237315974,12.75));
#6988=CARTESIAN_POINT('Ctrl Pts',(-2.89575377593937,9.33124817395869,-3.75));
#6989=CARTESIAN_POINT('Ctrl Pts',(-2.89575377593937,9.33124817395869,12.75));
#6990=CARTESIAN_POINT('Ctrl Pts',(-2.9396747031485,9.3712871143499,-3.75));
#6991=CARTESIAN_POINT('Ctrl Pts',(-2.9396747031485,9.3712871143499,12.75));
#6992=CARTESIAN_POINT('Ctrl Pts',(-2.98420577513995,9.4109471173216,-3.75));
#6993=CARTESIAN_POINT('Ctrl Pts',(-2.98420577513995,9.4109471173216,12.75));
#6994=CARTESIAN_POINT('Ctrl Pts',(-3.029344033256,9.4502236812248,-3.75));
#6995=CARTESIAN_POINT('Ctrl Pts',(-3.029344033256,9.4502236812248,12.75));
#6996=CARTESIAN_POINT('Ctrl Pts',(-3.07508913212203,9.4891113781729,-3.75));
#6997=CARTESIAN_POINT('Ctrl Pts',(-3.07508913212203,9.4891113781729,12.75));
#6998=CARTESIAN_POINT('Ctrl Pts',(-3.12143939300699,9.52760540436562,-3.75));
#6999=CARTESIAN_POINT('Ctrl Pts',(-3.12143939300699,9.52760540436562,12.75));
#7000=CARTESIAN_POINT('Ctrl Pts',(-3.16838785383003,9.56570313257491,-3.75));
#7001=CARTESIAN_POINT('Ctrl Pts',(-3.16838785383003,9.56570313257491,12.75));
#7002=CARTESIAN_POINT('Ctrl Pts',(-3.2159238260067,9.60340349406962,-3.75));
#7003=CARTESIAN_POINT('Ctrl Pts',(-3.2159238260067,9.60340349406962,12.75));
#7004=CARTESIAN_POINT('Ctrl Pts',(-3.26403452382222,9.64070633286081,-3.75));
#7005=CARTESIAN_POINT('Ctrl Pts',(-3.26403452382222,9.64070633286081,12.75));
#7006=CARTESIAN_POINT('Ctrl Pts',(-3.31270665744062,9.67761177523124,-3.75));
#7007=CARTESIAN_POINT('Ctrl Pts',(-3.31270665744062,9.67761177523124,12.75));
#7008=CARTESIAN_POINT('Ctrl Pts',(-3.36192803839197,9.71411959533041,-3.75));
#7009=CARTESIAN_POINT('Ctrl Pts',(-3.36192803839197,9.71411959533041,12.75));
#7010=CARTESIAN_POINT('Ctrl Pts',(-3.41168916880891,9.75022858813702,-3.75));
#7011=CARTESIAN_POINT('Ctrl Pts',(-3.41168916880891,9.75022858813702,12.75));
#7012=CARTESIAN_POINT('Ctrl Pts',(-3.46198252886956,9.78593684022037,-3.75));
#7013=CARTESIAN_POINT('Ctrl Pts',(-3.46198252886956,9.78593684022037,12.75));
#7014=CARTESIAN_POINT('Ctrl Pts',(-3.51280187273295,9.8212419982557,-3.75));
#7015=CARTESIAN_POINT('Ctrl Pts',(-3.51280187273295,9.8212419982557,12.75));
#7016=CARTESIAN_POINT('Ctrl Pts',(-3.56414151726151,9.85614154137781,-3.75));
#7017=CARTESIAN_POINT('Ctrl Pts',(-3.56414151726151,9.85614154137781,12.75));
#7018=CARTESIAN_POINT('Ctrl Pts',(-3.61599563628969,9.89063305253546,-3.75));
#7019=CARTESIAN_POINT('Ctrl Pts',(-3.61599563628969,9.89063305253546,12.75));
#7020=CARTESIAN_POINT('Ctrl Pts',(-3.66835753420625,9.92471449880883,-3.75));
#7021=CARTESIAN_POINT('Ctrl Pts',(-3.66835753420625,9.92471449880883,12.75));
#7022=CARTESIAN_POINT('Ctrl Pts',(-3.72121993173636,9.95838412799173,-3.75));
#7023=CARTESIAN_POINT('Ctrl Pts',(-3.72121993173636,9.95838412799173,12.75));
#7024=CARTESIAN_POINT('Ctrl Pts',(-3.77457526401004,9.99164036147395,-3.75));
#7025=CARTESIAN_POINT('Ctrl Pts',(-3.77457526401004,9.99164036147395,12.75));
#7026=CARTESIAN_POINT('Ctrl Pts',(-3.82841597408715,10.0244816905709,-3.75));
#7027=CARTESIAN_POINT('Ctrl Pts',(-3.82841597408715,10.0244816905709,12.75));
#7028=CARTESIAN_POINT('Ctrl Pts',(-3.88273479532262,10.056906577166,-3.75));
#7029=CARTESIAN_POINT('Ctrl Pts',(-3.88273479532262,10.056906577166,12.75));
#7030=CARTESIAN_POINT('Ctrl Pts',(-3.93752506012706,10.0889133486827,-3.75));
#7031=CARTESIAN_POINT('Ctrl Pts',(-3.93752506012706,10.0889133486827,12.75));
#7032=CARTESIAN_POINT('Ctrl Pts',(-3.99278057289046,10.1205002164952,-3.75));
#7033=CARTESIAN_POINT('Ctrl Pts',(-3.99278057289046,10.1205002164952,12.75));
#7034=CARTESIAN_POINT('Ctrl Pts',(-4.04849544744087,10.1516653064199,-3.75));
#7035=CARTESIAN_POINT('Ctrl Pts',(-4.04849544744087,10.1516653064199,12.75));
#7036=CARTESIAN_POINT('Ctrl Pts',(-4.10466394929486,10.1824066879509,-3.75));
#7037=CARTESIAN_POINT('Ctrl Pts',(-4.10466394929486,10.1824066879509,12.75));
#7038=CARTESIAN_POINT('Ctrl Pts',(-4.16128034451962,10.2127224064663,-3.75));
#7039=CARTESIAN_POINT('Ctrl Pts',(-4.16128034451962,10.2127224064663,12.75));
#7040=CARTESIAN_POINT('Ctrl Pts',(-4.21833871177567,10.2426105188232,-3.75));
#7041=CARTESIAN_POINT('Ctrl Pts',(-4.21833871177567,10.2426105188232,12.75));
#7042=CARTESIAN_POINT('Ctrl Pts',(-4.27583301771353,10.272069116189,-3.75));
#7043=CARTESIAN_POINT('Ctrl Pts',(-4.27583301771353,10.272069116189,12.75));
#7044=CARTESIAN_POINT('Ctrl Pts',(-4.33375724408483,10.3010963438997,-3.75));
#7045=CARTESIAN_POINT('Ctrl Pts',(-4.33375724408483,10.3010963438997,12.75));
#7046=CARTESIAN_POINT('Ctrl Pts',(-4.39210550098945,10.3296904287044,-3.75));
#7047=CARTESIAN_POINT('Ctrl Pts',(-4.39210550098945,10.3296904287044,12.75));
#7048=CARTESIAN_POINT('Ctrl Pts',(-4.45087212698485,10.3578496987941,-3.75));
#7049=CARTESIAN_POINT('Ctrl Pts',(-4.45087212698485,10.3578496987941,12.75));
#7050=CARTESIAN_POINT('Ctrl Pts',(-4.5100518320603,10.3855726289458,-3.75));
#7051=CARTESIAN_POINT('Ctrl Pts',(-4.5100518320603,10.3855726289458,12.75));
#7052=CARTESIAN_POINT('Ctrl Pts',(-4.56963961142454,10.4128577818052,-3.75));
#7053=CARTESIAN_POINT('Ctrl Pts',(-4.56963961142454,10.4128577818052,12.75));
#7054=CARTESIAN_POINT('Ctrl Pts',(-4.62963055491846,10.4397037052484,-3.75));
#7055=CARTESIAN_POINT('Ctrl Pts',(-4.62963055491846,10.4397037052484,12.75));
#7056=CARTESIAN_POINT('Ctrl Pts',(-4.69001967404875,10.4661088391609,-3.75));
#7057=CARTESIAN_POINT('Ctrl Pts',(-4.69001967404875,10.4661088391609,12.75));
#7058=CARTESIAN_POINT('Ctrl Pts',(-4.7508017470924,10.4920714379865,-3.75));
#7059=CARTESIAN_POINT('Ctrl Pts',(-4.7508017470924,10.4920714379865,12.75));
#7060=CARTESIAN_POINT('Ctrl Pts',(-4.81197108362035,10.5175894490106,-3.75));
#7061=CARTESIAN_POINT('Ctrl Pts',(-4.81197108362035,10.5175894490106,12.75));
#7062=CARTESIAN_POINT('Ctrl Pts',(-4.87352158939686,10.5426605691059,-3.75));
#7063=CARTESIAN_POINT('Ctrl Pts',(-4.87352158939686,10.5426605691059,12.75));
#7064=CARTESIAN_POINT('Ctrl Pts',(-4.93544714999767,10.5672824880187,-3.75));
#7065=CARTESIAN_POINT('Ctrl Pts',(-4.93544714999767,10.5672824880187,12.75));
#7066=CARTESIAN_POINT('Ctrl Pts',(-4.99774193408264,10.5914530920551,-3.75));
#7067=CARTESIAN_POINT('Ctrl Pts',(-4.99774193408264,10.5914530920551,12.75));
#7068=CARTESIAN_POINT('Ctrl Pts',(-5.06040071098369,10.6151706715837,-3.75));
#7069=CARTESIAN_POINT('Ctrl Pts',(-5.06040071098369,10.6151706715837,12.75));
#7070=CARTESIAN_POINT('Ctrl Pts',(-5.12341919820983,10.638434168447,-3.75));
#7071=CARTESIAN_POINT('Ctrl Pts',(-5.12341919820983,10.638434168447,12.75));
#7072=CARTESIAN_POINT('Ctrl Pts',(-5.18679427410258,10.661243291145,-3.75));
#7073=CARTESIAN_POINT('Ctrl Pts',(-5.18679427410258,10.661243291145,12.75));
#7074=CARTESIAN_POINT('Ctrl Pts',(-5.25052377191006,10.6835982206291,-3.75));
#7075=CARTESIAN_POINT('Ctrl Pts',(-5.25052377191006,10.6835982206291,12.75));
#7076=CARTESIAN_POINT('Ctrl Pts',(-5.30178983253176,10.7011191580639,-3.75));
#7077=CARTESIAN_POINT('Ctrl Pts',(-5.30178983253176,10.7011191580639,12.75));
#7078=CARTESIAN_POINT('Ctrl Pts',(-5.34039795525198,10.714055870666,-3.75));
#7079=CARTESIAN_POINT('Ctrl Pts',(-5.34039795525198,10.714055870666,12.75));
#7080=CARTESIAN_POINT('Ctrl Pts',(-5.3662071591827,10.7225897134991,-3.75));
#7081=CARTESIAN_POINT('Ctrl Pts',(-5.3662071591827,10.7225897134991,12.75));
#7082=CARTESIAN_POINT('Ctrl Pts',(-5.37912937500617,10.726833976852,-3.75));
#7083=CARTESIAN_POINT('Ctrl Pts',(-5.37912937500617,10.726833976852,12.75));
#7084=CARTESIAN_POINT('Ctrl Pts',(-2.066899701215,8.20077591276801,-1.));
#7085=CARTESIAN_POINT('Ctrl Pts',(-2.06955313972063,8.21130388109186,-1.));
#7086=CARTESIAN_POINT('Ctrl Pts',(-2.07530073900944,8.23220544002367,-1.));
#7087=CARTESIAN_POINT('Ctrl Pts',(-2.08524426770062,8.26309465918435,-1.));
#7088=CARTESIAN_POINT('Ctrl Pts',(-2.10101049300138,8.3034037182712,-1.));
#7089=CARTESIAN_POINT('Ctrl Pts',(-2.12411443763999,8.35261410600662,-1.));
#7090=CARTESIAN_POINT('Ctrl Pts',(-2.1496314108288,8.40100363162428,-1.));
#7091=CARTESIAN_POINT('Ctrl Pts',(-2.17660700812681,8.44891314968814,-1.));
#7092=CARTESIAN_POINT('Ctrl Pts',(-2.20438215159743,8.49657041043196,-1.));
#7093=CARTESIAN_POINT('Ctrl Pts',(-2.23274297834755,8.54403497990068,-1.));
#7094=CARTESIAN_POINT('Ctrl Pts',(-2.26174990860571,8.59126351952004,-1.));
#7095=CARTESIAN_POINT('Ctrl Pts',(-2.29162050823335,8.63815494571075,-1.));
#7096=CARTESIAN_POINT('Ctrl Pts',(-2.32260171926006,8.68459942442029,-1.));
#7097=CARTESIAN_POINT('Ctrl Pts',(-2.35482147675117,8.73053548487858,-1.));
#7098=CARTESIAN_POINT('Ctrl Pts',(-2.38824857383288,8.77596511266658,-1.));
#7099=CARTESIAN_POINT('Ctrl Pts',(-2.4227653824809,8.82092512134556,-1.));
#7100=CARTESIAN_POINT('Ctrl Pts',(-2.45821141167118,8.86546980570045,-1.));
#7101=CARTESIAN_POINT('Ctrl Pts',(-2.4944346415182,8.90965062344541,-1.));
#7102=CARTESIAN_POINT('Ctrl Pts',(-2.53134978004337,8.95349309713545,-1.));
#7103=CARTESIAN_POINT('Ctrl Pts',(-2.56893767747319,8.99699699918147,-1.));
#7104=CARTESIAN_POINT('Ctrl Pts',(-2.60721699951879,9.0401474973841,-1.));
#7105=CARTESIAN_POINT('Ctrl Pts',(-2.64622438896052,9.08292294803309,-1.));
#7106=CARTESIAN_POINT('Ctrl Pts',(-2.68599232523134,9.12530360007999,-1.));
#7107=CARTESIAN_POINT('Ctrl Pts',(-2.72652481622916,9.16728115317076,-1.));
#7108=CARTESIAN_POINT('Ctrl Pts',(-2.76780196452137,9.20885693589776,-1.));
#7109=CARTESIAN_POINT('Ctrl Pts',(-2.80979051507329,9.2500377269296,-1.));
#7110=CARTESIAN_POINT('Ctrl Pts',(-2.85245238280019,9.29083237315974,-1.));
#7111=CARTESIAN_POINT('Ctrl Pts',(-2.89575377593937,9.33124817395869,-1.));
#7112=CARTESIAN_POINT('Ctrl Pts',(-2.9396747031485,9.3712871143499,-1.));
#7113=CARTESIAN_POINT('Ctrl Pts',(-2.98420577513995,9.4109471173216,-1.));
#7114=CARTESIAN_POINT('Ctrl Pts',(-3.029344033256,9.4502236812248,-1.));
#7115=CARTESIAN_POINT('Ctrl Pts',(-3.07508913212203,9.4891113781729,-1.));
#7116=CARTESIAN_POINT('Ctrl Pts',(-3.12143939300699,9.52760540436562,-1.));
#7117=CARTESIAN_POINT('Ctrl Pts',(-3.16838785383003,9.56570313257491,-1.));
#7118=CARTESIAN_POINT('Ctrl Pts',(-3.2159238260067,9.60340349406962,-1.));
#7119=CARTESIAN_POINT('Ctrl Pts',(-3.26403452382222,9.64070633286081,-1.));
#7120=CARTESIAN_POINT('Ctrl Pts',(-3.31270665744062,9.67761177523124,-1.));
#7121=CARTESIAN_POINT('Ctrl Pts',(-3.36192803839197,9.71411959533041,-1.));
#7122=CARTESIAN_POINT('Ctrl Pts',(-3.41168916880891,9.75022858813702,-1.));
#7123=CARTESIAN_POINT('Ctrl Pts',(-3.46198252886956,9.78593684022037,-1.));
#7124=CARTESIAN_POINT('Ctrl Pts',(-3.51280187273295,9.8212419982557,-1.));
#7125=CARTESIAN_POINT('Ctrl Pts',(-3.56414151726151,9.85614154137781,-1.));
#7126=CARTESIAN_POINT('Ctrl Pts',(-3.61599563628969,9.89063305253546,-1.));
#7127=CARTESIAN_POINT('Ctrl Pts',(-3.66835753420625,9.92471449880883,-1.));
#7128=CARTESIAN_POINT('Ctrl Pts',(-3.72121993173636,9.95838412799173,-1.));
#7129=CARTESIAN_POINT('Ctrl Pts',(-3.77457526401004,9.99164036147395,-1.));
#7130=CARTESIAN_POINT('Ctrl Pts',(-3.82841597408715,10.0244816905709,-1.));
#7131=CARTESIAN_POINT('Ctrl Pts',(-3.88273479532262,10.056906577166,-1.));
#7132=CARTESIAN_POINT('Ctrl Pts',(-3.93752506012706,10.0889133486827,-1.));
#7133=CARTESIAN_POINT('Ctrl Pts',(-3.99278057289046,10.1205002164952,-1.));
#7134=CARTESIAN_POINT('Ctrl Pts',(-4.04849544744087,10.1516653064199,-1.));
#7135=CARTESIAN_POINT('Ctrl Pts',(-4.10466394929486,10.1824066879509,-1.));
#7136=CARTESIAN_POINT('Ctrl Pts',(-4.16128034451962,10.2127224064663,-1.));
#7137=CARTESIAN_POINT('Ctrl Pts',(-4.21833871177567,10.2426105188232,-1.));
#7138=CARTESIAN_POINT('Ctrl Pts',(-4.27583301771353,10.272069116189,-1.));
#7139=CARTESIAN_POINT('Ctrl Pts',(-4.33375724408483,10.3010963438997,-1.));
#7140=CARTESIAN_POINT('Ctrl Pts',(-4.39210550098945,10.3296904287044,-1.));
#7141=CARTESIAN_POINT('Ctrl Pts',(-4.45087212698485,10.3578496987941,-1.));
#7142=CARTESIAN_POINT('Ctrl Pts',(-4.5100518320603,10.3855726289458,-1.));
#7143=CARTESIAN_POINT('Ctrl Pts',(-4.56963961142454,10.4128577818052,-1.));
#7144=CARTESIAN_POINT('Ctrl Pts',(-4.62963055491846,10.4397037052484,-1.));
#7145=CARTESIAN_POINT('Ctrl Pts',(-4.69001967404875,10.4661088391609,-1.));
#7146=CARTESIAN_POINT('Ctrl Pts',(-4.7508017470924,10.4920714379865,-1.));
#7147=CARTESIAN_POINT('Ctrl Pts',(-4.81197108362035,10.5175894490106,-1.));
#7148=CARTESIAN_POINT('Ctrl Pts',(-4.87352158939686,10.5426605691059,-1.));
#7149=CARTESIAN_POINT('Ctrl Pts',(-4.93544714999767,10.5672824880187,-1.));
#7150=CARTESIAN_POINT('Ctrl Pts',(-4.99774193408264,10.5914530920551,-1.));
#7151=CARTESIAN_POINT('Ctrl Pts',(-5.06040071098369,10.6151706715837,-1.));
#7152=CARTESIAN_POINT('Ctrl Pts',(-5.12341919820983,10.638434168447,-1.));
#7153=CARTESIAN_POINT('Ctrl Pts',(-5.18679427410258,10.661243291145,-1.));
#7154=CARTESIAN_POINT('Ctrl Pts',(-5.25052377191006,10.6835982206291,-1.));
#7155=CARTESIAN_POINT('Ctrl Pts',(-5.30178983253176,10.7011191580639,-1.));
#7156=CARTESIAN_POINT('Ctrl Pts',(-5.34039795525198,10.714055870666,-1.));
#7157=CARTESIAN_POINT('Ctrl Pts',(-5.3662071591827,10.7225897134991,-1.));
#7158=CARTESIAN_POINT('Ctrl Pts',(-5.37912937500617,10.726833976852,-1.));
#7159=CARTESIAN_POINT('Ctrl Pts',(-2.066899701215,8.20077591276801,6.));
#7160=CARTESIAN_POINT('Ctrl Pts',(-2.06955313972063,8.21130388109186,6.));
#7161=CARTESIAN_POINT('Ctrl Pts',(-2.07530073900944,8.23220544002367,6.));
#7162=CARTESIAN_POINT('Ctrl Pts',(-2.08524426770062,8.26309465918435,6.));
#7163=CARTESIAN_POINT('Ctrl Pts',(-2.10101049300138,8.3034037182712,6.));
#7164=CARTESIAN_POINT('Ctrl Pts',(-2.12411443763999,8.35261410600662,6.));
#7165=CARTESIAN_POINT('Ctrl Pts',(-2.1496314108288,8.40100363162428,6.));
#7166=CARTESIAN_POINT('Ctrl Pts',(-2.17660700812681,8.44891314968814,6.));
#7167=CARTESIAN_POINT('Ctrl Pts',(-2.20438215159743,8.49657041043196,6.));
#7168=CARTESIAN_POINT('Ctrl Pts',(-2.23274297834755,8.54403497990068,6.));
#7169=CARTESIAN_POINT('Ctrl Pts',(-2.26174990860571,8.59126351952004,6.));
#7170=CARTESIAN_POINT('Ctrl Pts',(-2.29162050823335,8.63815494571075,6.));
#7171=CARTESIAN_POINT('Ctrl Pts',(-2.32260171926006,8.68459942442029,6.));
#7172=CARTESIAN_POINT('Ctrl Pts',(-2.35482147675117,8.73053548487858,6.));
#7173=CARTESIAN_POINT('Ctrl Pts',(-2.38824857383288,8.77596511266658,6.));
#7174=CARTESIAN_POINT('Ctrl Pts',(-2.4227653824809,8.82092512134556,6.));
#7175=CARTESIAN_POINT('Ctrl Pts',(-2.45821141167118,8.86546980570045,6.));
#7176=CARTESIAN_POINT('Ctrl Pts',(-2.4944346415182,8.90965062344541,6.));
#7177=CARTESIAN_POINT('Ctrl Pts',(-2.53134978004337,8.95349309713545,6.));
#7178=CARTESIAN_POINT('Ctrl Pts',(-2.56893767747319,8.99699699918147,6.));
#7179=CARTESIAN_POINT('Ctrl Pts',(-2.60721699951879,9.0401474973841,6.));
#7180=CARTESIAN_POINT('Ctrl Pts',(-2.64622438896052,9.08292294803309,6.));
#7181=CARTESIAN_POINT('Ctrl Pts',(-2.68599232523134,9.12530360007999,6.));
#7182=CARTESIAN_POINT('Ctrl Pts',(-2.72652481622916,9.16728115317076,6.));
#7183=CARTESIAN_POINT('Ctrl Pts',(-2.76780196452137,9.20885693589776,6.));
#7184=CARTESIAN_POINT('Ctrl Pts',(-2.80979051507329,9.2500377269296,6.));
#7185=CARTESIAN_POINT('Ctrl Pts',(-2.85245238280019,9.29083237315974,6.));
#7186=CARTESIAN_POINT('Ctrl Pts',(-2.89575377593937,9.33124817395869,6.));
#7187=CARTESIAN_POINT('Ctrl Pts',(-2.9396747031485,9.3712871143499,6.));
#7188=CARTESIAN_POINT('Ctrl Pts',(-2.98420577513995,9.4109471173216,6.));
#7189=CARTESIAN_POINT('Ctrl Pts',(-3.029344033256,9.4502236812248,6.));
#7190=CARTESIAN_POINT('Ctrl Pts',(-3.07508913212203,9.4891113781729,6.));
#7191=CARTESIAN_POINT('Ctrl Pts',(-3.12143939300699,9.52760540436562,6.));
#7192=CARTESIAN_POINT('Ctrl Pts',(-3.16838785383003,9.56570313257491,6.));
#7193=CARTESIAN_POINT('Ctrl Pts',(-3.2159238260067,9.60340349406962,6.));
#7194=CARTESIAN_POINT('Ctrl Pts',(-3.26403452382222,9.64070633286081,6.));
#7195=CARTESIAN_POINT('Ctrl Pts',(-3.31270665744062,9.67761177523124,6.));
#7196=CARTESIAN_POINT('Ctrl Pts',(-3.36192803839197,9.71411959533041,6.));
#7197=CARTESIAN_POINT('Ctrl Pts',(-3.41168916880891,9.75022858813702,6.));
#7198=CARTESIAN_POINT('Ctrl Pts',(-3.46198252886956,9.78593684022037,6.));
#7199=CARTESIAN_POINT('Ctrl Pts',(-3.51280187273295,9.8212419982557,6.));
#7200=CARTESIAN_POINT('Ctrl Pts',(-3.56414151726151,9.85614154137781,6.));
#7201=CARTESIAN_POINT('Ctrl Pts',(-3.61599563628969,9.89063305253546,6.));
#7202=CARTESIAN_POINT('Ctrl Pts',(-3.66835753420625,9.92471449880883,6.));
#7203=CARTESIAN_POINT('Ctrl Pts',(-3.72121993173636,9.95838412799173,6.));
#7204=CARTESIAN_POINT('Ctrl Pts',(-3.77457526401004,9.99164036147395,6.));
#7205=CARTESIAN_POINT('Ctrl Pts',(-3.82841597408715,10.0244816905709,6.));
#7206=CARTESIAN_POINT('Ctrl Pts',(-3.88273479532262,10.056906577166,6.));
#7207=CARTESIAN_POINT('Ctrl Pts',(-3.93752506012706,10.0889133486827,6.));
#7208=CARTESIAN_POINT('Ctrl Pts',(-3.99278057289046,10.1205002164952,6.));
#7209=CARTESIAN_POINT('Ctrl Pts',(-4.04849544744087,10.1516653064199,6.));
#7210=CARTESIAN_POINT('Ctrl Pts',(-4.10466394929486,10.1824066879509,6.));
#7211=CARTESIAN_POINT('Ctrl Pts',(-4.16128034451962,10.2127224064663,6.));
#7212=CARTESIAN_POINT('Ctrl Pts',(-4.21833871177567,10.2426105188232,6.));
#7213=CARTESIAN_POINT('Ctrl Pts',(-4.27583301771353,10.272069116189,6.));
#7214=CARTESIAN_POINT('Ctrl Pts',(-4.33375724408483,10.3010963438997,6.));
#7215=CARTESIAN_POINT('Ctrl Pts',(-4.39210550098945,10.3296904287044,6.));
#7216=CARTESIAN_POINT('Ctrl Pts',(-4.45087212698485,10.3578496987941,6.));
#7217=CARTESIAN_POINT('Ctrl Pts',(-4.5100518320603,10.3855726289458,6.));
#7218=CARTESIAN_POINT('Ctrl Pts',(-4.56963961142454,10.4128577818052,6.));
#7219=CARTESIAN_POINT('Ctrl Pts',(-4.62963055491846,10.4397037052484,6.));
#7220=CARTESIAN_POINT('Ctrl Pts',(-4.69001967404875,10.4661088391609,6.));
#7221=CARTESIAN_POINT('Ctrl Pts',(-4.7508017470924,10.4920714379865,6.));
#7222=CARTESIAN_POINT('Ctrl Pts',(-4.81197108362035,10.5175894490106,6.));
#7223=CARTESIAN_POINT('Ctrl Pts',(-4.87352158939686,10.5426605691059,6.));
#7224=CARTESIAN_POINT('Ctrl Pts',(-4.93544714999767,10.5672824880187,6.));
#7225=CARTESIAN_POINT('Ctrl Pts',(-4.99774193408264,10.5914530920551,6.));
#7226=CARTESIAN_POINT('Ctrl Pts',(-5.06040071098369,10.6151706715837,6.));
#7227=CARTESIAN_POINT('Ctrl Pts',(-5.12341919820983,10.638434168447,6.));
#7228=CARTESIAN_POINT('Ctrl Pts',(-5.18679427410258,10.661243291145,6.));
#7229=CARTESIAN_POINT('Ctrl Pts',(-5.25052377191006,10.6835982206291,6.));
#7230=CARTESIAN_POINT('Ctrl Pts',(-5.30178983253176,10.7011191580639,6.));
#7231=CARTESIAN_POINT('Ctrl Pts',(-5.34039795525198,10.714055870666,6.));
#7232=CARTESIAN_POINT('Ctrl Pts',(-5.3662071591827,10.7225897134991,6.));
#7233=CARTESIAN_POINT('Ctrl Pts',(-5.37912937500617,10.726833976852,6.));
#7234=CARTESIAN_POINT('Ctrl Pts',(5.37912937500617,10.726833976852,-3.75));
#7235=CARTESIAN_POINT('Ctrl Pts',(5.37912937500617,10.726833976852,12.75));
#7236=CARTESIAN_POINT('Ctrl Pts',(5.36620715918271,10.7225897134991,-3.75));
#7237=CARTESIAN_POINT('Ctrl Pts',(5.36620715918271,10.7225897134991,12.75));
#7238=CARTESIAN_POINT('Ctrl Pts',(5.34039795525198,10.714055870666,-3.75));
#7239=CARTESIAN_POINT('Ctrl Pts',(5.34039795525198,10.714055870666,12.75));
#7240=CARTESIAN_POINT('Ctrl Pts',(5.30178983253176,10.7011191580639,-3.75));
#7241=CARTESIAN_POINT('Ctrl Pts',(5.30178983253176,10.7011191580639,12.75));
#7242=CARTESIAN_POINT('Ctrl Pts',(5.25052377191006,10.6835982206291,-3.75));
#7243=CARTESIAN_POINT('Ctrl Pts',(5.25052377191006,10.6835982206291,12.75));
#7244=CARTESIAN_POINT('Ctrl Pts',(5.18679427410258,10.661243291145,-3.75));
#7245=CARTESIAN_POINT('Ctrl Pts',(5.18679427410258,10.661243291145,12.75));
#7246=CARTESIAN_POINT('Ctrl Pts',(5.12341919820984,10.638434168447,-3.75));
#7247=CARTESIAN_POINT('Ctrl Pts',(5.12341919820984,10.638434168447,12.75));
#7248=CARTESIAN_POINT('Ctrl Pts',(5.06040071098369,10.6151706715837,-3.75));
#7249=CARTESIAN_POINT('Ctrl Pts',(5.06040071098369,10.6151706715837,12.75));
#7250=CARTESIAN_POINT('Ctrl Pts',(4.99774193408264,10.5914530920551,-3.75));
#7251=CARTESIAN_POINT('Ctrl Pts',(4.99774193408264,10.5914530920551,12.75));
#7252=CARTESIAN_POINT('Ctrl Pts',(4.93544714999767,10.5672824880187,-3.75));
#7253=CARTESIAN_POINT('Ctrl Pts',(4.93544714999767,10.5672824880187,12.75));
#7254=CARTESIAN_POINT('Ctrl Pts',(4.87352158939686,10.5426605691059,-3.75));
#7255=CARTESIAN_POINT('Ctrl Pts',(4.87352158939686,10.5426605691059,12.75));
#7256=CARTESIAN_POINT('Ctrl Pts',(4.81197108362035,10.5175894490106,-3.75));
#7257=CARTESIAN_POINT('Ctrl Pts',(4.81197108362035,10.5175894490106,12.75));
#7258=CARTESIAN_POINT('Ctrl Pts',(4.7508017470924,10.4920714379865,-3.75));
#7259=CARTESIAN_POINT('Ctrl Pts',(4.7508017470924,10.4920714379865,12.75));
#7260=CARTESIAN_POINT('Ctrl Pts',(4.69001967404875,10.4661088391609,-3.75));
#7261=CARTESIAN_POINT('Ctrl Pts',(4.69001967404875,10.4661088391609,12.75));
#7262=CARTESIAN_POINT('Ctrl Pts',(4.62963055491846,10.4397037052484,-3.75));
#7263=CARTESIAN_POINT('Ctrl Pts',(4.62963055491846,10.4397037052484,12.75));
#7264=CARTESIAN_POINT('Ctrl Pts',(4.56963961142454,10.4128577818052,-3.75));
#7265=CARTESIAN_POINT('Ctrl Pts',(4.56963961142454,10.4128577818052,12.75));
#7266=CARTESIAN_POINT('Ctrl Pts',(4.5100518320603,10.3855726289458,-3.75));
#7267=CARTESIAN_POINT('Ctrl Pts',(4.5100518320603,10.3855726289458,12.75));
#7268=CARTESIAN_POINT('Ctrl Pts',(4.45087212698485,10.3578496987941,-3.75));
#7269=CARTESIAN_POINT('Ctrl Pts',(4.45087212698485,10.3578496987941,12.75));
#7270=CARTESIAN_POINT('Ctrl Pts',(4.39210550098945,10.3296904287044,-3.75));
#7271=CARTESIAN_POINT('Ctrl Pts',(4.39210550098945,10.3296904287044,12.75));
#7272=CARTESIAN_POINT('Ctrl Pts',(4.33375724408484,10.3010963438997,-3.75));
#7273=CARTESIAN_POINT('Ctrl Pts',(4.33375724408484,10.3010963438997,12.75));
#7274=CARTESIAN_POINT('Ctrl Pts',(4.27583301771353,10.272069116189,-3.75));
#7275=CARTESIAN_POINT('Ctrl Pts',(4.27583301771353,10.272069116189,12.75));
#7276=CARTESIAN_POINT('Ctrl Pts',(4.21833871177567,10.2426105188232,-3.75));
#7277=CARTESIAN_POINT('Ctrl Pts',(4.21833871177567,10.2426105188232,12.75));
#7278=CARTESIAN_POINT('Ctrl Pts',(4.16128034451962,10.2127224064663,-3.75));
#7279=CARTESIAN_POINT('Ctrl Pts',(4.16128034451962,10.2127224064663,12.75));
#7280=CARTESIAN_POINT('Ctrl Pts',(4.10466394929486,10.1824066879509,-3.75));
#7281=CARTESIAN_POINT('Ctrl Pts',(4.10466394929486,10.1824066879509,12.75));
#7282=CARTESIAN_POINT('Ctrl Pts',(4.04849544744087,10.1516653064199,-3.75));
#7283=CARTESIAN_POINT('Ctrl Pts',(4.04849544744087,10.1516653064199,12.75));
#7284=CARTESIAN_POINT('Ctrl Pts',(3.99278057289046,10.1205002164952,-3.75));
#7285=CARTESIAN_POINT('Ctrl Pts',(3.99278057289046,10.1205002164952,12.75));
#7286=CARTESIAN_POINT('Ctrl Pts',(3.93752506012707,10.0889133486827,-3.75));
#7287=CARTESIAN_POINT('Ctrl Pts',(3.93752506012707,10.0889133486827,12.75));
#7288=CARTESIAN_POINT('Ctrl Pts',(3.88273479532263,10.056906577166,-3.75));
#7289=CARTESIAN_POINT('Ctrl Pts',(3.88273479532263,10.056906577166,12.75));
#7290=CARTESIAN_POINT('Ctrl Pts',(3.82841597408715,10.0244816905709,-3.75));
#7291=CARTESIAN_POINT('Ctrl Pts',(3.82841597408715,10.0244816905709,12.75));
#7292=CARTESIAN_POINT('Ctrl Pts',(3.77457526401004,9.99164036147395,-3.75));
#7293=CARTESIAN_POINT('Ctrl Pts',(3.77457526401004,9.99164036147395,12.75));
#7294=CARTESIAN_POINT('Ctrl Pts',(3.72121993173636,9.95838412799172,-3.75));
#7295=CARTESIAN_POINT('Ctrl Pts',(3.72121993173636,9.95838412799172,12.75));
#7296=CARTESIAN_POINT('Ctrl Pts',(3.66835753420625,9.92471449880883,-3.75));
#7297=CARTESIAN_POINT('Ctrl Pts',(3.66835753420625,9.92471449880883,12.75));
#7298=CARTESIAN_POINT('Ctrl Pts',(3.61599563628969,9.89063305253546,-3.75));
#7299=CARTESIAN_POINT('Ctrl Pts',(3.61599563628969,9.89063305253546,12.75));
#7300=CARTESIAN_POINT('Ctrl Pts',(3.56414151726151,9.85614154137781,-3.75));
#7301=CARTESIAN_POINT('Ctrl Pts',(3.56414151726151,9.85614154137781,12.75));
#7302=CARTESIAN_POINT('Ctrl Pts',(3.51280187273295,9.8212419982557,-3.75));
#7303=CARTESIAN_POINT('Ctrl Pts',(3.51280187273295,9.8212419982557,12.75));
#7304=CARTESIAN_POINT('Ctrl Pts',(3.46198252886957,9.78593684022037,-3.75));
#7305=CARTESIAN_POINT('Ctrl Pts',(3.46198252886957,9.78593684022037,12.75));
#7306=CARTESIAN_POINT('Ctrl Pts',(3.41168916880891,9.75022858813702,-3.75));
#7307=CARTESIAN_POINT('Ctrl Pts',(3.41168916880891,9.75022858813702,12.75));
#7308=CARTESIAN_POINT('Ctrl Pts',(3.36192803839197,9.7141195953304,-3.75));
#7309=CARTESIAN_POINT('Ctrl Pts',(3.36192803839197,9.7141195953304,12.75));
#7310=CARTESIAN_POINT('Ctrl Pts',(3.31270665744062,9.67761177523123,-3.75));
#7311=CARTESIAN_POINT('Ctrl Pts',(3.31270665744062,9.67761177523123,12.75));
#7312=CARTESIAN_POINT('Ctrl Pts',(3.26403452382222,9.64070633286081,-3.75));
#7313=CARTESIAN_POINT('Ctrl Pts',(3.26403452382222,9.64070633286081,12.75));
#7314=CARTESIAN_POINT('Ctrl Pts',(3.2159238260067,9.60340349406962,-3.75));
#7315=CARTESIAN_POINT('Ctrl Pts',(3.2159238260067,9.60340349406962,12.75));
#7316=CARTESIAN_POINT('Ctrl Pts',(3.16838785383004,9.56570313257491,-3.75));
#7317=CARTESIAN_POINT('Ctrl Pts',(3.16838785383004,9.56570313257491,12.75));
#7318=CARTESIAN_POINT('Ctrl Pts',(3.12143939300699,9.52760540436562,-3.75));
#7319=CARTESIAN_POINT('Ctrl Pts',(3.12143939300699,9.52760540436562,12.75));
#7320=CARTESIAN_POINT('Ctrl Pts',(3.07508913212204,9.4891113781729,-3.75));
#7321=CARTESIAN_POINT('Ctrl Pts',(3.07508913212204,9.4891113781729,12.75));
#7322=CARTESIAN_POINT('Ctrl Pts',(3.02934403325601,9.4502236812248,-3.75));
#7323=CARTESIAN_POINT('Ctrl Pts',(3.02934403325601,9.4502236812248,12.75));
#7324=CARTESIAN_POINT('Ctrl Pts',(2.98420577513996,9.4109471173216,-3.75));
#7325=CARTESIAN_POINT('Ctrl Pts',(2.98420577513996,9.4109471173216,12.75));
#7326=CARTESIAN_POINT('Ctrl Pts',(2.9396747031485,9.3712871143499,-3.75));
#7327=CARTESIAN_POINT('Ctrl Pts',(2.9396747031485,9.3712871143499,12.75));
#7328=CARTESIAN_POINT('Ctrl Pts',(2.89575377593938,9.33124817395869,-3.75));
#7329=CARTESIAN_POINT('Ctrl Pts',(2.89575377593938,9.33124817395869,12.75));
#7330=CARTESIAN_POINT('Ctrl Pts',(2.8524523828002,9.29083237315974,-3.75));
#7331=CARTESIAN_POINT('Ctrl Pts',(2.8524523828002,9.29083237315974,12.75));
#7332=CARTESIAN_POINT('Ctrl Pts',(2.8097905150733,9.2500377269296,-3.75));
#7333=CARTESIAN_POINT('Ctrl Pts',(2.8097905150733,9.2500377269296,12.75));
#7334=CARTESIAN_POINT('Ctrl Pts',(2.76780196452137,9.20885693589776,-3.75));
#7335=CARTESIAN_POINT('Ctrl Pts',(2.76780196452137,9.20885693589776,12.75));
#7336=CARTESIAN_POINT('Ctrl Pts',(2.72652481622916,9.16728115317076,-3.75));
#7337=CARTESIAN_POINT('Ctrl Pts',(2.72652481622916,9.16728115317076,12.75));
#7338=CARTESIAN_POINT('Ctrl Pts',(2.68599232523134,9.12530360007999,-3.75));
#7339=CARTESIAN_POINT('Ctrl Pts',(2.68599232523134,9.12530360007999,12.75));
#7340=CARTESIAN_POINT('Ctrl Pts',(2.64622438896052,9.08292294803309,-3.75));
#7341=CARTESIAN_POINT('Ctrl Pts',(2.64622438896052,9.08292294803309,12.75));
#7342=CARTESIAN_POINT('Ctrl Pts',(2.60721699951879,9.0401474973841,-3.75));
#7343=CARTESIAN_POINT('Ctrl Pts',(2.60721699951879,9.0401474973841,12.75));
#7344=CARTESIAN_POINT('Ctrl Pts',(2.56893767747319,8.99699699918147,-3.75));
#7345=CARTESIAN_POINT('Ctrl Pts',(2.56893767747319,8.99699699918147,12.75));
#7346=CARTESIAN_POINT('Ctrl Pts',(2.53134978004338,8.95349309713545,-3.75));
#7347=CARTESIAN_POINT('Ctrl Pts',(2.53134978004338,8.95349309713545,12.75));
#7348=CARTESIAN_POINT('Ctrl Pts',(2.4944346415182,8.90965062344541,-3.75));
#7349=CARTESIAN_POINT('Ctrl Pts',(2.4944346415182,8.90965062344541,12.75));
#7350=CARTESIAN_POINT('Ctrl Pts',(2.45821141167119,8.86546980570045,-3.75));
#7351=CARTESIAN_POINT('Ctrl Pts',(2.45821141167119,8.86546980570045,12.75));
#7352=CARTESIAN_POINT('Ctrl Pts',(2.42276538248091,8.82092512134556,-3.75));
#7353=CARTESIAN_POINT('Ctrl Pts',(2.42276538248091,8.82092512134556,12.75));
#7354=CARTESIAN_POINT('Ctrl Pts',(2.38824857383288,8.77596511266658,-3.75));
#7355=CARTESIAN_POINT('Ctrl Pts',(2.38824857383288,8.77596511266658,12.75));
#7356=CARTESIAN_POINT('Ctrl Pts',(2.35482147675118,8.73053548487858,-3.75));
#7357=CARTESIAN_POINT('Ctrl Pts',(2.35482147675118,8.73053548487858,12.75));
#7358=CARTESIAN_POINT('Ctrl Pts',(2.32260171926006,8.68459942442028,-3.75));
#7359=CARTESIAN_POINT('Ctrl Pts',(2.32260171926006,8.68459942442028,12.75));
#7360=CARTESIAN_POINT('Ctrl Pts',(2.29162050823336,8.63815494571075,-3.75));
#7361=CARTESIAN_POINT('Ctrl Pts',(2.29162050823336,8.63815494571075,12.75));
#7362=CARTESIAN_POINT('Ctrl Pts',(2.26174990860571,8.59126351952004,-3.75));
#7363=CARTESIAN_POINT('Ctrl Pts',(2.26174990860571,8.59126351952004,12.75));
#7364=CARTESIAN_POINT('Ctrl Pts',(2.23274297834755,8.54403497990068,-3.75));
#7365=CARTESIAN_POINT('Ctrl Pts',(2.23274297834755,8.54403497990068,12.75));
#7366=CARTESIAN_POINT('Ctrl Pts',(2.20438215159743,8.49657041043195,-3.75));
#7367=CARTESIAN_POINT('Ctrl Pts',(2.20438215159743,8.49657041043195,12.75));
#7368=CARTESIAN_POINT('Ctrl Pts',(2.17660700812682,8.44891314968814,-3.75));
#7369=CARTESIAN_POINT('Ctrl Pts',(2.17660700812682,8.44891314968814,12.75));
#7370=CARTESIAN_POINT('Ctrl Pts',(2.1496314108288,8.40100363162428,-3.75));
#7371=CARTESIAN_POINT('Ctrl Pts',(2.1496314108288,8.40100363162428,12.75));
#7372=CARTESIAN_POINT('Ctrl Pts',(2.12411443763999,8.35261410600662,-3.75));
#7373=CARTESIAN_POINT('Ctrl Pts',(2.12411443763999,8.35261410600662,12.75));
#7374=CARTESIAN_POINT('Ctrl Pts',(2.10101049300138,8.3034037182712,-3.75));
#7375=CARTESIAN_POINT('Ctrl Pts',(2.10101049300138,8.3034037182712,12.75));
#7376=CARTESIAN_POINT('Ctrl Pts',(2.08524426770063,8.26309465918435,-3.75));
#7377=CARTESIAN_POINT('Ctrl Pts',(2.08524426770063,8.26309465918435,12.75));
#7378=CARTESIAN_POINT('Ctrl Pts',(2.07530073900944,8.23220544002367,-3.75));
#7379=CARTESIAN_POINT('Ctrl Pts',(2.07530073900944,8.23220544002367,12.75));
#7380=CARTESIAN_POINT('Ctrl Pts',(2.06955313972063,8.21130388109186,-3.75));
#7381=CARTESIAN_POINT('Ctrl Pts',(2.06955313972063,8.21130388109186,12.75));
#7382=CARTESIAN_POINT('Ctrl Pts',(2.066899701215,8.20077591276801,-3.75));
#7383=CARTESIAN_POINT('Ctrl Pts',(2.066899701215,8.20077591276801,12.75));
#7384=CARTESIAN_POINT('',(5.3791293750062,10.7268339768519,-1.));
#7385=CARTESIAN_POINT('Ctrl Pts',(5.37912937500617,10.726833976852,-1.));
#7386=CARTESIAN_POINT('Ctrl Pts',(5.36620715918271,10.7225897134991,-1.));
#7387=CARTESIAN_POINT('Ctrl Pts',(5.34039795525198,10.714055870666,-1.));
#7388=CARTESIAN_POINT('Ctrl Pts',(5.30178983253176,10.7011191580639,-1.));
#7389=CARTESIAN_POINT('Ctrl Pts',(5.25052377191006,10.6835982206291,-1.));
#7390=CARTESIAN_POINT('Ctrl Pts',(5.18679427410258,10.661243291145,-1.));
#7391=CARTESIAN_POINT('Ctrl Pts',(5.12341919820984,10.638434168447,-1.));
#7392=CARTESIAN_POINT('Ctrl Pts',(5.06040071098369,10.6151706715837,-1.));
#7393=CARTESIAN_POINT('Ctrl Pts',(4.99774193408264,10.5914530920551,-1.));
#7394=CARTESIAN_POINT('Ctrl Pts',(4.93544714999767,10.5672824880187,-1.));
#7395=CARTESIAN_POINT('Ctrl Pts',(4.87352158939686,10.5426605691059,-1.));
#7396=CARTESIAN_POINT('Ctrl Pts',(4.81197108362035,10.5175894490106,-1.));
#7397=CARTESIAN_POINT('Ctrl Pts',(4.7508017470924,10.4920714379865,-1.));
#7398=CARTESIAN_POINT('Ctrl Pts',(4.69001967404875,10.4661088391609,-1.));
#7399=CARTESIAN_POINT('Ctrl Pts',(4.62963055491846,10.4397037052484,-1.));
#7400=CARTESIAN_POINT('Ctrl Pts',(4.56963961142454,10.4128577818052,-1.));
#7401=CARTESIAN_POINT('Ctrl Pts',(4.5100518320603,10.3855726289458,-1.));
#7402=CARTESIAN_POINT('Ctrl Pts',(4.45087212698485,10.3578496987941,-1.));
#7403=CARTESIAN_POINT('Ctrl Pts',(4.39210550098945,10.3296904287044,-1.));
#7404=CARTESIAN_POINT('Ctrl Pts',(4.33375724408484,10.3010963438997,-1.));
#7405=CARTESIAN_POINT('Ctrl Pts',(4.27583301771353,10.272069116189,-1.));
#7406=CARTESIAN_POINT('Ctrl Pts',(4.21833871177567,10.2426105188232,-1.));
#7407=CARTESIAN_POINT('Ctrl Pts',(4.16128034451962,10.2127224064663,-1.));
#7408=CARTESIAN_POINT('Ctrl Pts',(4.10466394929486,10.1824066879509,-1.));
#7409=CARTESIAN_POINT('Ctrl Pts',(4.04849544744087,10.1516653064199,-1.));
#7410=CARTESIAN_POINT('Ctrl Pts',(3.99278057289046,10.1205002164952,-1.));
#7411=CARTESIAN_POINT('Ctrl Pts',(3.93752506012707,10.0889133486827,-1.));
#7412=CARTESIAN_POINT('Ctrl Pts',(3.88273479532263,10.056906577166,-1.));
#7413=CARTESIAN_POINT('Ctrl Pts',(3.82841597408715,10.0244816905709,-1.));
#7414=CARTESIAN_POINT('Ctrl Pts',(3.77457526401004,9.99164036147395,-1.));
#7415=CARTESIAN_POINT('Ctrl Pts',(3.72121993173636,9.95838412799172,-1.));
#7416=CARTESIAN_POINT('Ctrl Pts',(3.66835753420625,9.92471449880883,-1.));
#7417=CARTESIAN_POINT('Ctrl Pts',(3.61599563628969,9.89063305253546,-1.));
#7418=CARTESIAN_POINT('Ctrl Pts',(3.56414151726151,9.85614154137781,-1.));
#7419=CARTESIAN_POINT('Ctrl Pts',(3.51280187273295,9.8212419982557,-1.));
#7420=CARTESIAN_POINT('Ctrl Pts',(3.46198252886957,9.78593684022037,-1.));
#7421=CARTESIAN_POINT('Ctrl Pts',(3.41168916880891,9.75022858813702,-1.));
#7422=CARTESIAN_POINT('Ctrl Pts',(3.36192803839197,9.7141195953304,-1.));
#7423=CARTESIAN_POINT('Ctrl Pts',(3.31270665744062,9.67761177523123,-1.));
#7424=CARTESIAN_POINT('Ctrl Pts',(3.26403452382222,9.64070633286081,-1.));
#7425=CARTESIAN_POINT('Ctrl Pts',(3.2159238260067,9.60340349406962,-1.));
#7426=CARTESIAN_POINT('Ctrl Pts',(3.16838785383004,9.56570313257491,-1.));
#7427=CARTESIAN_POINT('Ctrl Pts',(3.12143939300699,9.52760540436562,-1.));
#7428=CARTESIAN_POINT('Ctrl Pts',(3.07508913212204,9.4891113781729,-1.));
#7429=CARTESIAN_POINT('Ctrl Pts',(3.02934403325601,9.4502236812248,-1.));
#7430=CARTESIAN_POINT('Ctrl Pts',(2.98420577513996,9.4109471173216,-1.));
#7431=CARTESIAN_POINT('Ctrl Pts',(2.9396747031485,9.3712871143499,-1.));
#7432=CARTESIAN_POINT('Ctrl Pts',(2.89575377593938,9.33124817395869,-1.));
#7433=CARTESIAN_POINT('Ctrl Pts',(2.8524523828002,9.29083237315974,-1.));
#7434=CARTESIAN_POINT('Ctrl Pts',(2.8097905150733,9.2500377269296,-1.));
#7435=CARTESIAN_POINT('Ctrl Pts',(2.76780196452137,9.20885693589776,-1.));
#7436=CARTESIAN_POINT('Ctrl Pts',(2.72652481622916,9.16728115317076,-1.));
#7437=CARTESIAN_POINT('Ctrl Pts',(2.68599232523134,9.12530360007999,-1.));
#7438=CARTESIAN_POINT('Ctrl Pts',(2.64622438896052,9.08292294803309,-1.));
#7439=CARTESIAN_POINT('Ctrl Pts',(2.60721699951879,9.0401474973841,-1.));
#7440=CARTESIAN_POINT('Ctrl Pts',(2.56893767747319,8.99699699918147,-1.));
#7441=CARTESIAN_POINT('Ctrl Pts',(2.53134978004338,8.95349309713545,-1.));
#7442=CARTESIAN_POINT('Ctrl Pts',(2.4944346415182,8.90965062344541,-1.));
#7443=CARTESIAN_POINT('Ctrl Pts',(2.45821141167119,8.86546980570045,-1.));
#7444=CARTESIAN_POINT('Ctrl Pts',(2.42276538248091,8.82092512134556,-1.));
#7445=CARTESIAN_POINT('Ctrl Pts',(2.38824857383288,8.77596511266658,-1.));
#7446=CARTESIAN_POINT('Ctrl Pts',(2.35482147675118,8.73053548487858,-1.));
#7447=CARTESIAN_POINT('Ctrl Pts',(2.32260171926006,8.68459942442028,-1.));
#7448=CARTESIAN_POINT('Ctrl Pts',(2.29162050823336,8.63815494571075,-1.));
#7449=CARTESIAN_POINT('Ctrl Pts',(2.26174990860571,8.59126351952004,-1.));
#7450=CARTESIAN_POINT('Ctrl Pts',(2.23274297834755,8.54403497990068,-1.));
#7451=CARTESIAN_POINT('Ctrl Pts',(2.20438215159743,8.49657041043195,-1.));
#7452=CARTESIAN_POINT('Ctrl Pts',(2.17660700812682,8.44891314968814,-1.));
#7453=CARTESIAN_POINT('Ctrl Pts',(2.1496314108288,8.40100363162428,-1.));
#7454=CARTESIAN_POINT('Ctrl Pts',(2.12411443763999,8.35261410600662,-1.));
#7455=CARTESIAN_POINT('Ctrl Pts',(2.10101049300138,8.3034037182712,-1.));
#7456=CARTESIAN_POINT('Ctrl Pts',(2.08524426770063,8.26309465918435,-1.));
#7457=CARTESIAN_POINT('Ctrl Pts',(2.07530073900944,8.23220544002367,-1.));
#7458=CARTESIAN_POINT('Ctrl Pts',(2.06955313972063,8.21130388109186,-1.));
#7459=CARTESIAN_POINT('Ctrl Pts',(2.066899701215,8.20077591276801,-1.));
#7460=CARTESIAN_POINT('',(5.3791293750062,10.7268339768519,6.));
#7461=CARTESIAN_POINT('Ctrl Pts',(5.37912937500617,10.726833976852,6.));
#7462=CARTESIAN_POINT('Ctrl Pts',(5.36620715918271,10.7225897134991,6.));
#7463=CARTESIAN_POINT('Ctrl Pts',(5.34039795525198,10.714055870666,6.));
#7464=CARTESIAN_POINT('Ctrl Pts',(5.30178983253176,10.7011191580639,6.));
#7465=CARTESIAN_POINT('Ctrl Pts',(5.25052377191006,10.6835982206291,6.));
#7466=CARTESIAN_POINT('Ctrl Pts',(5.18679427410258,10.661243291145,6.));
#7467=CARTESIAN_POINT('Ctrl Pts',(5.12341919820984,10.638434168447,6.));
#7468=CARTESIAN_POINT('Ctrl Pts',(5.06040071098369,10.6151706715837,6.));
#7469=CARTESIAN_POINT('Ctrl Pts',(4.99774193408264,10.5914530920551,6.));
#7470=CARTESIAN_POINT('Ctrl Pts',(4.93544714999767,10.5672824880187,6.));
#7471=CARTESIAN_POINT('Ctrl Pts',(4.87352158939686,10.5426605691059,6.));
#7472=CARTESIAN_POINT('Ctrl Pts',(4.81197108362035,10.5175894490106,6.));
#7473=CARTESIAN_POINT('Ctrl Pts',(4.7508017470924,10.4920714379865,6.));
#7474=CARTESIAN_POINT('Ctrl Pts',(4.69001967404875,10.4661088391609,6.));
#7475=CARTESIAN_POINT('Ctrl Pts',(4.62963055491846,10.4397037052484,6.));
#7476=CARTESIAN_POINT('Ctrl Pts',(4.56963961142454,10.4128577818052,6.));
#7477=CARTESIAN_POINT('Ctrl Pts',(4.5100518320603,10.3855726289458,6.));
#7478=CARTESIAN_POINT('Ctrl Pts',(4.45087212698485,10.3578496987941,6.));
#7479=CARTESIAN_POINT('Ctrl Pts',(4.39210550098945,10.3296904287044,6.));
#7480=CARTESIAN_POINT('Ctrl Pts',(4.33375724408484,10.3010963438997,6.));
#7481=CARTESIAN_POINT('Ctrl Pts',(4.27583301771353,10.272069116189,6.));
#7482=CARTESIAN_POINT('Ctrl Pts',(4.21833871177567,10.2426105188232,6.));
#7483=CARTESIAN_POINT('Ctrl Pts',(4.16128034451962,10.2127224064663,6.));
#7484=CARTESIAN_POINT('Ctrl Pts',(4.10466394929486,10.1824066879509,6.));
#7485=CARTESIAN_POINT('Ctrl Pts',(4.04849544744087,10.1516653064199,6.));
#7486=CARTESIAN_POINT('Ctrl Pts',(3.99278057289046,10.1205002164952,6.));
#7487=CARTESIAN_POINT('Ctrl Pts',(3.93752506012707,10.0889133486827,6.));
#7488=CARTESIAN_POINT('Ctrl Pts',(3.88273479532263,10.056906577166,6.));
#7489=CARTESIAN_POINT('Ctrl Pts',(3.82841597408715,10.0244816905709,6.));
#7490=CARTESIAN_POINT('Ctrl Pts',(3.77457526401004,9.99164036147395,6.));
#7491=CARTESIAN_POINT('Ctrl Pts',(3.72121993173636,9.95838412799172,6.));
#7492=CARTESIAN_POINT('Ctrl Pts',(3.66835753420625,9.92471449880883,6.));
#7493=CARTESIAN_POINT('Ctrl Pts',(3.61599563628969,9.89063305253546,6.));
#7494=CARTESIAN_POINT('Ctrl Pts',(3.56414151726151,9.85614154137781,6.));
#7495=CARTESIAN_POINT('Ctrl Pts',(3.51280187273295,9.8212419982557,6.));
#7496=CARTESIAN_POINT('Ctrl Pts',(3.46198252886957,9.78593684022037,6.));
#7497=CARTESIAN_POINT('Ctrl Pts',(3.41168916880891,9.75022858813702,6.));
#7498=CARTESIAN_POINT('Ctrl Pts',(3.36192803839197,9.7141195953304,6.));
#7499=CARTESIAN_POINT('Ctrl Pts',(3.31270665744062,9.67761177523123,6.));
#7500=CARTESIAN_POINT('Ctrl Pts',(3.26403452382222,9.64070633286081,6.));
#7501=CARTESIAN_POINT('Ctrl Pts',(3.2159238260067,9.60340349406962,6.));
#7502=CARTESIAN_POINT('Ctrl Pts',(3.16838785383004,9.56570313257491,6.));
#7503=CARTESIAN_POINT('Ctrl Pts',(3.12143939300699,9.52760540436562,6.));
#7504=CARTESIAN_POINT('Ctrl Pts',(3.07508913212204,9.4891113781729,6.));
#7505=CARTESIAN_POINT('Ctrl Pts',(3.02934403325601,9.4502236812248,6.));
#7506=CARTESIAN_POINT('Ctrl Pts',(2.98420577513996,9.4109471173216,6.));
#7507=CARTESIAN_POINT('Ctrl Pts',(2.9396747031485,9.3712871143499,6.));
#7508=CARTESIAN_POINT('Ctrl Pts',(2.89575377593938,9.33124817395869,6.));
#7509=CARTESIAN_POINT('Ctrl Pts',(2.8524523828002,9.29083237315974,6.));
#7510=CARTESIAN_POINT('Ctrl Pts',(2.8097905150733,9.2500377269296,6.));
#7511=CARTESIAN_POINT('Ctrl Pts',(2.76780196452137,9.20885693589776,6.));
#7512=CARTESIAN_POINT('Ctrl Pts',(2.72652481622916,9.16728115317076,6.));
#7513=CARTESIAN_POINT('Ctrl Pts',(2.68599232523134,9.12530360007999,6.));
#7514=CARTESIAN_POINT('Ctrl Pts',(2.64622438896052,9.08292294803309,6.));
#7515=CARTESIAN_POINT('Ctrl Pts',(2.60721699951879,9.0401474973841,6.));
#7516=CARTESIAN_POINT('Ctrl Pts',(2.56893767747319,8.99699699918147,6.));
#7517=CARTESIAN_POINT('Ctrl Pts',(2.53134978004338,8.95349309713545,6.));
#7518=CARTESIAN_POINT('Ctrl Pts',(2.4944346415182,8.90965062344541,6.));
#7519=CARTESIAN_POINT('Ctrl Pts',(2.45821141167119,8.86546980570045,6.));
#7520=CARTESIAN_POINT('Ctrl Pts',(2.42276538248091,8.82092512134556,6.));
#7521=CARTESIAN_POINT('Ctrl Pts',(2.38824857383288,8.77596511266658,6.));
#7522=CARTESIAN_POINT('Ctrl Pts',(2.35482147675118,8.73053548487858,6.));
#7523=CARTESIAN_POINT('Ctrl Pts',(2.32260171926006,8.68459942442028,6.));
#7524=CARTESIAN_POINT('Ctrl Pts',(2.29162050823336,8.63815494571075,6.));
#7525=CARTESIAN_POINT('Ctrl Pts',(2.26174990860571,8.59126351952004,6.));
#7526=CARTESIAN_POINT('Ctrl Pts',(2.23274297834755,8.54403497990068,6.));
#7527=CARTESIAN_POINT('Ctrl Pts',(2.20438215159743,8.49657041043195,6.));
#7528=CARTESIAN_POINT('Ctrl Pts',(2.17660700812682,8.44891314968814,6.));
#7529=CARTESIAN_POINT('Ctrl Pts',(2.1496314108288,8.40100363162428,6.));
#7530=CARTESIAN_POINT('Ctrl Pts',(2.12411443763999,8.35261410600662,6.));
#7531=CARTESIAN_POINT('Ctrl Pts',(2.10101049300138,8.3034037182712,6.));
#7532=CARTESIAN_POINT('Ctrl Pts',(2.08524426770063,8.26309465918435,6.));
#7533=CARTESIAN_POINT('Ctrl Pts',(2.07530073900944,8.23220544002367,6.));
#7534=CARTESIAN_POINT('Ctrl Pts',(2.06955313972063,8.21130388109186,6.));
#7535=CARTESIAN_POINT('Ctrl Pts',(2.066899701215,8.20077591276801,6.));
#7536=CARTESIAN_POINT('',(5.3791293750062,10.7268339768519,0.));
#7537=CARTESIAN_POINT('Origin',(1.99840144432528E-13,3.46133283549042E-13,
0.));
#7538=CARTESIAN_POINT('',(6.60014603862877,10.0218796774244,-1.));
#7539=CARTESIAN_POINT('Origin',(1.99840144432528E-13,3.46133283549042E-13,
-1.));
#7540=CARTESIAN_POINT('',(6.60014603862877,10.0218796774244,6.));
#7541=CARTESIAN_POINT('Origin',(1.99840144432528E-13,3.46133283549042E-13,
6.));
#7542=CARTESIAN_POINT('',(6.60014603862877,10.0218796774244,0.));
#7543=CARTESIAN_POINT('Ctrl Pts',(6.06863042059311,5.89037560471066,-3.75));
#7544=CARTESIAN_POINT('Ctrl Pts',(6.06863042059311,5.89037560471066,12.75));
#7545=CARTESIAN_POINT('Ctrl Pts',(6.07642118935899,5.89793753402584,-3.75));
#7546=CARTESIAN_POINT('Ctrl Pts',(6.07642118935899,5.89793753402584,12.75));
#7547=CARTESIAN_POINT('Ctrl Pts',(6.09164867072823,5.91336588048663,-3.75));
#7548=CARTESIAN_POINT('Ctrl Pts',(6.09164867072823,5.91336588048663,12.75));
#7549=CARTESIAN_POINT('Ctrl Pts',(6.11342775487885,5.93742183851679,-3.75));
#7550=CARTESIAN_POINT('Ctrl Pts',(6.11342775487885,5.93742183851679,12.75));
#7551=CARTESIAN_POINT('Ctrl Pts',(6.14045331140034,5.97123031969246,-3.75));
#7552=CARTESIAN_POINT('Ctrl Pts',(6.14045331140034,5.97123031969246,12.75));
#7553=CARTESIAN_POINT('Ctrl Pts',(6.17151878498999,6.01584411654484,-3.75));
#7554=CARTESIAN_POINT('Ctrl Pts',(6.17151878498999,6.01584411654484,12.75));
#7555=CARTESIAN_POINT('Ctrl Pts',(6.20066685685755,6.06213722636286,-3.75));
#7556=CARTESIAN_POINT('Ctrl Pts',(6.20066685685755,6.06213722636286,12.75));
#7557=CARTESIAN_POINT('Ctrl Pts',(6.22866991793492,6.10945353793713,-3.75));
#7558=CARTESIAN_POINT('Ctrl Pts',(6.22866991793492,6.10945353793713,12.75));
#7559=CARTESIAN_POINT('Ctrl Pts',(6.25605474467853,6.15733614814835,-3.75));
#7560=CARTESIAN_POINT('Ctrl Pts',(6.25605474467853,6.15733614814835,12.75));
#7561=CARTESIAN_POINT('Ctrl Pts',(6.28297985424308,6.20562962932065,-3.75));
#7562=CARTESIAN_POINT('Ctrl Pts',(6.28297985424308,6.20562962932065,12.75));
#7563=CARTESIAN_POINT('Ctrl Pts',(6.30937750420801,6.2543646376197,-3.75));
#7564=CARTESIAN_POINT('Ctrl Pts',(6.30937750420801,6.2543646376197,12.75));
#7565=CARTESIAN_POINT('Ctrl Pts',(6.33505137069502,6.30367904881887,-3.75));
#7566=CARTESIAN_POINT('Ctrl Pts',(6.33505137069502,6.30367904881887,12.75));
#7567=CARTESIAN_POINT('Ctrl Pts',(6.35978286360965,6.35373180396277,-3.75));
#7568=CARTESIAN_POINT('Ctrl Pts',(6.35978286360965,6.35373180396277,12.75));
#7569=CARTESIAN_POINT('Ctrl Pts',(6.38345478017076,6.40460296268299,-3.75));
#7570=CARTESIAN_POINT('Ctrl Pts',(6.38345478017076,6.40460296268299,12.75));
#7571=CARTESIAN_POINT('Ctrl Pts',(6.40608444337878,6.45626649182452,-3.75));
#7572=CARTESIAN_POINT('Ctrl Pts',(6.40608444337878,6.45626649182452,12.75));
#7573=CARTESIAN_POINT('Ctrl Pts',(6.42776254872513,6.50863892931076,-3.75));
#7574=CARTESIAN_POINT('Ctrl Pts',(6.42776254872513,6.50863892931076,12.75));
#7575=CARTESIAN_POINT('Ctrl Pts',(6.44861636238489,6.56160843323028,-3.75));
#7576=CARTESIAN_POINT('Ctrl Pts',(6.44861636238489,6.56160843323028,12.75));
#7577=CARTESIAN_POINT('Ctrl Pts',(6.46876645798849,6.6150690793574,-3.75));
#7578=CARTESIAN_POINT('Ctrl Pts',(6.46876645798849,6.6150690793574,12.75));
#7579=CARTESIAN_POINT('Ctrl Pts',(6.48827758470623,6.66895976394944,-3.75));
#7580=CARTESIAN_POINT('Ctrl Pts',(6.48827758470623,6.66895976394944,12.75));
#7581=CARTESIAN_POINT('Ctrl Pts',(6.50715912032692,6.72326378902151,-3.75));
#7582=CARTESIAN_POINT('Ctrl Pts',(6.50715912032692,6.72326378902151,12.75));
#7583=CARTESIAN_POINT('Ctrl Pts',(6.52538888693356,6.77798990345396,-3.75));
#7584=CARTESIAN_POINT('Ctrl Pts',(6.52538888693356,6.77798990345396,12.75));
#7585=CARTESIAN_POINT('Ctrl Pts',(6.54292981913304,6.83315901897031,-3.75));
#7586=CARTESIAN_POINT('Ctrl Pts',(6.54292981913304,6.83315901897031,12.75));
#7587=CARTESIAN_POINT('Ctrl Pts',(6.5597485722992,6.88878938806037,-3.75));
#7588=CARTESIAN_POINT('Ctrl Pts',(6.5597485722992,6.88878938806037,12.75));
#7589=CARTESIAN_POINT('Ctrl Pts',(6.5758359541656,6.94488033148853,-3.75));
#7590=CARTESIAN_POINT('Ctrl Pts',(6.5758359541656,6.94488033148853,12.75));
#7591=CARTESIAN_POINT('Ctrl Pts',(6.5912030640433,7.00141528186886,-3.75));
#7592=CARTESIAN_POINT('Ctrl Pts',(6.5912030640433,7.00141528186886,12.75));
#7593=CARTESIAN_POINT('Ctrl Pts',(6.60587239994885,7.05836882883084,-3.75));
#7594=CARTESIAN_POINT('Ctrl Pts',(6.60587239994885,7.05836882883084,12.75));
#7595=CARTESIAN_POINT('Ctrl Pts',(6.61987066605911,7.11571241317029,-3.75));
#7596=CARTESIAN_POINT('Ctrl Pts',(6.61987066605911,7.11571241317029,12.75));
#7597=CARTESIAN_POINT('Ctrl Pts',(6.63322107969569,7.17342042004755,-3.75));
#7598=CARTESIAN_POINT('Ctrl Pts',(6.63322107969569,7.17342042004755,12.75));
#7599=CARTESIAN_POINT('Ctrl Pts',(6.64593535561053,7.23147652896403,-3.75));
#7600=CARTESIAN_POINT('Ctrl Pts',(6.64593535561053,7.23147652896403,12.75));
#7601=CARTESIAN_POINT('Ctrl Pts',(6.65801638970246,7.28987157005223,-3.75));
#7602=CARTESIAN_POINT('Ctrl Pts',(6.65801638970246,7.28987157005223,12.75));
#7603=CARTESIAN_POINT('Ctrl Pts',(6.66946176275797,7.34860073021491,-3.75));
#7604=CARTESIAN_POINT('Ctrl Pts',(6.66946176275797,7.34860073021491,12.75));
#7605=CARTESIAN_POINT('Ctrl Pts',(6.68026694677668,7.40766099640557,-3.75));
#7606=CARTESIAN_POINT('Ctrl Pts',(6.68026694677668,7.40766099640557,12.75));
#7607=CARTESIAN_POINT('Ctrl Pts',(6.69042862091104,7.46704851290034,-3.75));
#7608=CARTESIAN_POINT('Ctrl Pts',(6.69042862091104,7.46704851290034,12.75));
#7609=CARTESIAN_POINT('Ctrl Pts',(6.69994799095524,7.52675593674632,-3.75));
#7610=CARTESIAN_POINT('Ctrl Pts',(6.69994799095524,7.52675593674632,12.75));
#7611=CARTESIAN_POINT('Ctrl Pts',(6.70882947565318,7.58677347699226,-3.75));
#7612=CARTESIAN_POINT('Ctrl Pts',(6.70882947565318,7.58677347699226,12.75));
#7613=CARTESIAN_POINT('Ctrl Pts',(6.71707933277187,7.64708998288989,-3.75));
#7614=CARTESIAN_POINT('Ctrl Pts',(6.71707933277187,7.64708998288989,12.75));
#7615=CARTESIAN_POINT('Ctrl Pts',(6.72470431659336,7.70769400824503,-3.75));
#7616=CARTESIAN_POINT('Ctrl Pts',(6.72470431659336,7.70769400824503,12.75));
#7617=CARTESIAN_POINT('Ctrl Pts',(6.73171032576036,7.76857488460783,-3.75));
#7618=CARTESIAN_POINT('Ctrl Pts',(6.73171032576036,7.76857488460783,12.75));
#7619=CARTESIAN_POINT('Ctrl Pts',(6.73810106562749,7.82972378407324,-3.75));
#7620=CARTESIAN_POINT('Ctrl Pts',(6.73810106562749,7.82972378407324,12.75));
#7621=CARTESIAN_POINT('Ctrl Pts',(6.74387863902608,7.89113323756912,-3.75));
#7622=CARTESIAN_POINT('Ctrl Pts',(6.74387863902608,7.89113323756912,12.75));
#7623=CARTESIAN_POINT('Ctrl Pts',(6.7490441308376,7.95279665937614,-3.75));
#7624=CARTESIAN_POINT('Ctrl Pts',(6.7490441308376,7.95279665937614,12.75));
#7625=CARTESIAN_POINT('Ctrl Pts',(6.75359819949754,8.01470786732018,-3.75));
#7626=CARTESIAN_POINT('Ctrl Pts',(6.75359819949754,8.01470786732018,12.75));
#7627=CARTESIAN_POINT('Ctrl Pts',(6.75754166486089,8.07686060726827,-3.75));
#7628=CARTESIAN_POINT('Ctrl Pts',(6.75754166486089,8.07686060726827,12.75));
#7629=CARTESIAN_POINT('Ctrl Pts',(6.76087611417306,8.13924806419107,-3.75));
#7630=CARTESIAN_POINT('Ctrl Pts',(6.76087611417306,8.13924806419107,12.75));
#7631=CARTESIAN_POINT('Ctrl Pts',(6.7636036696164,8.20186305794855,-3.75));
#7632=CARTESIAN_POINT('Ctrl Pts',(6.7636036696164,8.20186305794855,12.75));
#7633=CARTESIAN_POINT('Ctrl Pts',(6.76572674650935,8.26469824786602,-3.75));
#7634=CARTESIAN_POINT('Ctrl Pts',(6.76572674650935,8.26469824786602,12.75));
#7635=CARTESIAN_POINT('Ctrl Pts',(6.76724781676282,8.32774633509908,-3.75));
#7636=CARTESIAN_POINT('Ctrl Pts',(6.76724781676282,8.32774633509908,12.75));
#7637=CARTESIAN_POINT('Ctrl Pts',(6.76816918165128,8.39100025749018,-3.75));
#7638=CARTESIAN_POINT('Ctrl Pts',(6.76816918165128,8.39100025749018,12.75));
#7639=CARTESIAN_POINT('Ctrl Pts',(6.76849272647565,8.45445340444926,-3.75));
#7640=CARTESIAN_POINT('Ctrl Pts',(6.76849272647565,8.45445340444926,12.75));
#7641=CARTESIAN_POINT('Ctrl Pts',(6.76822000004555,8.51809951610774,-3.75));
#7642=CARTESIAN_POINT('Ctrl Pts',(6.76822000004555,8.51809951610774,12.75));
#7643=CARTESIAN_POINT('Ctrl Pts',(6.76735232235635,8.58193255779939,-3.75));
#7644=CARTESIAN_POINT('Ctrl Pts',(6.76735232235635,8.58193255779939,12.75));
#7645=CARTESIAN_POINT('Ctrl Pts',(6.76589088878265,8.64594659806298,-3.75));
#7646=CARTESIAN_POINT('Ctrl Pts',(6.76589088878265,8.64594659806298,12.75));
#7647=CARTESIAN_POINT('Ctrl Pts',(6.76383687353853,8.71013569385599,-3.75));
#7648=CARTESIAN_POINT('Ctrl Pts',(6.76383687353853,8.71013569385599,12.75));
#7649=CARTESIAN_POINT('Ctrl Pts',(6.76119155448275,8.77449374557664,-3.75));
#7650=CARTESIAN_POINT('Ctrl Pts',(6.76119155448275,8.77449374557664,12.75));
#7651=CARTESIAN_POINT('Ctrl Pts',(6.7579562951925,8.83901457377471,-3.75));
#7652=CARTESIAN_POINT('Ctrl Pts',(6.7579562951925,8.83901457377471,12.75));
#7653=CARTESIAN_POINT('Ctrl Pts',(6.75413249860576,8.90369203916218,-3.75));
#7654=CARTESIAN_POINT('Ctrl Pts',(6.75413249860576,8.90369203916218,12.75));
#7655=CARTESIAN_POINT('Ctrl Pts',(6.74972157399229,8.96852015431046,-3.75));
#7656=CARTESIAN_POINT('Ctrl Pts',(6.74972157399229,8.96852015431046,12.75));
#7657=CARTESIAN_POINT('Ctrl Pts',(6.74472490424422,9.03349318036198,-3.75));
#7658=CARTESIAN_POINT('Ctrl Pts',(6.74472490424422,9.03349318036198,12.75));
#7659=CARTESIAN_POINT('Ctrl Pts',(6.73914381348523,9.09860577342165,-3.75));
#7660=CARTESIAN_POINT('Ctrl Pts',(6.73914381348523,9.09860577342165,12.75));
#7661=CARTESIAN_POINT('Ctrl Pts',(6.73297955932548,9.16385288053588,-3.75));
#7662=CARTESIAN_POINT('Ctrl Pts',(6.73297955932548,9.16385288053588,12.75));
#7663=CARTESIAN_POINT('Ctrl Pts',(6.72623333926846,9.22922952332026,-3.75));
#7664=CARTESIAN_POINT('Ctrl Pts',(6.72623333926846,9.22922952332026,12.75));
#7665=CARTESIAN_POINT('Ctrl Pts',(6.71890629646187,9.2947306015555,-3.75));
#7666=CARTESIAN_POINT('Ctrl Pts',(6.71890629646187,9.2947306015555,12.75));
#7667=CARTESIAN_POINT('Ctrl Pts',(6.71099953007124,9.36035072031876,-3.75));
#7668=CARTESIAN_POINT('Ctrl Pts',(6.71099953007124,9.36035072031876,12.75));
#7669=CARTESIAN_POINT('Ctrl Pts',(6.70251410760819,9.42608392519666,-3.75));
#7670=CARTESIAN_POINT('Ctrl Pts',(6.70251410760819,9.42608392519666,12.75));
#7671=CARTESIAN_POINT('Ctrl Pts',(6.69345108162377,9.49192378686253,-3.75));
#7672=CARTESIAN_POINT('Ctrl Pts',(6.69345108162377,9.49192378686253,12.75));
#7673=CARTESIAN_POINT('Ctrl Pts',(6.68381150859182,9.55786385494286,-3.75));
#7674=CARTESIAN_POINT('Ctrl Pts',(6.68381150859182,9.55786385494286,12.75));
#7675=CARTESIAN_POINT('Ctrl Pts',(6.67359647366961,9.62389802250188,-3.75));
#7676=CARTESIAN_POINT('Ctrl Pts',(6.67359647366961,9.62389802250188,12.75));
#7677=CARTESIAN_POINT('Ctrl Pts',(6.66280711160719,9.69002090483258,-3.75));
#7678=CARTESIAN_POINT('Ctrl Pts',(6.66280711160719,9.69002090483258,12.75));
#7679=CARTESIAN_POINT('Ctrl Pts',(6.65144464725859,9.75622826411013,-3.75));
#7680=CARTESIAN_POINT('Ctrl Pts',(6.65144464725859,9.75622826411013,12.75));
#7681=CARTESIAN_POINT('Ctrl Pts',(6.63951038900667,9.82251725114898,-3.75));
#7682=CARTESIAN_POINT('Ctrl Pts',(6.63951038900667,9.82251725114898,12.75));
#7683=CARTESIAN_POINT('Ctrl Pts',(6.62700557693596,9.88888607996273,-3.75));
#7684=CARTESIAN_POINT('Ctrl Pts',(6.62700557693596,9.88888607996273,12.75));
#7685=CARTESIAN_POINT('Ctrl Pts',(6.61654612354183,9.94204425953052,-3.75));
#7686=CARTESIAN_POINT('Ctrl Pts',(6.61654612354183,9.94204425953052,12.75));
#7687=CARTESIAN_POINT('Ctrl Pts',(6.60844558393656,9.98194823089968,-3.75));
#7688=CARTESIAN_POINT('Ctrl Pts',(6.60844558393656,9.98194823089968,12.75));
#7689=CARTESIAN_POINT('Ctrl Pts',(6.60293150665659,10.0085665785717,-3.75));
#7690=CARTESIAN_POINT('Ctrl Pts',(6.60293150665659,10.0085665785717,12.75));
#7691=CARTESIAN_POINT('Ctrl Pts',(6.60014603862877,10.0218796774244,-3.75));
#7692=CARTESIAN_POINT('Ctrl Pts',(6.60014603862877,10.0218796774244,12.75));
#7693=CARTESIAN_POINT('Ctrl Pts',(6.06863042059311,5.89037560471066,-1.));
#7694=CARTESIAN_POINT('Ctrl Pts',(6.07642118935899,5.89793753402584,-1.));
#7695=CARTESIAN_POINT('Ctrl Pts',(6.09164867072823,5.91336588048663,-1.));
#7696=CARTESIAN_POINT('Ctrl Pts',(6.11342775487885,5.93742183851679,-1.));
#7697=CARTESIAN_POINT('Ctrl Pts',(6.14045331140034,5.97123031969246,-1.));
#7698=CARTESIAN_POINT('Ctrl Pts',(6.17151878498999,6.01584411654484,-1.));
#7699=CARTESIAN_POINT('Ctrl Pts',(6.20066685685755,6.06213722636286,-1.));
#7700=CARTESIAN_POINT('Ctrl Pts',(6.22866991793492,6.10945353793713,-1.));
#7701=CARTESIAN_POINT('Ctrl Pts',(6.25605474467853,6.15733614814835,-1.));
#7702=CARTESIAN_POINT('Ctrl Pts',(6.28297985424308,6.20562962932065,-1.));
#7703=CARTESIAN_POINT('Ctrl Pts',(6.30937750420801,6.2543646376197,-1.));
#7704=CARTESIAN_POINT('Ctrl Pts',(6.33505137069502,6.30367904881887,-1.));
#7705=CARTESIAN_POINT('Ctrl Pts',(6.35978286360965,6.35373180396277,-1.));
#7706=CARTESIAN_POINT('Ctrl Pts',(6.38345478017076,6.40460296268299,-1.));
#7707=CARTESIAN_POINT('Ctrl Pts',(6.40608444337878,6.45626649182452,-1.));
#7708=CARTESIAN_POINT('Ctrl Pts',(6.42776254872513,6.50863892931076,-1.));
#7709=CARTESIAN_POINT('Ctrl Pts',(6.44861636238489,6.56160843323028,-1.));
#7710=CARTESIAN_POINT('Ctrl Pts',(6.46876645798849,6.6150690793574,-1.));
#7711=CARTESIAN_POINT('Ctrl Pts',(6.48827758470623,6.66895976394944,-1.));
#7712=CARTESIAN_POINT('Ctrl Pts',(6.50715912032692,6.72326378902151,-1.));
#7713=CARTESIAN_POINT('Ctrl Pts',(6.52538888693356,6.77798990345396,-1.));
#7714=CARTESIAN_POINT('Ctrl Pts',(6.54292981913304,6.83315901897031,-1.));
#7715=CARTESIAN_POINT('Ctrl Pts',(6.5597485722992,6.88878938806037,-1.));
#7716=CARTESIAN_POINT('Ctrl Pts',(6.5758359541656,6.94488033148853,-1.));
#7717=CARTESIAN_POINT('Ctrl Pts',(6.5912030640433,7.00141528186886,-1.));
#7718=CARTESIAN_POINT('Ctrl Pts',(6.60587239994885,7.05836882883084,-1.));
#7719=CARTESIAN_POINT('Ctrl Pts',(6.61987066605911,7.11571241317029,-1.));
#7720=CARTESIAN_POINT('Ctrl Pts',(6.63322107969569,7.17342042004755,-1.));
#7721=CARTESIAN_POINT('Ctrl Pts',(6.64593535561053,7.23147652896403,-1.));
#7722=CARTESIAN_POINT('Ctrl Pts',(6.65801638970246,7.28987157005223,-1.));
#7723=CARTESIAN_POINT('Ctrl Pts',(6.66946176275797,7.34860073021491,-1.));
#7724=CARTESIAN_POINT('Ctrl Pts',(6.68026694677668,7.40766099640557,-1.));
#7725=CARTESIAN_POINT('Ctrl Pts',(6.69042862091104,7.46704851290034,-1.));
#7726=CARTESIAN_POINT('Ctrl Pts',(6.69994799095524,7.52675593674632,-1.));
#7727=CARTESIAN_POINT('Ctrl Pts',(6.70882947565318,7.58677347699226,-1.));
#7728=CARTESIAN_POINT('Ctrl Pts',(6.71707933277187,7.64708998288989,-1.));
#7729=CARTESIAN_POINT('Ctrl Pts',(6.72470431659336,7.70769400824503,-1.));
#7730=CARTESIAN_POINT('Ctrl Pts',(6.73171032576036,7.76857488460783,-1.));
#7731=CARTESIAN_POINT('Ctrl Pts',(6.73810106562749,7.82972378407324,-1.));
#7732=CARTESIAN_POINT('Ctrl Pts',(6.74387863902608,7.89113323756912,-1.));
#7733=CARTESIAN_POINT('Ctrl Pts',(6.7490441308376,7.95279665937614,-1.));
#7734=CARTESIAN_POINT('Ctrl Pts',(6.75359819949754,8.01470786732018,-1.));
#7735=CARTESIAN_POINT('Ctrl Pts',(6.75754166486089,8.07686060726827,-1.));
#7736=CARTESIAN_POINT('Ctrl Pts',(6.76087611417306,8.13924806419107,-1.));
#7737=CARTESIAN_POINT('Ctrl Pts',(6.7636036696164,8.20186305794855,-1.));
#7738=CARTESIAN_POINT('Ctrl Pts',(6.76572674650935,8.26469824786602,-1.));
#7739=CARTESIAN_POINT('Ctrl Pts',(6.76724781676282,8.32774633509908,-1.));
#7740=CARTESIAN_POINT('Ctrl Pts',(6.76816918165128,8.39100025749018,-1.));
#7741=CARTESIAN_POINT('Ctrl Pts',(6.76849272647565,8.45445340444926,-1.));
#7742=CARTESIAN_POINT('Ctrl Pts',(6.76822000004555,8.51809951610774,-1.));
#7743=CARTESIAN_POINT('Ctrl Pts',(6.76735232235635,8.58193255779939,-1.));
#7744=CARTESIAN_POINT('Ctrl Pts',(6.76589088878265,8.64594659806298,-1.));
#7745=CARTESIAN_POINT('Ctrl Pts',(6.76383687353853,8.71013569385599,-1.));
#7746=CARTESIAN_POINT('Ctrl Pts',(6.76119155448275,8.77449374557664,-1.));
#7747=CARTESIAN_POINT('Ctrl Pts',(6.7579562951925,8.83901457377471,-1.));
#7748=CARTESIAN_POINT('Ctrl Pts',(6.75413249860576,8.90369203916218,-1.));
#7749=CARTESIAN_POINT('Ctrl Pts',(6.74972157399229,8.96852015431046,-1.));
#7750=CARTESIAN_POINT('Ctrl Pts',(6.74472490424422,9.03349318036198,-1.));
#7751=CARTESIAN_POINT('Ctrl Pts',(6.73914381348523,9.09860577342165,-1.));
#7752=CARTESIAN_POINT('Ctrl Pts',(6.73297955932548,9.16385288053588,-1.));
#7753=CARTESIAN_POINT('Ctrl Pts',(6.72623333926846,9.22922952332026,-1.));
#7754=CARTESIAN_POINT('Ctrl Pts',(6.71890629646187,9.2947306015555,-1.));
#7755=CARTESIAN_POINT('Ctrl Pts',(6.71099953007124,9.36035072031876,-1.));
#7756=CARTESIAN_POINT('Ctrl Pts',(6.70251410760819,9.42608392519666,-1.));
#7757=CARTESIAN_POINT('Ctrl Pts',(6.69345108162377,9.49192378686253,-1.));
#7758=CARTESIAN_POINT('Ctrl Pts',(6.68381150859182,9.55786385494286,-1.));
#7759=CARTESIAN_POINT('Ctrl Pts',(6.67359647366961,9.62389802250188,-1.));
#7760=CARTESIAN_POINT('Ctrl Pts',(6.66280711160719,9.69002090483258,-1.));
#7761=CARTESIAN_POINT('Ctrl Pts',(6.65144464725859,9.75622826411013,-1.));
#7762=CARTESIAN_POINT('Ctrl Pts',(6.63951038900667,9.82251725114898,-1.));
#7763=CARTESIAN_POINT('Ctrl Pts',(6.62700557693596,9.88888607996273,-1.));
#7764=CARTESIAN_POINT('Ctrl Pts',(6.61654612354183,9.94204425953052,-1.));
#7765=CARTESIAN_POINT('Ctrl Pts',(6.60844558393656,9.98194823089968,-1.));
#7766=CARTESIAN_POINT('Ctrl Pts',(6.60293150665659,10.0085665785717,-1.));
#7767=CARTESIAN_POINT('Ctrl Pts',(6.60014603862877,10.0218796774244,-1.));
#7768=CARTESIAN_POINT('Ctrl Pts',(6.06863042059311,5.89037560471066,6.));
#7769=CARTESIAN_POINT('Ctrl Pts',(6.07642118935899,5.89793753402584,6.));
#7770=CARTESIAN_POINT('Ctrl Pts',(6.09164867072823,5.91336588048663,6.));
#7771=CARTESIAN_POINT('Ctrl Pts',(6.11342775487885,5.93742183851679,6.));
#7772=CARTESIAN_POINT('Ctrl Pts',(6.14045331140034,5.97123031969246,6.));
#7773=CARTESIAN_POINT('Ctrl Pts',(6.17151878498999,6.01584411654484,6.));
#7774=CARTESIAN_POINT('Ctrl Pts',(6.20066685685755,6.06213722636286,6.));
#7775=CARTESIAN_POINT('Ctrl Pts',(6.22866991793492,6.10945353793713,6.));
#7776=CARTESIAN_POINT('Ctrl Pts',(6.25605474467853,6.15733614814835,6.));
#7777=CARTESIAN_POINT('Ctrl Pts',(6.28297985424308,6.20562962932065,6.));
#7778=CARTESIAN_POINT('Ctrl Pts',(6.30937750420801,6.2543646376197,6.));
#7779=CARTESIAN_POINT('Ctrl Pts',(6.33505137069502,6.30367904881887,6.));
#7780=CARTESIAN_POINT('Ctrl Pts',(6.35978286360965,6.35373180396277,6.));
#7781=CARTESIAN_POINT('Ctrl Pts',(6.38345478017076,6.40460296268299,6.));
#7782=CARTESIAN_POINT('Ctrl Pts',(6.40608444337878,6.45626649182452,6.));
#7783=CARTESIAN_POINT('Ctrl Pts',(6.42776254872513,6.50863892931076,6.));
#7784=CARTESIAN_POINT('Ctrl Pts',(6.44861636238489,6.56160843323028,6.));
#7785=CARTESIAN_POINT('Ctrl Pts',(6.46876645798849,6.6150690793574,6.));
#7786=CARTESIAN_POINT('Ctrl Pts',(6.48827758470623,6.66895976394944,6.));
#7787=CARTESIAN_POINT('Ctrl Pts',(6.50715912032692,6.72326378902151,6.));
#7788=CARTESIAN_POINT('Ctrl Pts',(6.52538888693356,6.77798990345396,6.));
#7789=CARTESIAN_POINT('Ctrl Pts',(6.54292981913304,6.83315901897031,6.));
#7790=CARTESIAN_POINT('Ctrl Pts',(6.5597485722992,6.88878938806037,6.));
#7791=CARTESIAN_POINT('Ctrl Pts',(6.5758359541656,6.94488033148853,6.));
#7792=CARTESIAN_POINT('Ctrl Pts',(6.5912030640433,7.00141528186886,6.));
#7793=CARTESIAN_POINT('Ctrl Pts',(6.60587239994885,7.05836882883084,6.));
#7794=CARTESIAN_POINT('Ctrl Pts',(6.61987066605911,7.11571241317029,6.));
#7795=CARTESIAN_POINT('Ctrl Pts',(6.63322107969569,7.17342042004755,6.));
#7796=CARTESIAN_POINT('Ctrl Pts',(6.64593535561053,7.23147652896403,6.));
#7797=CARTESIAN_POINT('Ctrl Pts',(6.65801638970246,7.28987157005223,6.));
#7798=CARTESIAN_POINT('Ctrl Pts',(6.66946176275797,7.34860073021491,6.));
#7799=CARTESIAN_POINT('Ctrl Pts',(6.68026694677668,7.40766099640557,6.));
#7800=CARTESIAN_POINT('Ctrl Pts',(6.69042862091104,7.46704851290034,6.));
#7801=CARTESIAN_POINT('Ctrl Pts',(6.69994799095524,7.52675593674632,6.));
#7802=CARTESIAN_POINT('Ctrl Pts',(6.70882947565318,7.58677347699226,6.));
#7803=CARTESIAN_POINT('Ctrl Pts',(6.71707933277187,7.64708998288989,6.));
#7804=CARTESIAN_POINT('Ctrl Pts',(6.72470431659336,7.70769400824503,6.));
#7805=CARTESIAN_POINT('Ctrl Pts',(6.73171032576036,7.76857488460783,6.));
#7806=CARTESIAN_POINT('Ctrl Pts',(6.73810106562749,7.82972378407324,6.));
#7807=CARTESIAN_POINT('Ctrl Pts',(6.74387863902608,7.89113323756912,6.));
#7808=CARTESIAN_POINT('Ctrl Pts',(6.7490441308376,7.95279665937614,6.));
#7809=CARTESIAN_POINT('Ctrl Pts',(6.75359819949754,8.01470786732018,6.));
#7810=CARTESIAN_POINT('Ctrl Pts',(6.75754166486089,8.07686060726827,6.));
#7811=CARTESIAN_POINT('Ctrl Pts',(6.76087611417306,8.13924806419107,6.));
#7812=CARTESIAN_POINT('Ctrl Pts',(6.7636036696164,8.20186305794855,6.));
#7813=CARTESIAN_POINT('Ctrl Pts',(6.76572674650935,8.26469824786602,6.));
#7814=CARTESIAN_POINT('Ctrl Pts',(6.76724781676282,8.32774633509908,6.));
#7815=CARTESIAN_POINT('Ctrl Pts',(6.76816918165128,8.39100025749018,6.));
#7816=CARTESIAN_POINT('Ctrl Pts',(6.76849272647565,8.45445340444926,6.));
#7817=CARTESIAN_POINT('Ctrl Pts',(6.76822000004555,8.51809951610774,6.));
#7818=CARTESIAN_POINT('Ctrl Pts',(6.76735232235635,8.58193255779939,6.));
#7819=CARTESIAN_POINT('Ctrl Pts',(6.76589088878265,8.64594659806298,6.));
#7820=CARTESIAN_POINT('Ctrl Pts',(6.76383687353853,8.71013569385599,6.));
#7821=CARTESIAN_POINT('Ctrl Pts',(6.76119155448275,8.77449374557664,6.));
#7822=CARTESIAN_POINT('Ctrl Pts',(6.7579562951925,8.83901457377471,6.));
#7823=CARTESIAN_POINT('Ctrl Pts',(6.75413249860576,8.90369203916218,6.));
#7824=CARTESIAN_POINT('Ctrl Pts',(6.74972157399229,8.96852015431046,6.));
#7825=CARTESIAN_POINT('Ctrl Pts',(6.74472490424422,9.03349318036198,6.));
#7826=CARTESIAN_POINT('Ctrl Pts',(6.73914381348523,9.09860577342165,6.));
#7827=CARTESIAN_POINT('Ctrl Pts',(6.73297955932548,9.16385288053588,6.));
#7828=CARTESIAN_POINT('Ctrl Pts',(6.72623333926846,9.22922952332026,6.));
#7829=CARTESIAN_POINT('Ctrl Pts',(6.71890629646187,9.2947306015555,6.));
#7830=CARTESIAN_POINT('Ctrl Pts',(6.71099953007124,9.36035072031876,6.));
#7831=CARTESIAN_POINT('Ctrl Pts',(6.70251410760819,9.42608392519666,6.));
#7832=CARTESIAN_POINT('Ctrl Pts',(6.69345108162377,9.49192378686253,6.));
#7833=CARTESIAN_POINT('Ctrl Pts',(6.68381150859182,9.55786385494286,6.));
#7834=CARTESIAN_POINT('Ctrl Pts',(6.67359647366961,9.62389802250188,6.));
#7835=CARTESIAN_POINT('Ctrl Pts',(6.66280711160719,9.69002090483258,6.));
#7836=CARTESIAN_POINT('Ctrl Pts',(6.65144464725859,9.75622826411013,6.));
#7837=CARTESIAN_POINT('Ctrl Pts',(6.63951038900667,9.82251725114898,6.));
#7838=CARTESIAN_POINT('Ctrl Pts',(6.62700557693596,9.88888607996273,6.));
#7839=CARTESIAN_POINT('Ctrl Pts',(6.61654612354183,9.94204425953052,6.));
#7840=CARTESIAN_POINT('Ctrl Pts',(6.60844558393656,9.98194823089968,6.));
#7841=CARTESIAN_POINT('Ctrl Pts',(6.60293150665659,10.0085665785717,6.));
#7842=CARTESIAN_POINT('Ctrl Pts',(6.60014603862877,10.0218796774244,6.));
#7843=CARTESIAN_POINT('Origin',(0.,0.,-1.));
#7844=CARTESIAN_POINT('Origin',(0.,0.,-1.));
#7845=CARTESIAN_POINT('Origin',(0.,0.,-1.));
#7846=CARTESIAN_POINT('Origin',(0.,0.,-1.));
#7847=CARTESIAN_POINT('',(5.02458355455784,2.3072496837722,-1.));
#7848=CARTESIAN_POINT('Origin',(0.,0.,-1.));
#7849=CARTESIAN_POINT('',(6.20653880480254,1.76258817211517,-1.));
#7850=CARTESIAN_POINT('Origin',(5.93335250998519,2.72454931910811,-1.));
#7851=CARTESIAN_POINT('',(8.13553012180811,2.31040030805735,-1.));
#7852=CARTESIAN_POINT('',(4.06776506090406,1.15520015402867,-1.));
#7853=CARTESIAN_POINT('',(11.9792754136349,0.704954299427496,-1.));
#7854=CARTESIAN_POINT('Ctrl Pts',(11.9792754136349,0.704954299427529,-1.));
#7855=CARTESIAN_POINT('Ctrl Pts',(11.9691386658393,0.714023134927411,-1.));
#7856=CARTESIAN_POINT('Ctrl Pts',(11.9488435391885,0.73210763976631,-1.));
#7857=CARTESIAN_POINT('Ctrl Pts',(11.9183359560736,0.759074898533419,-1.));
#7858=CARTESIAN_POINT('Ctrl Pts',(11.877529348846,0.794712140666325,-1.));
#7859=CARTESIAN_POINT('Ctrl Pts',(11.8263046631092,0.838726039995982,-1.));
#7860=CARTESIAN_POINT('Ctrl Pts',(11.7748638454684,0.882205904336896,-1.));
#7861=CARTESIAN_POINT('Ctrl Pts',(11.7232078225909,0.925149766751161,-1.));
#7862=CARTESIAN_POINT('Ctrl Pts',(11.6713384077523,0.967555069553193,-1.));
#7863=CARTESIAN_POINT('Ctrl Pts',(11.6192586585895,1.00941863307588,-1.));
#7864=CARTESIAN_POINT('Ctrl Pts',(11.5669726710206,1.05073678224334,-1.));
#7865=CARTESIAN_POINT('Ctrl Pts',(11.5144851912285,1.09150552381395,-1.));
#7866=CARTESIAN_POINT('Ctrl Pts',(11.4618012771636,1.13172071766774,-1.));
#7867=CARTESIAN_POINT('Ctrl Pts',(11.4089259705106,1.17137823760545,-1.));
#7868=CARTESIAN_POINT('Ctrl Pts',(11.3558638941869,1.21047418192819,-1.));
#7869=CARTESIAN_POINT('Ctrl Pts',(11.30261917075,1.24900490126928,-1.));
#7870=CARTESIAN_POINT('Ctrl Pts',(11.2491956455455,1.28696685552412,-1.));
#7871=CARTESIAN_POINT('Ctrl Pts',(11.1955970312291,1.32435651843207,-1.));
#7872=CARTESIAN_POINT('Ctrl Pts',(11.1418270749817,1.36117027439398,-1.));
#7873=CARTESIAN_POINT('Ctrl Pts',(11.0878897426906,1.39740430473756,-1.));
#7874=CARTESIAN_POINT('Ctrl Pts',(11.033789312906,1.43305454241432,-1.));
#7875=CARTESIAN_POINT('Ctrl Pts',(10.9795302662584,1.46811677324654,-1.));
#7876=CARTESIAN_POINT('Ctrl Pts',(10.9251172180581,1.50258671261028,-1.));
#7877=CARTESIAN_POINT('Ctrl Pts',(10.8705548380775,1.53646008988796,-1.));
#7878=CARTESIAN_POINT('Ctrl Pts',(10.8158477697972,1.56973274862052,-1.));
#7879=CARTESIAN_POINT('Ctrl Pts',(10.761000572936,1.60240070038749,-1.));
#7880=CARTESIAN_POINT('Ctrl Pts',(10.7060177866027,1.63445994423348,-1.));
#7881=CARTESIAN_POINT('Ctrl Pts',(10.6509039769739,1.66590631967585,-1.));
#7882=CARTESIAN_POINT('Ctrl Pts',(10.59566379085,1.69673535547184,-1.));
#7883=CARTESIAN_POINT('Ctrl Pts',(10.5403020105194,1.72694211360792,-1.));
#7884=CARTESIAN_POINT('Ctrl Pts',(10.4848236013528,1.75652107004318,-1.));
#7885=CARTESIAN_POINT('Ctrl Pts',(10.4292336483793,1.78546643461776,-1.));
#7886=CARTESIAN_POINT('Ctrl Pts',(10.3735373011506,1.81377244526718,-1.));
#7887=CARTESIAN_POINT('Ctrl Pts',(10.317739716759,1.84143367405762,-1.));
#7888=CARTESIAN_POINT('Ctrl Pts',(10.2618460035706,1.86844533887956,-1.));
#7889=CARTESIAN_POINT('Ctrl Pts',(10.2058611678956,1.89480360265125,-1.));
#7890=CARTESIAN_POINT('Ctrl Pts',(10.1497902344364,1.92050480406378,-1.));
#7891=CARTESIAN_POINT('Ctrl Pts',(10.0936383641523,1.94554471072257,-1.));
#7892=CARTESIAN_POINT('Ctrl Pts',(10.037410974034,1.96991776698621,-1.));
#7893=CARTESIAN_POINT('Ctrl Pts',(9.98111385659409,1.99361634997092,-1.));
#7894=CARTESIAN_POINT('Ctrl Pts',(9.92475330165988,2.01663001707736,-1.));
#7895=CARTESIAN_POINT('Ctrl Pts',(9.86833584478527,2.03894719582859,-1.));
#7896=CARTESIAN_POINT('Ctrl Pts',(9.81186801391803,2.06055689146528,-1.));
#7897=CARTESIAN_POINT('Ctrl Pts',(9.75535607889871,2.08145038176732,-1.));
#7898=CARTESIAN_POINT('Ctrl Pts',(9.69880579601398,2.10162295100989,-1.));
#7899=CARTESIAN_POINT('Ctrl Pts',(9.64222216484242,2.12107554726937,-1.));
#7900=CARTESIAN_POINT('Ctrl Pts',(9.58561005875903,2.13981058538587,-1.));
#7901=CARTESIAN_POINT('Ctrl Pts',(9.52897485563506,2.15782775391113,-1.));
#7902=CARTESIAN_POINT('Ctrl Pts',(9.4723230488593,2.17511995998945,-1.));
#7903=CARTESIAN_POINT('Ctrl Pts',(9.41566291502215,2.19166889809876,-1.));
#7904=CARTESIAN_POINT('Ctrl Pts',(9.35900502856467,2.2074416540289,-1.));
#7905=CARTESIAN_POINT('Ctrl Pts',(9.30236077039477,2.22240082168223,-1.));
#7906=CARTESIAN_POINT('Ctrl Pts',(9.24574089753053,2.23651421201962,-1.));
#7907=CARTESIAN_POINT('Ctrl Pts',(9.18915420809356,2.24976392906278,-1.));
#7908=CARTESIAN_POINT('Ctrl Pts',(9.13260588645235,2.26215759393014,-1.));
#7909=CARTESIAN_POINT('Ctrl Pts',(9.07609679780011,2.27373321015996,-1.));
#7910=CARTESIAN_POINT('Ctrl Pts',(9.0196273647496,2.28453333318601,-1.));
#7911=CARTESIAN_POINT('Ctrl Pts',(8.96320109950669,2.29458154408801,-1.));
#7912=CARTESIAN_POINT('Ctrl Pts',(8.90682777405608,2.30386137247017,-1.));
#7913=CARTESIAN_POINT('Ctrl Pts',(8.85052793120604,2.31228619203479,-1.));
#7914=CARTESIAN_POINT('Ctrl Pts',(8.79433301721166,2.31969862084206,-1.));
#7915=CARTESIAN_POINT('Ctrl Pts',(8.73827625692193,2.32593252219559,-1.));
#7916=CARTESIAN_POINT('Ctrl Pts',(8.68238458286971,2.33086762045752,-1.));
#7917=CARTESIAN_POINT('Ctrl Pts',(8.62667187892838,2.33447589689188,-1.));
#7918=CARTESIAN_POINT('Ctrl Pts',(8.57112741281372,2.33689888190034,-1.));
#7919=CARTESIAN_POINT('Ctrl Pts',(8.51572283259063,2.33840535058003,-1.));
#7920=CARTESIAN_POINT('Ctrl Pts',(8.46043689627596,2.3392342622836,-1.));
#7921=CARTESIAN_POINT('Ctrl Pts',(8.40527692606173,2.339459611751,-1.));
#7922=CARTESIAN_POINT('Ctrl Pts',(8.35029826768635,2.33886640526141,-1.));
#7923=CARTESIAN_POINT('Ctrl Pts',(8.29563322262997,2.33676998946178,-1.));
#7924=CARTESIAN_POINT('Ctrl Pts',(8.24146380440172,2.33217339857873,-1.));
#7925=CARTESIAN_POINT('Ctrl Pts',(8.19867202257947,2.32567282066755,-1.));
#7926=CARTESIAN_POINT('Ctrl Pts',(8.16694940973767,2.31883955953704,-1.));
#7927=CARTESIAN_POINT('Ctrl Pts',(8.14597432907962,2.31336634706602,-1.));
#7928=CARTESIAN_POINT('Ctrl Pts',(8.13553012180811,2.31040030805735,-1.));
#7929=CARTESIAN_POINT('',(11.9792754136349,-0.704954299427528,-1.));
#7930=CARTESIAN_POINT('Origin',(3.99680288865056E-13,0.,-1.));
#7931=CARTESIAN_POINT('',(8.13553012180811,-2.31040030805735,-1.));
#7932=CARTESIAN_POINT('Ctrl Pts',(8.13553012180811,-2.31040030805735,-1.));
#7933=CARTESIAN_POINT('Ctrl Pts',(8.14597432907962,-2.31336634706602,-1.));
#7934=CARTESIAN_POINT('Ctrl Pts',(8.16694940973767,-2.31883955953704,-1.));
#7935=CARTESIAN_POINT('Ctrl Pts',(8.19867202257947,-2.32567282066755,-1.));
#7936=CARTESIAN_POINT('Ctrl Pts',(8.24146380440172,-2.33217339857873,-1.));
#7937=CARTESIAN_POINT('Ctrl Pts',(8.29563322262997,-2.33676998946178,-1.));
#7938=CARTESIAN_POINT('Ctrl Pts',(8.35029826768635,-2.33886640526141,-1.));
#7939=CARTESIAN_POINT('Ctrl Pts',(8.40527692606173,-2.339459611751,-1.));
#7940=CARTESIAN_POINT('Ctrl Pts',(8.46043689627596,-2.3392342622836,-1.));
#7941=CARTESIAN_POINT('Ctrl Pts',(8.51572283259063,-2.33840535058003,-1.));
#7942=CARTESIAN_POINT('Ctrl Pts',(8.57112741281372,-2.33689888190034,-1.));
#7943=CARTESIAN_POINT('Ctrl Pts',(8.62667187892838,-2.33447589689188,-1.));
#7944=CARTESIAN_POINT('Ctrl Pts',(8.68238458286971,-2.33086762045752,-1.));
#7945=CARTESIAN_POINT('Ctrl Pts',(8.73827625692193,-2.32593252219559,-1.));
#7946=CARTESIAN_POINT('Ctrl Pts',(8.79433301721166,-2.31969862084206,-1.));
#7947=CARTESIAN_POINT('Ctrl Pts',(8.85052793120604,-2.31228619203479,-1.));
#7948=CARTESIAN_POINT('Ctrl Pts',(8.90682777405608,-2.30386137247017,-1.));
#7949=CARTESIAN_POINT('Ctrl Pts',(8.96320109950669,-2.29458154408801,-1.));
#7950=CARTESIAN_POINT('Ctrl Pts',(9.0196273647496,-2.28453333318601,-1.));
#7951=CARTESIAN_POINT('Ctrl Pts',(9.07609679780011,-2.27373321015996,-1.));
#7952=CARTESIAN_POINT('Ctrl Pts',(9.13260588645235,-2.26215759393014,-1.));
#7953=CARTESIAN_POINT('Ctrl Pts',(9.18915420809356,-2.24976392906278,-1.));
#7954=CARTESIAN_POINT('Ctrl Pts',(9.24574089753053,-2.23651421201962,-1.));
#7955=CARTESIAN_POINT('Ctrl Pts',(9.30236077039477,-2.22240082168223,-1.));
#7956=CARTESIAN_POINT('Ctrl Pts',(9.35900502856467,-2.2074416540289,-1.));
#7957=CARTESIAN_POINT('Ctrl Pts',(9.41566291502215,-2.19166889809876,-1.));
#7958=CARTESIAN_POINT('Ctrl Pts',(9.4723230488593,-2.17511995998945,-1.));
#7959=CARTESIAN_POINT('Ctrl Pts',(9.52897485563506,-2.15782775391113,-1.));
#7960=CARTESIAN_POINT('Ctrl Pts',(9.58561005875903,-2.13981058538587,-1.));
#7961=CARTESIAN_POINT('Ctrl Pts',(9.64222216484242,-2.12107554726937,-1.));
#7962=CARTESIAN_POINT('Ctrl Pts',(9.69880579601398,-2.10162295100989,-1.));
#7963=CARTESIAN_POINT('Ctrl Pts',(9.75535607889871,-2.08145038176732,-1.));
#7964=CARTESIAN_POINT('Ctrl Pts',(9.81186801391803,-2.06055689146528,-1.));
#7965=CARTESIAN_POINT('Ctrl Pts',(9.86833584478527,-2.03894719582859,-1.));
#7966=CARTESIAN_POINT('Ctrl Pts',(9.92475330165988,-2.01663001707736,-1.));
#7967=CARTESIAN_POINT('Ctrl Pts',(9.98111385659409,-1.99361634997092,-1.));
#7968=CARTESIAN_POINT('Ctrl Pts',(10.037410974034,-1.96991776698621,-1.));
#7969=CARTESIAN_POINT('Ctrl Pts',(10.0936383641523,-1.94554471072257,-1.));
#7970=CARTESIAN_POINT('Ctrl Pts',(10.1497902344364,-1.92050480406378,-1.));
#7971=CARTESIAN_POINT('Ctrl Pts',(10.2058611678956,-1.89480360265125,-1.));
#7972=CARTESIAN_POINT('Ctrl Pts',(10.2618460035706,-1.86844533887956,-1.));
#7973=CARTESIAN_POINT('Ctrl Pts',(10.317739716759,-1.84143367405762,-1.));
#7974=CARTESIAN_POINT('Ctrl Pts',(10.3735373011506,-1.81377244526718,-1.));
#7975=CARTESIAN_POINT('Ctrl Pts',(10.4292336483793,-1.78546643461776,-1.));
#7976=CARTESIAN_POINT('Ctrl Pts',(10.4848236013528,-1.75652107004318,-1.));
#7977=CARTESIAN_POINT('Ctrl Pts',(10.5403020105194,-1.72694211360792,-1.));
#7978=CARTESIAN_POINT('Ctrl Pts',(10.59566379085,-1.69673535547184,-1.));
#7979=CARTESIAN_POINT('Ctrl Pts',(10.6509039769739,-1.66590631967585,-1.));
#7980=CARTESIAN_POINT('Ctrl Pts',(10.7060177866027,-1.63445994423348,-1.));
#7981=CARTESIAN_POINT('Ctrl Pts',(10.761000572936,-1.60240070038749,-1.));
#7982=CARTESIAN_POINT('Ctrl Pts',(10.8158477697972,-1.56973274862052,-1.));
#7983=CARTESIAN_POINT('Ctrl Pts',(10.8705548380775,-1.53646008988796,-1.));
#7984=CARTESIAN_POINT('Ctrl Pts',(10.9251172180581,-1.50258671261028,-1.));
#7985=CARTESIAN_POINT('Ctrl Pts',(10.9795302662584,-1.46811677324654,-1.));
#7986=CARTESIAN_POINT('Ctrl Pts',(11.033789312906,-1.43305454241432,-1.));
#7987=CARTESIAN_POINT('Ctrl Pts',(11.0878897426906,-1.39740430473756,-1.));
#7988=CARTESIAN_POINT('Ctrl Pts',(11.1418270749817,-1.36117027439398,-1.));
#7989=CARTESIAN_POINT('Ctrl Pts',(11.1955970312291,-1.32435651843207,-1.));
#7990=CARTESIAN_POINT('Ctrl Pts',(11.2491956455455,-1.28696685552412,-1.));
#7991=CARTESIAN_POINT('Ctrl Pts',(11.30261917075,-1.24900490126928,-1.));
#7992=CARTESIAN_POINT('Ctrl Pts',(11.3558638941869,-1.21047418192819,-1.));
#7993=CARTESIAN_POINT('Ctrl Pts',(11.4089259705106,-1.17137823760545,-1.));
#7994=CARTESIAN_POINT('Ctrl Pts',(11.4618012771636,-1.13172071766774,-1.));
#7995=CARTESIAN_POINT('Ctrl Pts',(11.5144851912285,-1.09150552381395,-1.));
#7996=CARTESIAN_POINT('Ctrl Pts',(11.5669726710206,-1.05073678224334,-1.));
#7997=CARTESIAN_POINT('Ctrl Pts',(11.6192586585895,-1.00941863307588,-1.));
#7998=CARTESIAN_POINT('Ctrl Pts',(11.6713384077523,-0.967555069553193,-1.));
#7999=CARTESIAN_POINT('Ctrl Pts',(11.7232078225909,-0.925149766751161,-1.));
#8000=CARTESIAN_POINT('Ctrl Pts',(11.7748638454684,-0.882205904336896,-1.));
#8001=CARTESIAN_POINT('Ctrl Pts',(11.8263046631092,-0.838726039995982,-1.));
#8002=CARTESIAN_POINT('Ctrl Pts',(11.877529348846,-0.794712140666325,-1.));
#8003=CARTESIAN_POINT('Ctrl Pts',(11.9183359560736,-0.759074898533419,-1.));
#8004=CARTESIAN_POINT('Ctrl Pts',(11.9488435391885,-0.73210763976631,-1.));
#8005=CARTESIAN_POINT('Ctrl Pts',(11.9691386658393,-0.714023134927411,-1.));
#8006=CARTESIAN_POINT('Ctrl Pts',(11.9792754136349,-0.704954299427529,-1.));
#8007=CARTESIAN_POINT('',(6.20653880480254,-1.76258817211517,-1.));
#8008=CARTESIAN_POINT('',(2.65453178512701,-0.75385758054847,-1.));
#8009=CARTESIAN_POINT('',(5.02458355455784,-2.3072496837722,-1.));
#8010=CARTESIAN_POINT('Origin',(5.93335250998519,-2.72454931910811,-1.));
#8011=CARTESIAN_POINT('Origin',(0.,0.,-1.));
#8012=CARTESIAN_POINT('Origin',(0.,0.,-1.));
#8013=CARTESIAN_POINT('',(-5.,6.12323399573677E-16,-1.));
#8014=CARTESIAN_POINT('Origin',(0.,0.,-1.));
#8015=CARTESIAN_POINT('Origin',(0.,0.,0.));
#8016=CARTESIAN_POINT('',(5.02458355455784,2.3072496837722,6.));
#8017=CARTESIAN_POINT('Origin',(0.,0.,6.));
#8018=CARTESIAN_POINT('',(5.02458355455784,2.3072496837722,0.));
#8019=CARTESIAN_POINT('Origin',(0.,0.,0.));
#8020=CARTESIAN_POINT('Origin',(0.,0.,6.));
#8021=CARTESIAN_POINT('Origin',(0.,0.,0.));
#8022=CARTESIAN_POINT('Origin',(0.,0.,6.));
#8023=CARTESIAN_POINT('Origin',(0.,0.,0.));
#8024=CARTESIAN_POINT('Origin',(0.,0.,6.));
#8025=CARTESIAN_POINT('Origin',(0.,0.,0.));
#8026=CARTESIAN_POINT('Origin',(0.,0.,6.));
#8027=CARTESIAN_POINT('Origin',(5.93335250998519,2.72454931910811,0.));
#8028=CARTESIAN_POINT('',(6.20653880480254,1.76258817211517,6.));
#8029=CARTESIAN_POINT('Origin',(5.93335250998519,2.72454931910811,6.));
#8030=CARTESIAN_POINT('',(6.20653880480254,1.76258817211517,0.));
#8031=CARTESIAN_POINT('Origin',(8.13553012180811,2.31040030805735,0.));
#8032=CARTESIAN_POINT('',(8.13553012180811,2.31040030805735,6.));
#8033=CARTESIAN_POINT('',(4.06776506090406,1.15520015402867,6.));
#8034=CARTESIAN_POINT('',(8.13553012180811,2.31040030805735,0.));
#8035=CARTESIAN_POINT('Origin',(5.93335250998519,-2.72454931910811,0.));
#8036=CARTESIAN_POINT('',(6.20653880480254,-1.76258817211517,6.));
#8037=CARTESIAN_POINT('',(6.20653880480254,-1.76258817211517,0.));
#8038=CARTESIAN_POINT('',(5.02458355455784,-2.3072496837722,6.));
#8039=CARTESIAN_POINT('Origin',(5.93335250998519,-2.72454931910811,6.));
#8040=CARTESIAN_POINT('',(5.02458355455784,-2.3072496837722,0.));
#8041=CARTESIAN_POINT('Origin',(5.30906357025403,-1.50771516109694,0.));
#8042=CARTESIAN_POINT('',(8.13553012180811,-2.31040030805735,6.));
#8043=CARTESIAN_POINT('',(8.13553012180811,-2.31040030805735,0.));
#8044=CARTESIAN_POINT('',(2.65453178512701,-0.75385758054847,6.));
#8045=CARTESIAN_POINT('Ctrl Pts',(11.9792754136349,0.704954299427529,-3.75));
#8046=CARTESIAN_POINT('Ctrl Pts',(11.9792754136349,0.704954299427529,12.75));
#8047=CARTESIAN_POINT('Ctrl Pts',(11.9691386658393,0.714023134927411,-3.75));
#8048=CARTESIAN_POINT('Ctrl Pts',(11.9691386658393,0.714023134927411,12.75));
#8049=CARTESIAN_POINT('Ctrl Pts',(11.9488435391885,0.73210763976631,-3.75));
#8050=CARTESIAN_POINT('Ctrl Pts',(11.9488435391885,0.73210763976631,12.75));
#8051=CARTESIAN_POINT('Ctrl Pts',(11.9183359560736,0.759074898533419,-3.75));
#8052=CARTESIAN_POINT('Ctrl Pts',(11.9183359560736,0.759074898533419,12.75));
#8053=CARTESIAN_POINT('Ctrl Pts',(11.877529348846,0.794712140666325,-3.75));
#8054=CARTESIAN_POINT('Ctrl Pts',(11.877529348846,0.794712140666325,12.75));
#8055=CARTESIAN_POINT('Ctrl Pts',(11.8263046631092,0.838726039995982,-3.75));
#8056=CARTESIAN_POINT('Ctrl Pts',(11.8263046631092,0.838726039995982,12.75));
#8057=CARTESIAN_POINT('Ctrl Pts',(11.7748638454684,0.882205904336896,-3.75));
#8058=CARTESIAN_POINT('Ctrl Pts',(11.7748638454684,0.882205904336896,12.75));
#8059=CARTESIAN_POINT('Ctrl Pts',(11.7232078225909,0.925149766751161,-3.75));
#8060=CARTESIAN_POINT('Ctrl Pts',(11.7232078225909,0.925149766751161,12.75));
#8061=CARTESIAN_POINT('Ctrl Pts',(11.6713384077523,0.967555069553193,-3.75));
#8062=CARTESIAN_POINT('Ctrl Pts',(11.6713384077523,0.967555069553193,12.75));
#8063=CARTESIAN_POINT('Ctrl Pts',(11.6192586585895,1.00941863307588,-3.75));
#8064=CARTESIAN_POINT('Ctrl Pts',(11.6192586585895,1.00941863307588,12.75));
#8065=CARTESIAN_POINT('Ctrl Pts',(11.5669726710206,1.05073678224334,-3.75));
#8066=CARTESIAN_POINT('Ctrl Pts',(11.5669726710206,1.05073678224334,12.75));
#8067=CARTESIAN_POINT('Ctrl Pts',(11.5144851912285,1.09150552381395,-3.75));
#8068=CARTESIAN_POINT('Ctrl Pts',(11.5144851912285,1.09150552381395,12.75));
#8069=CARTESIAN_POINT('Ctrl Pts',(11.4618012771636,1.13172071766774,-3.75));
#8070=CARTESIAN_POINT('Ctrl Pts',(11.4618012771636,1.13172071766774,12.75));
#8071=CARTESIAN_POINT('Ctrl Pts',(11.4089259705106,1.17137823760545,-3.75));
#8072=CARTESIAN_POINT('Ctrl Pts',(11.4089259705106,1.17137823760545,12.75));
#8073=CARTESIAN_POINT('Ctrl Pts',(11.3558638941869,1.21047418192819,-3.75));
#8074=CARTESIAN_POINT('Ctrl Pts',(11.3558638941869,1.21047418192819,12.75));
#8075=CARTESIAN_POINT('Ctrl Pts',(11.30261917075,1.24900490126928,-3.75));
#8076=CARTESIAN_POINT('Ctrl Pts',(11.30261917075,1.24900490126928,12.75));
#8077=CARTESIAN_POINT('Ctrl Pts',(11.2491956455455,1.28696685552412,-3.75));
#8078=CARTESIAN_POINT('Ctrl Pts',(11.2491956455455,1.28696685552412,12.75));
#8079=CARTESIAN_POINT('Ctrl Pts',(11.1955970312291,1.32435651843207,-3.75));
#8080=CARTESIAN_POINT('Ctrl Pts',(11.1955970312291,1.32435651843207,12.75));
#8081=CARTESIAN_POINT('Ctrl Pts',(11.1418270749817,1.36117027439398,-3.75));
#8082=CARTESIAN_POINT('Ctrl Pts',(11.1418270749817,1.36117027439398,12.75));
#8083=CARTESIAN_POINT('Ctrl Pts',(11.0878897426906,1.39740430473756,-3.75));
#8084=CARTESIAN_POINT('Ctrl Pts',(11.0878897426906,1.39740430473756,12.75));
#8085=CARTESIAN_POINT('Ctrl Pts',(11.033789312906,1.43305454241432,-3.75));
#8086=CARTESIAN_POINT('Ctrl Pts',(11.033789312906,1.43305454241432,12.75));
#8087=CARTESIAN_POINT('Ctrl Pts',(10.9795302662584,1.46811677324654,-3.75));
#8088=CARTESIAN_POINT('Ctrl Pts',(10.9795302662584,1.46811677324654,12.75));
#8089=CARTESIAN_POINT('Ctrl Pts',(10.9251172180581,1.50258671261028,-3.75));
#8090=CARTESIAN_POINT('Ctrl Pts',(10.9251172180581,1.50258671261028,12.75));
#8091=CARTESIAN_POINT('Ctrl Pts',(10.8705548380775,1.53646008988796,-3.75));
#8092=CARTESIAN_POINT('Ctrl Pts',(10.8705548380775,1.53646008988796,12.75));
#8093=CARTESIAN_POINT('Ctrl Pts',(10.8158477697972,1.56973274862052,-3.75));
#8094=CARTESIAN_POINT('Ctrl Pts',(10.8158477697972,1.56973274862052,12.75));
#8095=CARTESIAN_POINT('Ctrl Pts',(10.761000572936,1.60240070038749,-3.75));
#8096=CARTESIAN_POINT('Ctrl Pts',(10.761000572936,1.60240070038749,12.75));
#8097=CARTESIAN_POINT('Ctrl Pts',(10.7060177866027,1.63445994423348,-3.75));
#8098=CARTESIAN_POINT('Ctrl Pts',(10.7060177866027,1.63445994423348,12.75));
#8099=CARTESIAN_POINT('Ctrl Pts',(10.6509039769739,1.66590631967585,-3.75));
#8100=CARTESIAN_POINT('Ctrl Pts',(10.6509039769739,1.66590631967585,12.75));
#8101=CARTESIAN_POINT('Ctrl Pts',(10.59566379085,1.69673535547184,-3.75));
#8102=CARTESIAN_POINT('Ctrl Pts',(10.59566379085,1.69673535547184,12.75));
#8103=CARTESIAN_POINT('Ctrl Pts',(10.5403020105194,1.72694211360792,-3.75));
#8104=CARTESIAN_POINT('Ctrl Pts',(10.5403020105194,1.72694211360792,12.75));
#8105=CARTESIAN_POINT('Ctrl Pts',(10.4848236013528,1.75652107004318,-3.75));
#8106=CARTESIAN_POINT('Ctrl Pts',(10.4848236013528,1.75652107004318,12.75));
#8107=CARTESIAN_POINT('Ctrl Pts',(10.4292336483793,1.78546643461776,-3.75));
#8108=CARTESIAN_POINT('Ctrl Pts',(10.4292336483793,1.78546643461776,12.75));
#8109=CARTESIAN_POINT('Ctrl Pts',(10.3735373011506,1.81377244526718,-3.75));
#8110=CARTESIAN_POINT('Ctrl Pts',(10.3735373011506,1.81377244526718,12.75));
#8111=CARTESIAN_POINT('Ctrl Pts',(10.317739716759,1.84143367405762,-3.75));
#8112=CARTESIAN_POINT('Ctrl Pts',(10.317739716759,1.84143367405762,12.75));
#8113=CARTESIAN_POINT('Ctrl Pts',(10.2618460035706,1.86844533887956,-3.75));
#8114=CARTESIAN_POINT('Ctrl Pts',(10.2618460035706,1.86844533887956,12.75));
#8115=CARTESIAN_POINT('Ctrl Pts',(10.2058611678956,1.89480360265125,-3.75));
#8116=CARTESIAN_POINT('Ctrl Pts',(10.2058611678956,1.89480360265125,12.75));
#8117=CARTESIAN_POINT('Ctrl Pts',(10.1497902344364,1.92050480406378,-3.75));
#8118=CARTESIAN_POINT('Ctrl Pts',(10.1497902344364,1.92050480406378,12.75));
#8119=CARTESIAN_POINT('Ctrl Pts',(10.0936383641523,1.94554471072257,-3.75));
#8120=CARTESIAN_POINT('Ctrl Pts',(10.0936383641523,1.94554471072257,12.75));
#8121=CARTESIAN_POINT('Ctrl Pts',(10.037410974034,1.96991776698621,-3.75));
#8122=CARTESIAN_POINT('Ctrl Pts',(10.037410974034,1.96991776698621,12.75));
#8123=CARTESIAN_POINT('Ctrl Pts',(9.98111385659409,1.99361634997092,-3.75));
#8124=CARTESIAN_POINT('Ctrl Pts',(9.98111385659409,1.99361634997092,12.75));
#8125=CARTESIAN_POINT('Ctrl Pts',(9.92475330165988,2.01663001707736,-3.75));
#8126=CARTESIAN_POINT('Ctrl Pts',(9.92475330165988,2.01663001707736,12.75));
#8127=CARTESIAN_POINT('Ctrl Pts',(9.86833584478527,2.03894719582859,-3.75));
#8128=CARTESIAN_POINT('Ctrl Pts',(9.86833584478527,2.03894719582859,12.75));
#8129=CARTESIAN_POINT('Ctrl Pts',(9.81186801391803,2.06055689146528,-3.75));
#8130=CARTESIAN_POINT('Ctrl Pts',(9.81186801391803,2.06055689146528,12.75));
#8131=CARTESIAN_POINT('Ctrl Pts',(9.75535607889871,2.08145038176732,-3.75));
#8132=CARTESIAN_POINT('Ctrl Pts',(9.75535607889871,2.08145038176732,12.75));
#8133=CARTESIAN_POINT('Ctrl Pts',(9.69880579601398,2.10162295100989,-3.75));
#8134=CARTESIAN_POINT('Ctrl Pts',(9.69880579601398,2.10162295100989,12.75));
#8135=CARTESIAN_POINT('Ctrl Pts',(9.64222216484242,2.12107554726937,-3.75));
#8136=CARTESIAN_POINT('Ctrl Pts',(9.64222216484242,2.12107554726937,12.75));
#8137=CARTESIAN_POINT('Ctrl Pts',(9.58561005875903,2.13981058538587,-3.75));
#8138=CARTESIAN_POINT('Ctrl Pts',(9.58561005875903,2.13981058538587,12.75));
#8139=CARTESIAN_POINT('Ctrl Pts',(9.52897485563506,2.15782775391113,-3.75));
#8140=CARTESIAN_POINT('Ctrl Pts',(9.52897485563506,2.15782775391113,12.75));
#8141=CARTESIAN_POINT('Ctrl Pts',(9.4723230488593,2.17511995998945,-3.75));
#8142=CARTESIAN_POINT('Ctrl Pts',(9.4723230488593,2.17511995998945,12.75));
#8143=CARTESIAN_POINT('Ctrl Pts',(9.41566291502215,2.19166889809876,-3.75));
#8144=CARTESIAN_POINT('Ctrl Pts',(9.41566291502215,2.19166889809876,12.75));
#8145=CARTESIAN_POINT('Ctrl Pts',(9.35900502856467,2.2074416540289,-3.75));
#8146=CARTESIAN_POINT('Ctrl Pts',(9.35900502856467,2.2074416540289,12.75));
#8147=CARTESIAN_POINT('Ctrl Pts',(9.30236077039477,2.22240082168223,-3.75));
#8148=CARTESIAN_POINT('Ctrl Pts',(9.30236077039477,2.22240082168223,12.75));
#8149=CARTESIAN_POINT('Ctrl Pts',(9.24574089753053,2.23651421201962,-3.75));
#8150=CARTESIAN_POINT('Ctrl Pts',(9.24574089753053,2.23651421201962,12.75));
#8151=CARTESIAN_POINT('Ctrl Pts',(9.18915420809356,2.24976392906278,-3.75));
#8152=CARTESIAN_POINT('Ctrl Pts',(9.18915420809356,2.24976392906278,12.75));
#8153=CARTESIAN_POINT('Ctrl Pts',(9.13260588645235,2.26215759393014,-3.75));
#8154=CARTESIAN_POINT('Ctrl Pts',(9.13260588645235,2.26215759393014,12.75));
#8155=CARTESIAN_POINT('Ctrl Pts',(9.07609679780011,2.27373321015996,-3.75));
#8156=CARTESIAN_POINT('Ctrl Pts',(9.07609679780011,2.27373321015996,12.75));
#8157=CARTESIAN_POINT('Ctrl Pts',(9.0196273647496,2.28453333318601,-3.75));
#8158=CARTESIAN_POINT('Ctrl Pts',(9.0196273647496,2.28453333318601,12.75));
#8159=CARTESIAN_POINT('Ctrl Pts',(8.96320109950669,2.29458154408801,-3.75));
#8160=CARTESIAN_POINT('Ctrl Pts',(8.96320109950669,2.29458154408801,12.75));
#8161=CARTESIAN_POINT('Ctrl Pts',(8.90682777405608,2.30386137247017,-3.75));
#8162=CARTESIAN_POINT('Ctrl Pts',(8.90682777405608,2.30386137247017,12.75));
#8163=CARTESIAN_POINT('Ctrl Pts',(8.85052793120604,2.31228619203479,-3.75));
#8164=CARTESIAN_POINT('Ctrl Pts',(8.85052793120604,2.31228619203479,12.75));
#8165=CARTESIAN_POINT('Ctrl Pts',(8.79433301721166,2.31969862084206,-3.75));
#8166=CARTESIAN_POINT('Ctrl Pts',(8.79433301721166,2.31969862084206,12.75));
#8167=CARTESIAN_POINT('Ctrl Pts',(8.73827625692193,2.32593252219559,-3.75));
#8168=CARTESIAN_POINT('Ctrl Pts',(8.73827625692193,2.32593252219559,12.75));
#8169=CARTESIAN_POINT('Ctrl Pts',(8.68238458286971,2.33086762045752,-3.75));
#8170=CARTESIAN_POINT('Ctrl Pts',(8.68238458286971,2.33086762045752,12.75));
#8171=CARTESIAN_POINT('Ctrl Pts',(8.62667187892838,2.33447589689188,-3.75));
#8172=CARTESIAN_POINT('Ctrl Pts',(8.62667187892838,2.33447589689188,12.75));
#8173=CARTESIAN_POINT('Ctrl Pts',(8.57112741281372,2.33689888190034,-3.75));
#8174=CARTESIAN_POINT('Ctrl Pts',(8.57112741281372,2.33689888190034,12.75));
#8175=CARTESIAN_POINT('Ctrl Pts',(8.51572283259063,2.33840535058003,-3.75));
#8176=CARTESIAN_POINT('Ctrl Pts',(8.51572283259063,2.33840535058003,12.75));
#8177=CARTESIAN_POINT('Ctrl Pts',(8.46043689627596,2.3392342622836,-3.75));
#8178=CARTESIAN_POINT('Ctrl Pts',(8.46043689627596,2.3392342622836,12.75));
#8179=CARTESIAN_POINT('Ctrl Pts',(8.40527692606173,2.339459611751,-3.75));
#8180=CARTESIAN_POINT('Ctrl Pts',(8.40527692606173,2.339459611751,12.75));
#8181=CARTESIAN_POINT('Ctrl Pts',(8.35029826768635,2.33886640526141,-3.75));
#8182=CARTESIAN_POINT('Ctrl Pts',(8.35029826768635,2.33886640526141,12.75));
#8183=CARTESIAN_POINT('Ctrl Pts',(8.29563322262997,2.33676998946178,-3.75));
#8184=CARTESIAN_POINT('Ctrl Pts',(8.29563322262997,2.33676998946178,12.75));
#8185=CARTESIAN_POINT('Ctrl Pts',(8.24146380440172,2.33217339857873,-3.75));
#8186=CARTESIAN_POINT('Ctrl Pts',(8.24146380440172,2.33217339857873,12.75));
#8187=CARTESIAN_POINT('Ctrl Pts',(8.19867202257947,2.32567282066755,-3.75));
#8188=CARTESIAN_POINT('Ctrl Pts',(8.19867202257947,2.32567282066755,12.75));
#8189=CARTESIAN_POINT('Ctrl Pts',(8.16694940973767,2.31883955953704,-3.75));
#8190=CARTESIAN_POINT('Ctrl Pts',(8.16694940973767,2.31883955953704,12.75));
#8191=CARTESIAN_POINT('Ctrl Pts',(8.14597432907962,2.31336634706602,-3.75));
#8192=CARTESIAN_POINT('Ctrl Pts',(8.14597432907962,2.31336634706602,12.75));
#8193=CARTESIAN_POINT('Ctrl Pts',(8.13553012180811,2.31040030805735,-3.75));
#8194=CARTESIAN_POINT('Ctrl Pts',(8.13553012180811,2.31040030805735,12.75));
#8195=CARTESIAN_POINT('',(11.9792754136349,0.704954299427496,6.));
#8196=CARTESIAN_POINT('Ctrl Pts',(11.9792754136349,0.704954299427529,6.));
#8197=CARTESIAN_POINT('Ctrl Pts',(11.9691386658393,0.714023134927411,6.));
#8198=CARTESIAN_POINT('Ctrl Pts',(11.9488435391885,0.73210763976631,6.));
#8199=CARTESIAN_POINT('Ctrl Pts',(11.9183359560736,0.759074898533419,6.));
#8200=CARTESIAN_POINT('Ctrl Pts',(11.877529348846,0.794712140666325,6.));
#8201=CARTESIAN_POINT('Ctrl Pts',(11.8263046631092,0.838726039995982,6.));
#8202=CARTESIAN_POINT('Ctrl Pts',(11.7748638454684,0.882205904336896,6.));
#8203=CARTESIAN_POINT('Ctrl Pts',(11.7232078225909,0.925149766751161,6.));
#8204=CARTESIAN_POINT('Ctrl Pts',(11.6713384077523,0.967555069553193,6.));
#8205=CARTESIAN_POINT('Ctrl Pts',(11.6192586585895,1.00941863307588,6.));
#8206=CARTESIAN_POINT('Ctrl Pts',(11.5669726710206,1.05073678224334,6.));
#8207=CARTESIAN_POINT('Ctrl Pts',(11.5144851912285,1.09150552381395,6.));
#8208=CARTESIAN_POINT('Ctrl Pts',(11.4618012771636,1.13172071766774,6.));
#8209=CARTESIAN_POINT('Ctrl Pts',(11.4089259705106,1.17137823760545,6.));
#8210=CARTESIAN_POINT('Ctrl Pts',(11.3558638941869,1.21047418192819,6.));
#8211=CARTESIAN_POINT('Ctrl Pts',(11.30261917075,1.24900490126928,6.));
#8212=CARTESIAN_POINT('Ctrl Pts',(11.2491956455455,1.28696685552412,6.));
#8213=CARTESIAN_POINT('Ctrl Pts',(11.1955970312291,1.32435651843207,6.));
#8214=CARTESIAN_POINT('Ctrl Pts',(11.1418270749817,1.36117027439398,6.));
#8215=CARTESIAN_POINT('Ctrl Pts',(11.0878897426906,1.39740430473756,6.));
#8216=CARTESIAN_POINT('Ctrl Pts',(11.033789312906,1.43305454241432,6.));
#8217=CARTESIAN_POINT('Ctrl Pts',(10.9795302662584,1.46811677324654,6.));
#8218=CARTESIAN_POINT('Ctrl Pts',(10.9251172180581,1.50258671261028,6.));
#8219=CARTESIAN_POINT('Ctrl Pts',(10.8705548380775,1.53646008988796,6.));
#8220=CARTESIAN_POINT('Ctrl Pts',(10.8158477697972,1.56973274862052,6.));
#8221=CARTESIAN_POINT('Ctrl Pts',(10.761000572936,1.60240070038749,6.));
#8222=CARTESIAN_POINT('Ctrl Pts',(10.7060177866027,1.63445994423348,6.));
#8223=CARTESIAN_POINT('Ctrl Pts',(10.6509039769739,1.66590631967585,6.));
#8224=CARTESIAN_POINT('Ctrl Pts',(10.59566379085,1.69673535547184,6.));
#8225=CARTESIAN_POINT('Ctrl Pts',(10.5403020105194,1.72694211360792,6.));
#8226=CARTESIAN_POINT('Ctrl Pts',(10.4848236013528,1.75652107004318,6.));
#8227=CARTESIAN_POINT('Ctrl Pts',(10.4292336483793,1.78546643461776,6.));
#8228=CARTESIAN_POINT('Ctrl Pts',(10.3735373011506,1.81377244526718,6.));
#8229=CARTESIAN_POINT('Ctrl Pts',(10.317739716759,1.84143367405762,6.));
#8230=CARTESIAN_POINT('Ctrl Pts',(10.2618460035706,1.86844533887956,6.));
#8231=CARTESIAN_POINT('Ctrl Pts',(10.2058611678956,1.89480360265125,6.));
#8232=CARTESIAN_POINT('Ctrl Pts',(10.1497902344364,1.92050480406378,6.));
#8233=CARTESIAN_POINT('Ctrl Pts',(10.0936383641523,1.94554471072257,6.));
#8234=CARTESIAN_POINT('Ctrl Pts',(10.037410974034,1.96991776698621,6.));
#8235=CARTESIAN_POINT('Ctrl Pts',(9.98111385659409,1.99361634997092,6.));
#8236=CARTESIAN_POINT('Ctrl Pts',(9.92475330165988,2.01663001707736,6.));
#8237=CARTESIAN_POINT('Ctrl Pts',(9.86833584478527,2.03894719582859,6.));
#8238=CARTESIAN_POINT('Ctrl Pts',(9.81186801391803,2.06055689146528,6.));
#8239=CARTESIAN_POINT('Ctrl Pts',(9.75535607889871,2.08145038176732,6.));
#8240=CARTESIAN_POINT('Ctrl Pts',(9.69880579601398,2.10162295100989,6.));
#8241=CARTESIAN_POINT('Ctrl Pts',(9.64222216484242,2.12107554726937,6.));
#8242=CARTESIAN_POINT('Ctrl Pts',(9.58561005875903,2.13981058538587,6.));
#8243=CARTESIAN_POINT('Ctrl Pts',(9.52897485563506,2.15782775391113,6.));
#8244=CARTESIAN_POINT('Ctrl Pts',(9.4723230488593,2.17511995998945,6.));
#8245=CARTESIAN_POINT('Ctrl Pts',(9.41566291502215,2.19166889809876,6.));
#8246=CARTESIAN_POINT('Ctrl Pts',(9.35900502856467,2.2074416540289,6.));
#8247=CARTESIAN_POINT('Ctrl Pts',(9.30236077039477,2.22240082168223,6.));
#8248=CARTESIAN_POINT('Ctrl Pts',(9.24574089753053,2.23651421201962,6.));
#8249=CARTESIAN_POINT('Ctrl Pts',(9.18915420809356,2.24976392906278,6.));
#8250=CARTESIAN_POINT('Ctrl Pts',(9.13260588645235,2.26215759393014,6.));
#8251=CARTESIAN_POINT('Ctrl Pts',(9.07609679780011,2.27373321015996,6.));
#8252=CARTESIAN_POINT('Ctrl Pts',(9.0196273647496,2.28453333318601,6.));
#8253=CARTESIAN_POINT('Ctrl Pts',(8.96320109950669,2.29458154408801,6.));
#8254=CARTESIAN_POINT('Ctrl Pts',(8.90682777405608,2.30386137247017,6.));
#8255=CARTESIAN_POINT('Ctrl Pts',(8.85052793120604,2.31228619203479,6.));
#8256=CARTESIAN_POINT('Ctrl Pts',(8.79433301721166,2.31969862084206,6.));
#8257=CARTESIAN_POINT('Ctrl Pts',(8.73827625692193,2.32593252219559,6.));
#8258=CARTESIAN_POINT('Ctrl Pts',(8.68238458286971,2.33086762045752,6.));
#8259=CARTESIAN_POINT('Ctrl Pts',(8.62667187892838,2.33447589689188,6.));
#8260=CARTESIAN_POINT('Ctrl Pts',(8.57112741281372,2.33689888190034,6.));
#8261=CARTESIAN_POINT('Ctrl Pts',(8.51572283259063,2.33840535058003,6.));
#8262=CARTESIAN_POINT('Ctrl Pts',(8.46043689627596,2.3392342622836,6.));
#8263=CARTESIAN_POINT('Ctrl Pts',(8.40527692606173,2.339459611751,6.));
#8264=CARTESIAN_POINT('Ctrl Pts',(8.35029826768635,2.33886640526141,6.));
#8265=CARTESIAN_POINT('Ctrl Pts',(8.29563322262997,2.33676998946178,6.));
#8266=CARTESIAN_POINT('Ctrl Pts',(8.24146380440172,2.33217339857873,6.));
#8267=CARTESIAN_POINT('Ctrl Pts',(8.19867202257947,2.32567282066755,6.));
#8268=CARTESIAN_POINT('Ctrl Pts',(8.16694940973767,2.31883955953704,6.));
#8269=CARTESIAN_POINT('Ctrl Pts',(8.14597432907962,2.31336634706602,6.));
#8270=CARTESIAN_POINT('Ctrl Pts',(8.13553012180811,2.31040030805735,6.));
#8271=CARTESIAN_POINT('',(11.9792754136349,0.704954299427496,0.));
#8272=CARTESIAN_POINT('Origin',(3.99680288865056E-13,0.,0.));
#8273=CARTESIAN_POINT('',(11.9792754136349,-0.704954299427528,6.));
#8274=CARTESIAN_POINT('Origin',(3.99680288865056E-13,0.,6.));
#8275=CARTESIAN_POINT('',(11.9792754136349,-0.704954299427528,0.));
#8276=CARTESIAN_POINT('Ctrl Pts',(8.13553012180811,-2.31040030805735,-3.75));
#8277=CARTESIAN_POINT('Ctrl Pts',(8.13553012180811,-2.31040030805735,12.75));
#8278=CARTESIAN_POINT('Ctrl Pts',(8.14597432907962,-2.31336634706602,-3.75));
#8279=CARTESIAN_POINT('Ctrl Pts',(8.14597432907962,-2.31336634706602,12.75));
#8280=CARTESIAN_POINT('Ctrl Pts',(8.16694940973767,-2.31883955953704,-3.75));
#8281=CARTESIAN_POINT('Ctrl Pts',(8.16694940973767,-2.31883955953704,12.75));
#8282=CARTESIAN_POINT('Ctrl Pts',(8.19867202257947,-2.32567282066755,-3.75));
#8283=CARTESIAN_POINT('Ctrl Pts',(8.19867202257947,-2.32567282066755,12.75));
#8284=CARTESIAN_POINT('Ctrl Pts',(8.24146380440172,-2.33217339857873,-3.75));
#8285=CARTESIAN_POINT('Ctrl Pts',(8.24146380440172,-2.33217339857873,12.75));
#8286=CARTESIAN_POINT('Ctrl Pts',(8.29563322262997,-2.33676998946178,-3.75));
#8287=CARTESIAN_POINT('Ctrl Pts',(8.29563322262997,-2.33676998946178,12.75));
#8288=CARTESIAN_POINT('Ctrl Pts',(8.35029826768635,-2.33886640526141,-3.75));
#8289=CARTESIAN_POINT('Ctrl Pts',(8.35029826768635,-2.33886640526141,12.75));
#8290=CARTESIAN_POINT('Ctrl Pts',(8.40527692606173,-2.339459611751,-3.75));
#8291=CARTESIAN_POINT('Ctrl Pts',(8.40527692606173,-2.339459611751,12.75));
#8292=CARTESIAN_POINT('Ctrl Pts',(8.46043689627596,-2.3392342622836,-3.75));
#8293=CARTESIAN_POINT('Ctrl Pts',(8.46043689627596,-2.3392342622836,12.75));
#8294=CARTESIAN_POINT('Ctrl Pts',(8.51572283259063,-2.33840535058003,-3.75));
#8295=CARTESIAN_POINT('Ctrl Pts',(8.51572283259063,-2.33840535058003,12.75));
#8296=CARTESIAN_POINT('Ctrl Pts',(8.57112741281372,-2.33689888190034,-3.75));
#8297=CARTESIAN_POINT('Ctrl Pts',(8.57112741281372,-2.33689888190034,12.75));
#8298=CARTESIAN_POINT('Ctrl Pts',(8.62667187892838,-2.33447589689188,-3.75));
#8299=CARTESIAN_POINT('Ctrl Pts',(8.62667187892838,-2.33447589689188,12.75));
#8300=CARTESIAN_POINT('Ctrl Pts',(8.68238458286971,-2.33086762045752,-3.75));
#8301=CARTESIAN_POINT('Ctrl Pts',(8.68238458286971,-2.33086762045752,12.75));
#8302=CARTESIAN_POINT('Ctrl Pts',(8.73827625692193,-2.32593252219559,-3.75));
#8303=CARTESIAN_POINT('Ctrl Pts',(8.73827625692193,-2.32593252219559,12.75));
#8304=CARTESIAN_POINT('Ctrl Pts',(8.79433301721166,-2.31969862084206,-3.75));
#8305=CARTESIAN_POINT('Ctrl Pts',(8.79433301721166,-2.31969862084206,12.75));
#8306=CARTESIAN_POINT('Ctrl Pts',(8.85052793120604,-2.31228619203479,-3.75));
#8307=CARTESIAN_POINT('Ctrl Pts',(8.85052793120604,-2.31228619203479,12.75));
#8308=CARTESIAN_POINT('Ctrl Pts',(8.90682777405608,-2.30386137247017,-3.75));
#8309=CARTESIAN_POINT('Ctrl Pts',(8.90682777405608,-2.30386137247017,12.75));
#8310=CARTESIAN_POINT('Ctrl Pts',(8.96320109950669,-2.29458154408801,-3.75));
#8311=CARTESIAN_POINT('Ctrl Pts',(8.96320109950669,-2.29458154408801,12.75));
#8312=CARTESIAN_POINT('Ctrl Pts',(9.0196273647496,-2.28453333318601,-3.75));
#8313=CARTESIAN_POINT('Ctrl Pts',(9.0196273647496,-2.28453333318601,12.75));
#8314=CARTESIAN_POINT('Ctrl Pts',(9.07609679780011,-2.27373321015996,-3.75));
#8315=CARTESIAN_POINT('Ctrl Pts',(9.07609679780011,-2.27373321015996,12.75));
#8316=CARTESIAN_POINT('Ctrl Pts',(9.13260588645235,-2.26215759393014,-3.75));
#8317=CARTESIAN_POINT('Ctrl Pts',(9.13260588645235,-2.26215759393014,12.75));
#8318=CARTESIAN_POINT('Ctrl Pts',(9.18915420809356,-2.24976392906278,-3.75));
#8319=CARTESIAN_POINT('Ctrl Pts',(9.18915420809356,-2.24976392906278,12.75));
#8320=CARTESIAN_POINT('Ctrl Pts',(9.24574089753053,-2.23651421201962,-3.75));
#8321=CARTESIAN_POINT('Ctrl Pts',(9.24574089753053,-2.23651421201962,12.75));
#8322=CARTESIAN_POINT('Ctrl Pts',(9.30236077039477,-2.22240082168223,-3.75));
#8323=CARTESIAN_POINT('Ctrl Pts',(9.30236077039477,-2.22240082168223,12.75));
#8324=CARTESIAN_POINT('Ctrl Pts',(9.35900502856467,-2.2074416540289,-3.75));
#8325=CARTESIAN_POINT('Ctrl Pts',(9.35900502856467,-2.2074416540289,12.75));
#8326=CARTESIAN_POINT('Ctrl Pts',(9.41566291502215,-2.19166889809876,-3.75));
#8327=CARTESIAN_POINT('Ctrl Pts',(9.41566291502215,-2.19166889809876,12.75));
#8328=CARTESIAN_POINT('Ctrl Pts',(9.4723230488593,-2.17511995998945,-3.75));
#8329=CARTESIAN_POINT('Ctrl Pts',(9.4723230488593,-2.17511995998945,12.75));
#8330=CARTESIAN_POINT('Ctrl Pts',(9.52897485563506,-2.15782775391113,-3.75));
#8331=CARTESIAN_POINT('Ctrl Pts',(9.52897485563506,-2.15782775391113,12.75));
#8332=CARTESIAN_POINT('Ctrl Pts',(9.58561005875903,-2.13981058538587,-3.75));
#8333=CARTESIAN_POINT('Ctrl Pts',(9.58561005875903,-2.13981058538587,12.75));
#8334=CARTESIAN_POINT('Ctrl Pts',(9.64222216484242,-2.12107554726937,-3.75));
#8335=CARTESIAN_POINT('Ctrl Pts',(9.64222216484242,-2.12107554726937,12.75));
#8336=CARTESIAN_POINT('Ctrl Pts',(9.69880579601398,-2.10162295100989,-3.75));
#8337=CARTESIAN_POINT('Ctrl Pts',(9.69880579601398,-2.10162295100989,12.75));
#8338=CARTESIAN_POINT('Ctrl Pts',(9.75535607889871,-2.08145038176732,-3.75));
#8339=CARTESIAN_POINT('Ctrl Pts',(9.75535607889871,-2.08145038176732,12.75));
#8340=CARTESIAN_POINT('Ctrl Pts',(9.81186801391803,-2.06055689146528,-3.75));
#8341=CARTESIAN_POINT('Ctrl Pts',(9.81186801391803,-2.06055689146528,12.75));
#8342=CARTESIAN_POINT('Ctrl Pts',(9.86833584478527,-2.03894719582859,-3.75));
#8343=CARTESIAN_POINT('Ctrl Pts',(9.86833584478527,-2.03894719582859,12.75));
#8344=CARTESIAN_POINT('Ctrl Pts',(9.92475330165988,-2.01663001707736,-3.75));
#8345=CARTESIAN_POINT('Ctrl Pts',(9.92475330165988,-2.01663001707736,12.75));
#8346=CARTESIAN_POINT('Ctrl Pts',(9.98111385659409,-1.99361634997092,-3.75));
#8347=CARTESIAN_POINT('Ctrl Pts',(9.98111385659409,-1.99361634997092,12.75));
#8348=CARTESIAN_POINT('Ctrl Pts',(10.037410974034,-1.96991776698621,-3.75));
#8349=CARTESIAN_POINT('Ctrl Pts',(10.037410974034,-1.96991776698621,12.75));
#8350=CARTESIAN_POINT('Ctrl Pts',(10.0936383641523,-1.94554471072257,-3.75));
#8351=CARTESIAN_POINT('Ctrl Pts',(10.0936383641523,-1.94554471072257,12.75));
#8352=CARTESIAN_POINT('Ctrl Pts',(10.1497902344364,-1.92050480406378,-3.75));
#8353=CARTESIAN_POINT('Ctrl Pts',(10.1497902344364,-1.92050480406378,12.75));
#8354=CARTESIAN_POINT('Ctrl Pts',(10.2058611678956,-1.89480360265125,-3.75));
#8355=CARTESIAN_POINT('Ctrl Pts',(10.2058611678956,-1.89480360265125,12.75));
#8356=CARTESIAN_POINT('Ctrl Pts',(10.2618460035706,-1.86844533887956,-3.75));
#8357=CARTESIAN_POINT('Ctrl Pts',(10.2618460035706,-1.86844533887956,12.75));
#8358=CARTESIAN_POINT('Ctrl Pts',(10.317739716759,-1.84143367405762,-3.75));
#8359=CARTESIAN_POINT('Ctrl Pts',(10.317739716759,-1.84143367405762,12.75));
#8360=CARTESIAN_POINT('Ctrl Pts',(10.3735373011506,-1.81377244526718,-3.75));
#8361=CARTESIAN_POINT('Ctrl Pts',(10.3735373011506,-1.81377244526718,12.75));
#8362=CARTESIAN_POINT('Ctrl Pts',(10.4292336483793,-1.78546643461776,-3.75));
#8363=CARTESIAN_POINT('Ctrl Pts',(10.4292336483793,-1.78546643461776,12.75));
#8364=CARTESIAN_POINT('Ctrl Pts',(10.4848236013528,-1.75652107004318,-3.75));
#8365=CARTESIAN_POINT('Ctrl Pts',(10.4848236013528,-1.75652107004318,12.75));
#8366=CARTESIAN_POINT('Ctrl Pts',(10.5403020105194,-1.72694211360792,-3.75));
#8367=CARTESIAN_POINT('Ctrl Pts',(10.5403020105194,-1.72694211360792,12.75));
#8368=CARTESIAN_POINT('Ctrl Pts',(10.59566379085,-1.69673535547184,-3.75));
#8369=CARTESIAN_POINT('Ctrl Pts',(10.59566379085,-1.69673535547184,12.75));
#8370=CARTESIAN_POINT('Ctrl Pts',(10.6509039769739,-1.66590631967585,-3.75));
#8371=CARTESIAN_POINT('Ctrl Pts',(10.6509039769739,-1.66590631967585,12.75));
#8372=CARTESIAN_POINT('Ctrl Pts',(10.7060177866027,-1.63445994423348,-3.75));
#8373=CARTESIAN_POINT('Ctrl Pts',(10.7060177866027,-1.63445994423348,12.75));
#8374=CARTESIAN_POINT('Ctrl Pts',(10.761000572936,-1.60240070038749,-3.75));
#8375=CARTESIAN_POINT('Ctrl Pts',(10.761000572936,-1.60240070038749,12.75));
#8376=CARTESIAN_POINT('Ctrl Pts',(10.8158477697972,-1.56973274862052,-3.75));
#8377=CARTESIAN_POINT('Ctrl Pts',(10.8158477697972,-1.56973274862052,12.75));
#8378=CARTESIAN_POINT('Ctrl Pts',(10.8705548380775,-1.53646008988796,-3.75));
#8379=CARTESIAN_POINT('Ctrl Pts',(10.8705548380775,-1.53646008988796,12.75));
#8380=CARTESIAN_POINT('Ctrl Pts',(10.9251172180581,-1.50258671261028,-3.75));
#8381=CARTESIAN_POINT('Ctrl Pts',(10.9251172180581,-1.50258671261028,12.75));
#8382=CARTESIAN_POINT('Ctrl Pts',(10.9795302662584,-1.46811677324654,-3.75));
#8383=CARTESIAN_POINT('Ctrl Pts',(10.9795302662584,-1.46811677324654,12.75));
#8384=CARTESIAN_POINT('Ctrl Pts',(11.033789312906,-1.43305454241432,-3.75));
#8385=CARTESIAN_POINT('Ctrl Pts',(11.033789312906,-1.43305454241432,12.75));
#8386=CARTESIAN_POINT('Ctrl Pts',(11.0878897426906,-1.39740430473756,-3.75));
#8387=CARTESIAN_POINT('Ctrl Pts',(11.0878897426906,-1.39740430473756,12.75));
#8388=CARTESIAN_POINT('Ctrl Pts',(11.1418270749817,-1.36117027439398,-3.75));
#8389=CARTESIAN_POINT('Ctrl Pts',(11.1418270749817,-1.36117027439398,12.75));
#8390=CARTESIAN_POINT('Ctrl Pts',(11.1955970312291,-1.32435651843207,-3.75));
#8391=CARTESIAN_POINT('Ctrl Pts',(11.1955970312291,-1.32435651843207,12.75));
#8392=CARTESIAN_POINT('Ctrl Pts',(11.2491956455455,-1.28696685552412,-3.75));
#8393=CARTESIAN_POINT('Ctrl Pts',(11.2491956455455,-1.28696685552412,12.75));
#8394=CARTESIAN_POINT('Ctrl Pts',(11.30261917075,-1.24900490126928,-3.75));
#8395=CARTESIAN_POINT('Ctrl Pts',(11.30261917075,-1.24900490126928,12.75));
#8396=CARTESIAN_POINT('Ctrl Pts',(11.3558638941869,-1.21047418192819,-3.75));
#8397=CARTESIAN_POINT('Ctrl Pts',(11.3558638941869,-1.21047418192819,12.75));
#8398=CARTESIAN_POINT('Ctrl Pts',(11.4089259705106,-1.17137823760545,-3.75));
#8399=CARTESIAN_POINT('Ctrl Pts',(11.4089259705106,-1.17137823760545,12.75));
#8400=CARTESIAN_POINT('Ctrl Pts',(11.4618012771636,-1.13172071766774,-3.75));
#8401=CARTESIAN_POINT('Ctrl Pts',(11.4618012771636,-1.13172071766774,12.75));
#8402=CARTESIAN_POINT('Ctrl Pts',(11.5144851912285,-1.09150552381395,-3.75));
#8403=CARTESIAN_POINT('Ctrl Pts',(11.5144851912285,-1.09150552381395,12.75));
#8404=CARTESIAN_POINT('Ctrl Pts',(11.5669726710206,-1.05073678224334,-3.75));
#8405=CARTESIAN_POINT('Ctrl Pts',(11.5669726710206,-1.05073678224334,12.75));
#8406=CARTESIAN_POINT('Ctrl Pts',(11.6192586585895,-1.00941863307588,-3.75));
#8407=CARTESIAN_POINT('Ctrl Pts',(11.6192586585895,-1.00941863307588,12.75));
#8408=CARTESIAN_POINT('Ctrl Pts',(11.6713384077523,-0.967555069553193,-3.75));
#8409=CARTESIAN_POINT('Ctrl Pts',(11.6713384077523,-0.967555069553193,12.75));
#8410=CARTESIAN_POINT('Ctrl Pts',(11.7232078225909,-0.925149766751161,-3.75));
#8411=CARTESIAN_POINT('Ctrl Pts',(11.7232078225909,-0.925149766751161,12.75));
#8412=CARTESIAN_POINT('Ctrl Pts',(11.7748638454684,-0.882205904336896,-3.75));
#8413=CARTESIAN_POINT('Ctrl Pts',(11.7748638454684,-0.882205904336896,12.75));
#8414=CARTESIAN_POINT('Ctrl Pts',(11.8263046631092,-0.838726039995982,-3.75));
#8415=CARTESIAN_POINT('Ctrl Pts',(11.8263046631092,-0.838726039995982,12.75));
#8416=CARTESIAN_POINT('Ctrl Pts',(11.877529348846,-0.794712140666325,-3.75));
#8417=CARTESIAN_POINT('Ctrl Pts',(11.877529348846,-0.794712140666325,12.75));
#8418=CARTESIAN_POINT('Ctrl Pts',(11.9183359560736,-0.759074898533419,-3.75));
#8419=CARTESIAN_POINT('Ctrl Pts',(11.9183359560736,-0.759074898533419,12.75));
#8420=CARTESIAN_POINT('Ctrl Pts',(11.9488435391885,-0.73210763976631,-3.75));
#8421=CARTESIAN_POINT('Ctrl Pts',(11.9488435391885,-0.73210763976631,12.75));
#8422=CARTESIAN_POINT('Ctrl Pts',(11.9691386658393,-0.714023134927411,-3.75));
#8423=CARTESIAN_POINT('Ctrl Pts',(11.9691386658393,-0.714023134927411,12.75));
#8424=CARTESIAN_POINT('Ctrl Pts',(11.9792754136349,-0.704954299427529,-3.75));
#8425=CARTESIAN_POINT('Ctrl Pts',(11.9792754136349,-0.704954299427529,12.75));
#8426=CARTESIAN_POINT('Ctrl Pts',(8.13553012180811,-2.31040030805735,6.));
#8427=CARTESIAN_POINT('Ctrl Pts',(8.14597432907962,-2.31336634706602,6.));
#8428=CARTESIAN_POINT('Ctrl Pts',(8.16694940973767,-2.31883955953704,6.));
#8429=CARTESIAN_POINT('Ctrl Pts',(8.19867202257947,-2.32567282066755,6.));
#8430=CARTESIAN_POINT('Ctrl Pts',(8.24146380440172,-2.33217339857873,6.));
#8431=CARTESIAN_POINT('Ctrl Pts',(8.29563322262997,-2.33676998946178,6.));
#8432=CARTESIAN_POINT('Ctrl Pts',(8.35029826768635,-2.33886640526141,6.));
#8433=CARTESIAN_POINT('Ctrl Pts',(8.40527692606173,-2.339459611751,6.));
#8434=CARTESIAN_POINT('Ctrl Pts',(8.46043689627596,-2.3392342622836,6.));
#8435=CARTESIAN_POINT('Ctrl Pts',(8.51572283259063,-2.33840535058003,6.));
#8436=CARTESIAN_POINT('Ctrl Pts',(8.57112741281372,-2.33689888190034,6.));
#8437=CARTESIAN_POINT('Ctrl Pts',(8.62667187892838,-2.33447589689188,6.));
#8438=CARTESIAN_POINT('Ctrl Pts',(8.68238458286971,-2.33086762045752,6.));
#8439=CARTESIAN_POINT('Ctrl Pts',(8.73827625692193,-2.32593252219559,6.));
#8440=CARTESIAN_POINT('Ctrl Pts',(8.79433301721166,-2.31969862084206,6.));
#8441=CARTESIAN_POINT('Ctrl Pts',(8.85052793120604,-2.31228619203479,6.));
#8442=CARTESIAN_POINT('Ctrl Pts',(8.90682777405608,-2.30386137247017,6.));
#8443=CARTESIAN_POINT('Ctrl Pts',(8.96320109950669,-2.29458154408801,6.));
#8444=CARTESIAN_POINT('Ctrl Pts',(9.0196273647496,-2.28453333318601,6.));
#8445=CARTESIAN_POINT('Ctrl Pts',(9.07609679780011,-2.27373321015996,6.));
#8446=CARTESIAN_POINT('Ctrl Pts',(9.13260588645235,-2.26215759393014,6.));
#8447=CARTESIAN_POINT('Ctrl Pts',(9.18915420809356,-2.24976392906278,6.));
#8448=CARTESIAN_POINT('Ctrl Pts',(9.24574089753053,-2.23651421201962,6.));
#8449=CARTESIAN_POINT('Ctrl Pts',(9.30236077039477,-2.22240082168223,6.));
#8450=CARTESIAN_POINT('Ctrl Pts',(9.35900502856467,-2.2074416540289,6.));
#8451=CARTESIAN_POINT('Ctrl Pts',(9.41566291502215,-2.19166889809876,6.));
#8452=CARTESIAN_POINT('Ctrl Pts',(9.4723230488593,-2.17511995998945,6.));
#8453=CARTESIAN_POINT('Ctrl Pts',(9.52897485563506,-2.15782775391113,6.));
#8454=CARTESIAN_POINT('Ctrl Pts',(9.58561005875903,-2.13981058538587,6.));
#8455=CARTESIAN_POINT('Ctrl Pts',(9.64222216484242,-2.12107554726937,6.));
#8456=CARTESIAN_POINT('Ctrl Pts',(9.69880579601398,-2.10162295100989,6.));
#8457=CARTESIAN_POINT('Ctrl Pts',(9.75535607889871,-2.08145038176732,6.));
#8458=CARTESIAN_POINT('Ctrl Pts',(9.81186801391803,-2.06055689146528,6.));
#8459=CARTESIAN_POINT('Ctrl Pts',(9.86833584478527,-2.03894719582859,6.));
#8460=CARTESIAN_POINT('Ctrl Pts',(9.92475330165988,-2.01663001707736,6.));
#8461=CARTESIAN_POINT('Ctrl Pts',(9.98111385659409,-1.99361634997092,6.));
#8462=CARTESIAN_POINT('Ctrl Pts',(10.037410974034,-1.96991776698621,6.));
#8463=CARTESIAN_POINT('Ctrl Pts',(10.0936383641523,-1.94554471072257,6.));
#8464=CARTESIAN_POINT('Ctrl Pts',(10.1497902344364,-1.92050480406378,6.));
#8465=CARTESIAN_POINT('Ctrl Pts',(10.2058611678956,-1.89480360265125,6.));
#8466=CARTESIAN_POINT('Ctrl Pts',(10.2618460035706,-1.86844533887956,6.));
#8467=CARTESIAN_POINT('Ctrl Pts',(10.317739716759,-1.84143367405762,6.));
#8468=CARTESIAN_POINT('Ctrl Pts',(10.3735373011506,-1.81377244526718,6.));
#8469=CARTESIAN_POINT('Ctrl Pts',(10.4292336483793,-1.78546643461776,6.));
#8470=CARTESIAN_POINT('Ctrl Pts',(10.4848236013528,-1.75652107004318,6.));
#8471=CARTESIAN_POINT('Ctrl Pts',(10.5403020105194,-1.72694211360792,6.));
#8472=CARTESIAN_POINT('Ctrl Pts',(10.59566379085,-1.69673535547184,6.));
#8473=CARTESIAN_POINT('Ctrl Pts',(10.6509039769739,-1.66590631967585,6.));
#8474=CARTESIAN_POINT('Ctrl Pts',(10.7060177866027,-1.63445994423348,6.));
#8475=CARTESIAN_POINT('Ctrl Pts',(10.761000572936,-1.60240070038749,6.));
#8476=CARTESIAN_POINT('Ctrl Pts',(10.8158477697972,-1.56973274862052,6.));
#8477=CARTESIAN_POINT('Ctrl Pts',(10.8705548380775,-1.53646008988796,6.));
#8478=CARTESIAN_POINT('Ctrl Pts',(10.9251172180581,-1.50258671261028,6.));
#8479=CARTESIAN_POINT('Ctrl Pts',(10.9795302662584,-1.46811677324654,6.));
#8480=CARTESIAN_POINT('Ctrl Pts',(11.033789312906,-1.43305454241432,6.));
#8481=CARTESIAN_POINT('Ctrl Pts',(11.0878897426906,-1.39740430473756,6.));
#8482=CARTESIAN_POINT('Ctrl Pts',(11.1418270749817,-1.36117027439398,6.));
#8483=CARTESIAN_POINT('Ctrl Pts',(11.1955970312291,-1.32435651843207,6.));
#8484=CARTESIAN_POINT('Ctrl Pts',(11.2491956455455,-1.28696685552412,6.));
#8485=CARTESIAN_POINT('Ctrl Pts',(11.30261917075,-1.24900490126928,6.));
#8486=CARTESIAN_POINT('Ctrl Pts',(11.3558638941869,-1.21047418192819,6.));
#8487=CARTESIAN_POINT('Ctrl Pts',(11.4089259705106,-1.17137823760545,6.));
#8488=CARTESIAN_POINT('Ctrl Pts',(11.4618012771636,-1.13172071766774,6.));
#8489=CARTESIAN_POINT('Ctrl Pts',(11.5144851912285,-1.09150552381395,6.));
#8490=CARTESIAN_POINT('Ctrl Pts',(11.5669726710206,-1.05073678224334,6.));
#8491=CARTESIAN_POINT('Ctrl Pts',(11.6192586585895,-1.00941863307588,6.));
#8492=CARTESIAN_POINT('Ctrl Pts',(11.6713384077523,-0.967555069553193,6.));
#8493=CARTESIAN_POINT('Ctrl Pts',(11.7232078225909,-0.925149766751161,6.));
#8494=CARTESIAN_POINT('Ctrl Pts',(11.7748638454684,-0.882205904336896,6.));
#8495=CARTESIAN_POINT('Ctrl Pts',(11.8263046631092,-0.838726039995982,6.));
#8496=CARTESIAN_POINT('Ctrl Pts',(11.877529348846,-0.794712140666325,6.));
#8497=CARTESIAN_POINT('Ctrl Pts',(11.9183359560736,-0.759074898533419,6.));
#8498=CARTESIAN_POINT('Ctrl Pts',(11.9488435391885,-0.73210763976631,6.));
#8499=CARTESIAN_POINT('Ctrl Pts',(11.9691386658393,-0.714023134927411,6.));
#8500=CARTESIAN_POINT('Ctrl Pts',(11.9792754136349,-0.704954299427529,6.));
#8501=CARTESIAN_POINT('Origin',(0.,0.,6.));
#8502=CARTESIAN_POINT('Origin',(0.,0.,6.));
#8503=CARTESIAN_POINT('',(-5.,6.12323399573677E-16,6.));
#8504=CARTESIAN_POINT('Origin',(0.,0.,6.));
#8505=CARTESIAN_POINT('Origin',(0.,0.,0.));
#8506=CARTESIAN_POINT('',(-5.,-6.12323399573677E-16,0.));
#8507=CARTESIAN_POINT('Origin',(0.,0.,0.));
#9802=UNCERTAINTY_MEASURE_WITH_UNIT(LENGTH_MEASURE(0.01),#9823,
'DISTANCE_ACCURACY_VALUE',
'Maximum model space distance between geometric entities at asserted c
onnectivities');
#9811=UNCERTAINTY_MEASURE_WITH_UNIT(LENGTH_MEASURE(0.01),#9823,
'DISTANCE_ACCURACY_VALUE',
'Maximum model space distance between geometric entities at asserted c
onnectivities');
#9813=(
GEOMETRIC_REPRESENTATION_CONTEXT(3)
GLOBAL_UNCERTAINTY_ASSIGNED_CONTEXT((#9802))
GLOBAL_UNIT_ASSIGNED_CONTEXT((#9823,#9825,#9826))
REPRESENTATION_CONTEXT('','3D')
);
#9822=(
GEOMETRIC_REPRESENTATION_CONTEXT(3)
GLOBAL_UNCERTAINTY_ASSIGNED_CONTEXT((#9811))
GLOBAL_UNIT_ASSIGNED_CONTEXT((#9823,#9825,#9826))
REPRESENTATION_CONTEXT('','3D')
);
#9823=(
LENGTH_UNIT()
NAMED_UNIT(*)
SI_UNIT(.MILLI.,.METRE.)
);
#9825=(
NAMED_UNIT(*)
PLANE_ANGLE_UNIT()
SI_UNIT($,.RADIAN.)
);
#9826=(
NAMED_UNIT(*)
SI_UNIT($,.STERADIAN.)
SOLID_ANGLE_UNIT()
);
#9828=SHAPE_DEFINITION_REPRESENTATION(#9838,#9857);
#9838=PRODUCT_DEFINITION_SHAPE('',$,#9868);
#9857=SHAPE_REPRESENTATION('',(#3398),#9813);
#9866=PRODUCT_DEFINITION_CONTEXT('part definition',#9898,'design');
#9868=PRODUCT_DEFINITION('Spider','Spider',#9878,#9866);
#9878=PRODUCT_DEFINITION_FORMATION('',$,#9901);
#9898=APPLICATION_CONTEXT(
'Core Data for Automotive Mechanical Design Process');
#9899=PRODUCT_CONTEXT('part definition',#9898,'mechanical');
#9901=PRODUCT('Spider','Spider',
'Spur Gear; Module: 3.0; Num Teeth: 6; Pressure Angle: 20.0; Backlash:
 0.00 mm',(#9899));
#9911=PRESENTATION_STYLE_ASSIGNMENT((#9914));
#9914=SURFACE_STYLE_USAGE(.BOTH.,#9917);
#9917=SURFACE_SIDE_STYLE('',(#9920));
#9920=SURFACE_STYLE_FILL_AREA(#9923);
#9923=FILL_AREA_STYLE('Opaque(78,78,78)',(#9926));
#9926=FILL_AREA_STYLE_COLOUR('Opaque(78,78,78)',#9929);
#9929=COLOUR_RGB('Opaque(78,78,78)', 0.09019608, 0.27058824, 0.51372549);
ENDSEC;
END-ISO-10303-21;
